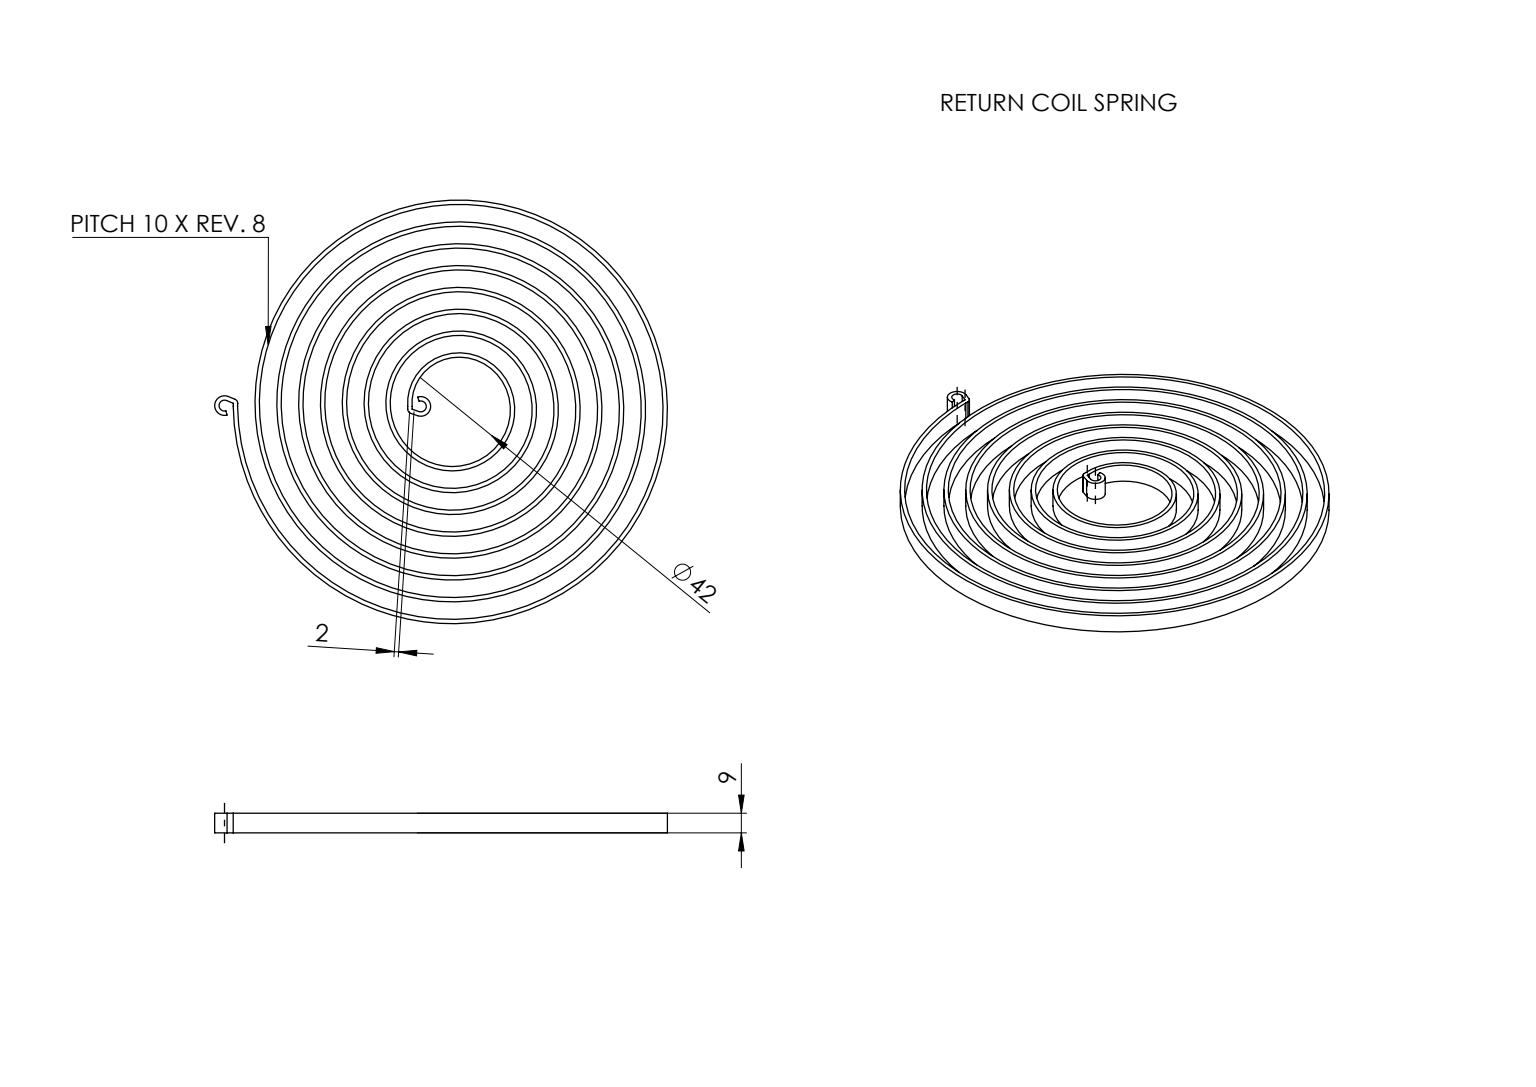
ISO-10303-21;
HEADER;
FILE_DESCRIPTION (('STEP AP214'),
    '1' );
FILE_NAME ('Return Coil Spring.step',
    '2026-10-08T11:45:07',
    ( '' ),
    ( '' ),
    'SwSTEP 2.0',
    'SolidWorks 2026',
    '' );
FILE_SCHEMA (( 'AUTOMOTIVE_DESIGN' ));
ENDSEC;

DATA;
#8=CARTESIAN_POINT ( 'NONE',  ( -38.31599561464027914, 40.00000000000000000, 10.26995502114586678 ) ) ;
#9=CARTESIAN_POINT ( 'NONE',  ( -48.87578956996785706, 40.00000000000000000, 16.50293044077288940 ) ) ;
#19=CARTESIAN_POINT ( 'NONE',  ( -15.99999999999997691, 17.11489954122026447, -2.499999999999994671 ) ) ;
#36=CARTESIAN_POINT ( 'NONE',  ( -50.06114249714176623, 31.00000000000000355, -38.53249520213265811 ) ) ;
#44=CARTESIAN_POINT ( 'NONE',  ( 25.34170449640226508, 40.00000000000000000, 74.97748276543396173 ) ) ;
#56=CARTESIAN_POINT ( 'NONE',  ( 73.00591898829820536, 31.00000000000000000, 19.54754034098114701 ) ) ;
#81=DIRECTION ( 'NONE',  ( 0.000000000000000000, 1.000000000000000000, -1.060184893785364939E-15 ) ) ;
#85=CARTESIAN_POINT ( 'NONE',  ( 15.66220904948440662, 31.00000000000000355, -31.63873590539992264 ) ) ;
#94=CARTESIAN_POINT ( 'NONE',  ( 55.55275676651330485, 40.00000000000000000, 14.97830846782891712 ) ) ;
#109=CARTESIAN_POINT ( 'NONE',  ( 33.03432996520027132, 31.00000000000000355, -28.98482729919588863 ) ) ;
#116=CARTESIAN_POINT ( 'NONE',  ( -78.67873774631718220, 31.00000000000000711, 60.36924185307643143 ) ) ;
#119=CARTESIAN_POINT ( 'NONE',  ( -67.85934734803990409, 31.00000000000000711, 22.92939687791763248 ) ) ;
#120=CARTESIAN_POINT ( 'NONE',  ( 33.43413415811954792, 40.00000000000000000, -67.56680175473154293 ) ) ;
#139=CARTESIAN_POINT ( 'NONE',  ( -5.399612364985466151, 40.00000000000000000, -82.39583333413678190 ) ) ;
#157=ADVANCED_FACE ( 'NONE', ( #19485 ), #6553, .F. ) ;
#159=( LENGTH_UNIT ( ) NAMED_UNIT ( * ) SI_UNIT ( .MILLI., .METRE. ) );
#168=CARTESIAN_POINT ( 'NONE',  ( -23.19911330973958030, 31.00000000000000355, -68.30030121463531145 ) ) ;
#171=CARTESIAN_POINT ( 'NONE',  ( 32.80084743084299248, 31.00000000000000355, 19.01436317119123842 ) ) ;
#172=CARTESIAN_POINT ( 'NONE',  ( -21.28946418274055929, 40.00000000000000000, -79.45670318283352174 ) ) ;
#183=CARTESIAN_POINT ( 'NONE',  ( 50.09382087749727930, 40.00000000000000000, 24.69014870349942825 ) ) ;
#197=CARTESIAN_POINT ( 'NONE',  ( 96.56285295106283684, 31.00000000000000000, 12.84127866191736977 ) ) ;
#213=CARTESIAN_POINT ( 'NONE',  ( -25.29482881991252086, 31.00000000000000355, -32.96004927633274662 ) ) ;
#219=CARTESIAN_POINT ( 'NONE',  ( 32.11716166826300167, 40.00000000000000000, 15.82712457579038912 ) ) ;
#221=CARTESIAN_POINT ( 'NONE',  ( 42.86166521172830102, 40.00000000000000000, 21.22462828019262204 ) ) ;
#230=CARTESIAN_POINT ( 'NONE',  ( 7.028922914820973311, 40.00000000000000000, 26.21578750688660264 ) ) ;
#237=VECTOR ( 'NONE', #15107, 1000.000000000000000 ) ;
#249=CARTESIAN_POINT ( 'NONE',  ( -20.51812799676685373, 31.00000000000000355, -60.74091093256831897 ) ) ;
#257=CARTESIAN_POINT ( 'NONE',  ( -10.54315780146311532, 40.00000000000000000, 79.17709703063971460 ) ) ;
#270=CARTESIAN_POINT ( 'NONE',  ( -45.94448050778635917, 31.00000000000000355, -79.54744219826071117 ) ) ;
#292=ORIENTED_EDGE ( 'NONE', *, *, #9832, .T. ) ;
#302=CARTESIAN_POINT ( 'NONE',  ( -29.39530816626169241, 31.00000000000000355, -14.54745122861254814 ) ) ;
#314=CARTESIAN_POINT ( 'NONE',  ( -17.30549157494238344, 40.00000000000000000, -51.24895740946764988 ) ) ;
#324=CARTESIAN_POINT ( 'NONE',  ( -105.9879088449591933, 17.11489954122026447, -4.880719929157669945 ) ) ;
#325=CARTESIAN_POINT ( 'NONE',  ( 3.108867721649529958, 31.00000000000000355, 47.39583333474234905 ) ) ;
#333=CARTESIAN_POINT ( 'NONE',  ( -20.64238946400878305, 31.00000000000000355, 3.177240882809045708 ) ) ;
#335=CARTESIAN_POINT ( 'NONE',  ( 58.84426737335365232, 31.00000000000000355, 76.69096868241209108 ) ) ;
#340=CARTESIAN_POINT ( 'NONE',  ( -25.88810397299713628, 31.00000000000000355, 75.89534075019484760 ) ) ;
#341=CARTESIAN_POINT ( 'NONE',  ( -79.00001692107187523, 40.00000000000000711, 21.04436337234429999 ) ) ;
#346=ORIENTED_EDGE ( 'NONE', *, *, #31412, .T. ) ;
#357=CARTESIAN_POINT ( 'NONE',  ( 36.87680687886029318, 40.00000000000000000, -74.81172728975037955 ) ) ;
#386=CARTESIAN_POINT ( 'NONE',  ( -20.07939870814534089, 31.00000000000000355, -2.638545259751242877 ) ) ;
#390=ADVANCED_FACE ( 'NONE', ( #24276 ), #4353, .F. ) ;
#393=CARTESIAN_POINT ( 'NONE',  ( -9.469526743414824921, 31.00000000000000355, -71.82433816204535049 ) ) ;
#396=CARTESIAN_POINT ( 'NONE',  ( 31.88898475263450649, 31.00000000000000355, 36.48290236124523744 ) ) ;
#397=CARTESIAN_POINT ( 'NONE',  ( 63.16980243745005907, 39.99999999999999289, -55.41789732285823078 ) ) ;
#413=CARTESIAN_POINT ( 'NONE',  ( 51.69409438402072965, 40.00000000000000000, -17.56033928829605273 ) ) ;
#426=CARTESIAN_POINT ( 'NONE',  ( -73.90312034494817794, 31.00000000000000711, -56.84521418461152109 ) ) ;
#440=CARTESIAN_POINT ( 'NONE',  ( -101.9145453900124068, 31.00000000000000355, -1.407535261550473704 ) ) ;
#448=AXIS2_PLACEMENT_3D ( 'NONE', #41556, #21331, #31328 ) ;
#450=CARTESIAN_POINT ( 'NONE',  ( -39.89583333501392559, 31.00000000000000355, 2.617993869485681468 ) ) ;
#457=CARTESIAN_POINT ( 'NONE',  ( -16.75480014238754478, 40.00000000000000000, -49.32177912249007790 ) ) ;
#458=CARTESIAN_POINT ( 'NONE',  ( -37.13421060599359436, 40.00000000000000000, -21.52932707635456211 ) ) ;
#466=CARTESIAN_POINT ( 'NONE',  ( -12.50349052776452297, 40.00000000000000000, 25.37591446456323041 ) ) ;
#468=DIRECTION ( 'NONE',  ( 0.000000000000000000, 1.000000000000000000, 0.000000000000000000 ) ) ;
#484=CARTESIAN_POINT ( 'NONE',  ( -59.63693792270941429, 31.00000000000000711, 15.87187584493272929 ) ) ;
#488=FACE_OUTER_BOUND ( 'NONE', #34162, .T. ) ;
#491=CARTESIAN_POINT ( 'NONE',  ( -82.09281090897877675, 40.00000000000000711, -5.486092462564050365 ) ) ;
#511=CARTESIAN_POINT ( 'NONE',  ( -60.37409795221152109, 31.00000000000000711, -68.82020352599361956 ) ) ;
#517=EDGE_CURVE ( 'NONE', #5078, #15357, #24037, .T. ) ;
#541=CARTESIAN_POINT ( 'NONE',  ( 2.319640971205256363, 31.00000000000000355, -34.59922639972668179 ) ) ;
#548=CARTESIAN_POINT ( 'NONE',  ( -6.590854309045714565, 40.00000000000000000, 49.37518673228670707 ) ) ;
#558=CARTESIAN_POINT ( 'NONE',  ( 40.56819808336118882, 31.00000000000000355, -35.59309480518532354 ) ) ;
#567=CARTESIAN_POINT ( 'NONE',  ( 5.935205493550105516, 40.00000000000000000, -22.18504493031268865 ) ) ;
#573=CARTESIAN_POINT ( 'NONE',  ( 61.98103557012429121, 31.00000000000000000, 47.69015029125303329 ) ) ;
#574=CARTESIAN_POINT ( 'NONE',  ( 73.52353481979008620, 39.99999999999999289, 25.08131146963209090 ) ) ;
#586=CARTESIAN_POINT ( 'NONE',  ( 84.89583333414414312, 39.99999999999999289, -5.563236982362012029 ) ) ;
#589=ORIENTED_EDGE ( 'NONE', *, *, #18866, .T. ) ;
#591=CARTESIAN_POINT ( 'NONE',  ( -105.9879088449591933, 31.00000000000000355, -0.3807199291576673361 ) ) ;
#600=DIRECTION ( 'NONE',  ( 0.000000000000000000, 1.000000000000000000, -1.060184893785364939E-15 ) ) ;
#608=CARTESIAN_POINT ( 'NONE',  ( -10.31048697494744815, 31.00000000000000355, -30.34325702988586215 ) ) ;
#614=CARTESIAN_POINT ( 'NONE',  ( -68.16583574478268304, 31.00000000000000711, -18.25112749842637427 ) ) ;
#617=CARTESIAN_POINT ( 'NONE',  ( -13.02511903071888355, 31.00000000000000355, 48.29538318457647961 ) ) ;
#618=CARTESIAN_POINT ( 'NONE',  ( -79.89583333417640176, 40.00000000000000711, 5.235987747608064957 ) ) ;
#627=CARTESIAN_POINT ( 'NONE',  ( 35.44578089419255917, 40.00000000000000000, -40.42088417236866604 ) ) ;
#644=VECTOR ( 'NONE', #35434, 1000.000000000000000 ) ;
#659=CARTESIAN_POINT ( 'NONE',  ( -19.20510714644778361, 31.00000000000000355, 33.27066566623395261 ) ) ;
#666=CARTESIAN_POINT ( 'NONE',  ( -29.60425243605831724, 40.00000000000000000, 38.59963703562669934 ) ) ;
#667=CARTESIAN_POINT ( 'NONE',  ( 40.10317558969867946, 40.00000000000000000, -23.06553963618951286 ) ) ;
#677=CARTESIAN_POINT ( 'NONE',  ( 15.62097837807030842, 40.00000000000000000, -17.81927981957692353 ) ) ;
#695=CARTESIAN_POINT ( 'NONE',  ( 4.437437895627577511, 31.00000000000000355, 69.40004907510417809 ) ) ;
#702=CARTESIAN_POINT ( 'NONE',  ( -6.060882879309179572, 40.00000000000000000, -94.40013096063921694 ) ) ;
#707=DIRECTION ( 'NONE',  ( 0.000000000000000000, 0.000000000000000000, -1.000000000000000000 ) ) ;
#716=CARTESIAN_POINT ( 'NONE',  ( -72.39171112334068425, 31.00000000000000711, -55.52881859171880308 ) ) ;
#733=DIRECTION ( 'NONE',  ( -0.9470131699890044219, 0.000000000000000000, 0.3211947320043981868 ) ) ;
#745=VECTOR ( 'NONE', #33359, 1000.000000000000000 ) ;
#749=CARTESIAN_POINT ( 'NONE',  ( -8.786317949316114095, 31.00000000000000355, -33.00646673688142840 ) ) ;
#757=CARTESIAN_POINT ( 'NONE',  ( 15.22596115864829969, 40.00000000000000000, 57.21640888977480444 ) ) ;
#771=CARTESIAN_POINT ( 'NONE',  ( 52.68777711438346500, 31.00000000000000355, 17.88338314711659294 ) ) ;
#776=CARTESIAN_POINT ( 'NONE',  ( -16.73417733071809721, 40.00000000000000000, -12.82953315787133519 ) ) ;
#781=CARTESIAN_POINT ( 'NONE',  ( 68.60033760563639760, 31.00000000000000000, -33.70054013428169526 ) ) ;
#782=CARTESIAN_POINT ( 'NONE',  ( 57.21690105882998267, 39.99999999999999289, -50.04162206025958426 ) ) ;
#796=CARTESIAN_POINT ( 'NONE',  ( 21.49215960483416410, 40.00000000000000000, -80.26604385357094884 ) ) ;
#820=CARTESIAN_POINT ( 'NONE',  ( -24.68525358734468611, 31.00000000000000355, -18.92943107747915832 ) ) ;
#827=CARTESIAN_POINT ( 'NONE',  ( -61.47519263390311295, 31.00000000000000711, -35.49250405583519807 ) ) ;
#832=CARTESIAN_POINT ( 'NONE',  ( 22.78600399167716262, 31.00000000000000355, -39.30137845375363526 ) ) ;
#834=CARTESIAN_POINT ( 'NONE',  ( -68.69954721042445556, 40.00000000000000711, 39.68009708086182741 ) ) ;
#845=CARTESIAN_POINT ( 'NONE',  ( -47.94314659152439617, 40.00000000000000000, -16.27230485535717719 ) ) ;
#858=CARTESIAN_POINT ( 'NONE',  ( -96.33078216555148288, 31.00000000000000711, 32.58251675337926656 ) ) ;
#859=ADVANCED_FACE ( 'NONE', ( #7595 ), #30942, .T. ) ;
#873=CARTESIAN_POINT ( 'NONE',  ( 21.71086051706764763, 31.00000000000000355, -37.60982366119799991 ) ) ;
#882=CARTESIAN_POINT ( 'NONE',  ( 6.197074855318628117, 40.00000000000000000, 46.98549035852928313 ) ) ;
#883=CARTESIAN_POINT ( 'NONE',  ( 56.43498182459031653, 40.00000000000000000, -7.339809665447900144 ) ) ;
#893=CARTESIAN_POINT ( 'NONE',  ( 24.60508655230852781, 40.00000000000000000, 6.583411914924224284 ) ) ;
#907=CARTESIAN_POINT ( 'NONE',  ( 58.79931003850258975, 31.00000000000000355, 51.72161244499935151 ) ) ;
#908=ADVANCED_FACE ( 'NONE', ( #10220 ), #3863, .T. ) ;
#916=CARTESIAN_POINT ( 'NONE',  ( 63.29164158768324455, 39.99999999999999289, -71.97807289018581400 ) ) ;
#927=CARTESIAN_POINT ( 'NONE',  ( -39.09256291070916944, 31.00000000000000355, 79.30589209199378331 ) ) ;
#934=CARTESIAN_POINT ( 'NONE',  ( -15.43003214871520434, 40.00000000000000000, -17.59684744742188300 ) ) ;
#954=CARTESIAN_POINT ( 'NONE',  ( 25.04716826810500763, 31.00000000000000355, 3.293035637142270655 ) ) ;
#962=CARTESIAN_POINT ( 'NONE',  ( -19.32876798325804302, 31.00000000000000355, -39.37500834189552279 ) ) ;
#969=CARTESIAN_POINT ( 'NONE',  ( 60.82800096160986669, 39.99999999999999289, 30.10617641797072963 ) ) ;
#981=CARTESIAN_POINT ( 'NONE',  ( 54.89583333452979730, 31.00000000000000355, -3.599741573803383332 ) ) ;
#991=CARTESIAN_POINT ( 'NONE',  ( -4.233603722440171246, 40.00000000000000000, -32.08218167604271542 ) ) ;
#995=CARTESIAN_POINT ( 'NONE',  ( 72.60479858918232310, 31.00000000000000000, -24.53750584076950503 ) ) ;
#996=CARTESIAN_POINT ( 'NONE',  ( 60.45897909546184934, 39.99999999999999289, -46.24578392211154210 ) ) ;
#999=AXIS2_PLACEMENT_3D ( 'NONE', #30530, #600, #23567 ) ;
#1009=FACE_OUTER_BOUND ( 'NONE', #21764, .T. ) ;
#1012=CARTESIAN_POINT ( 'NONE',  ( 76.36724925129128394, 39.99999999999999289, 58.57876755120444301 ) ) ;
#1013=LINE ( 'NONE', #20939, #23659 ) ;
#1023=CARTESIAN_POINT ( 'NONE',  ( -18.66214908251097881, 40.00000000000000000, 24.25811346063289164 ) ) ;
#1036=CARTESIAN_POINT ( 'NONE',  ( 23.12883206328222130, 31.00000000000000355, 11.39561251172168355 ) ) ;
#1047=CARTESIAN_POINT ( 'NONE',  ( 40.54457361686378647, 31.00000000000000355, 52.83773991529862712 ) ) ;
#1049=CARTESIAN_POINT ( 'NONE',  ( 38.14553738579559905, 31.00000000000000355, 29.36968266378863746 ) ) ;
#1050=CARTESIAN_POINT ( 'NONE',  ( -76.41092972884307244, 40.00000000000000711, -25.93877460596726436 ) ) ;
#1064=CARTESIAN_POINT ( 'NONE',  ( 47.00375723443311671, 40.00000000000000000, -27.15133022689256137 ) ) ;
#1096=CARTESIAN_POINT ( 'NONE',  ( 28.66079171547214699, 31.00000000000000355, 21.97938003711830035 ) ) ;
#1108=CARTESIAN_POINT ( 'NONE',  ( 12.21457428495364006, 40.00000000000000000, 45.57612047952555656 ) ) ;
#1109=CARTESIAN_POINT ( 'NONE',  ( -47.35250803175856049, 40.00000000000000000, -23.44639516808875257 ) ) ;
#1118=CARTESIAN_POINT ( 'NONE',  ( 25.10416666396844576, 40.00000000000000000, 1.636246165087044124 ) ) ;
#1136=CARTESIAN_POINT ( 'NONE',  ( 50.06853320191206791, 31.00000000000000000, -56.91684085115753078 ) ) ;
#1145=ORIENTED_EDGE ( 'NONE', *, *, #9536, .T. ) ;
#1146=CARTESIAN_POINT ( 'NONE',  ( 58.37089435906660384, 39.99999999999999289, -75.89027429297954086 ) ) ;
#1155=CARTESIAN_POINT ( 'NONE',  ( 81.15556025174309696, 31.00000000000000000, 27.54985289775053658 ) ) ;
#1160=CARTESIAN_POINT ( 'NONE',  ( -13.43146050690766735, 40.00000000000000000, 27.15249184974963015 ) ) ;
#1164=AXIS2_PLACEMENT_3D ( 'NONE', #31098, #1183, #33928 ) ;
#1183=DIRECTION ( 'NONE',  ( 0.000000000000000000, -1.000000000000000000, 5.297542245118643184E-16 ) ) ;
#1188=CARTESIAN_POINT ( 'NONE',  ( 14.57966847436265212, 31.00000000000000355, -42.69519604896471776 ) ) ;
#1197=CARTESIAN_POINT ( 'NONE',  ( -20.51812799677388455, 40.00000000000000000, -60.74091093256832607 ) ) ;
#1212=CARTESIAN_POINT ( 'NONE',  ( 17.07784400123870938, 31.00000000000000355, -50.31546185293520779 ) ) ;
#1219=CARTESIAN_POINT ( 'NONE',  ( 29.64712525329720449, 40.00000000000000000, -17.12831674356021239 ) ) ;
#1225=CARTESIAN_POINT ( 'NONE',  ( 64.75392801420538547, 31.00000000000000000, -56.64582372546510669 ) ) ;
#1226=CARTESIAN_POINT ( 'NONE',  ( 42.86165537668587433, 40.00000000000000000, -73.99543480067944756 ) ) ;
#1231=VECTOR ( 'NONE', #41233, 1000.000000000000000 ) ;
#1242=CARTESIAN_POINT ( 'NONE',  ( 63.67823170517923614, 39.99999999999999289, 72.58713758494482704 ) ) ;
#1257=CARTESIAN_POINT ( 'NONE',  ( -29.39530816626169596, 40.00000000000000000, -14.54745122861429252 ) ) ;
#1271=CARTESIAN_POINT ( 'NONE',  ( -4.233603722440171246, 31.00000000000000355, -32.08218167604271542 ) ) ;
#1272=ORIENTED_EDGE ( 'NONE', *, *, #26632, .F. ) ;
#1277=CARTESIAN_POINT ( 'NONE',  ( -75.41724699911947027, 31.00000000000000711, 25.61573074746135248 ) ) ;
#1280=CARTESIAN_POINT ( 'NONE',  ( 41.62382930724211860, 31.00000000000000355, -20.43270582883756248 ) ) ;
#1281=CARTESIAN_POINT ( 'NONE',  ( -58.57471716409879292, 40.00000000000000711, 66.78942258476980953 ) ) ;
#1289=CARTESIAN_POINT ( 'NONE',  ( -22.00000000000000000, 31.00000000000000355, -7.355690625810191807E-15 ) ) ;
#1291=AXIS2_PLACEMENT_3D ( 'NONE', #13178, #29752, #29970 ) ;
#1293=CARTESIAN_POINT ( 'NONE',  ( -16.10381281257427943, 40.00000000000000000, -60.09637020943575436 ) ) ;
#1325=CARTESIAN_POINT ( 'NONE',  ( 32.65420139560029611, 31.00000000000000355, -42.57517516360295673 ) ) ;
#1332=CARTESIAN_POINT ( 'NONE',  ( -38.92335646797288717, 40.00000000000000000, 29.86975225897632313 ) ) ;
#1333=CARTESIAN_POINT ( 'NONE',  ( -26.81486728383016072, 40.00000000000000000, -46.61672233255473685 ) ) ;
#1339=CARTESIAN_POINT ( 'NONE',  ( -38.31599561464027914, 40.00000000000000000, 10.26995502114586678 ) ) ;
#1355=CARTESIAN_POINT ( 'NONE',  ( -22.66037885604483648, 31.00000000000000355, 66.40833514169634100 ) ) ;
#1361=EDGE_CURVE ( 'NONE', #7867, #25259, #40258, .T. ) ;
#1364=CARTESIAN_POINT ( 'NONE',  ( -29.11455967534193334, 40.00000000000000000, 85.38284731560057139 ) ) ;
#1365=CARTESIAN_POINT ( 'NONE',  ( -1.587008504153756938, 31.00000000000000355, -24.39691638390477380 ) ) ;
#1381=CARTESIAN_POINT ( 'NONE',  ( 26.62151981922250243, 40.00000000000000000, -3.482817046706076169 ) ) ;
#1383=VERTEX_POINT ( 'NONE', #10602 ) ;
#1402=CARTESIAN_POINT ( 'NONE',  ( -15.99999999999997691, 17.11489954122026447, 5.571627607371296764E-15 ) ) ;
#1405=CARTESIAN_POINT ( 'NONE',  ( -40.27082278477694643, 31.00000000000000355, 10.71261860272906397 ) ) ;
#1414=CARTESIAN_POINT ( 'NONE',  ( 66.37122006405570573, 39.99999999999999289, -8.639838683448301637 ) ) ;
#1417=FACE_OUTER_BOUND ( 'NONE', #14128, .T. ) ;
#1425=CARTESIAN_POINT ( 'NONE',  ( -27.38011802910879311, 31.00000000000000355, -55.51905197969063011 ) ) ;
#1426=DIRECTION ( 'NONE',  ( 0.9247238835424298475, 0.000000000000000000, 0.3806385939525924744 ) ) ;
#1435=CARTESIAN_POINT ( 'NONE',  ( 83.01093309086799366, 31.00000000000000000, 28.30804032755801458 ) ) ;
#1436=CARTESIAN_POINT ( 'NONE',  ( -59.98614492175870794, 40.00000000000000711, 68.21249229748744369 ) ) ;
#1449=CARTESIAN_POINT ( 'NONE',  ( -99.89583333318432778, 40.00000000000000711, 6.544984695199788760 ) ) ;
#1463=CARTESIAN_POINT ( 'NONE',  ( -15.23573235977941032, 40.00000000000000000, 26.30445775087293114 ) ) ;
#1473=PLANE ( 'NONE',  #40141 ) ;
#1478=CARTESIAN_POINT ( 'NONE',  ( -1.799870782497340782, 31.00000000000000355, 27.60416666422008802 ) ) ;
#1484=CARTESIAN_POINT ( 'NONE',  ( -77.84600223180727596, 31.00000000000000711, -20.84395318355897686 ) ) ;
#1488=CARTESIAN_POINT ( 'NONE',  ( 43.74200748489511881, 31.00000000000000355, 38.49442098324159645 ) ) ;
#1491=CARTESIAN_POINT ( 'NONE',  ( 6.054110834496887250, 40.00000000000000000, -92.60416666599778068 ) ) ;
#1504=CARTESIAN_POINT ( 'NONE',  ( -8.856203846296160975, 40.00000000000000000, 67.27320953167645712 ) ) ;
#1517=CARTESIAN_POINT ( 'NONE',  ( 6.386360208629405122, 31.00000000000000355, 99.40013590833048340 ) ) ;
#1533=CARTESIAN_POINT ( 'NONE',  ( 23.39270017067629936, 31.00000000000000355, 40.49502024156475244 ) ) ;
#1544=CARTESIAN_POINT ( 'NONE',  ( -46.87443272357899815, 40.00000000000000000, 35.96965017775951878 ) ) ;
#1545=CARTESIAN_POINT ( 'NONE',  ( -59.63693792272297856, 40.00000000000000711, 15.87187584492933823 ) ) ;
#1552=CARTESIAN_POINT ( 'NONE',  ( 7.411374251232441424, 31.00000000000000355, -21.84767871671174788 ) ) ;
#1555=CARTESIAN_POINT ( 'NONE',  ( 20.45440555730427690, 40.00000000000000000, -26.67302265141799467 ) ) ;
#1563=FACE_OUTER_BOUND ( 'NONE', #19348, .T. ) ;
#1570=CARTESIAN_POINT ( 'NONE',  ( -31.21560191380782001, 31.00000000000000355, 63.07420938637471863 ) ) ;
#1578=CARTESIAN_POINT ( 'NONE',  ( 72.29027477046881245, 39.99999999999999289, -63.25088587038124643 ) ) ;
#1579=CARTESIAN_POINT ( 'NONE',  ( -101.1468392228030098, 40.00000000000000711, 13.20405500234329921 ) ) ;
#1594=CARTESIAN_POINT ( 'NONE',  ( -3.169834189307653816, 40.00000000000000000, -24.13593742708953727 ) ) ;
#1620=CARTESIAN_POINT ( 'NONE',  ( 41.62382930724211860, 31.00000000000000355, -20.43270582883756248 ) ) ;
#1621=ORIENTED_EDGE ( 'NONE', *, *, #34799, .T. ) ;
#1629=CARTESIAN_POINT ( 'NONE',  ( -38.62815422673675414, 40.00000000000000000, -50.51519254952906124 ) ) ;
#1636=( NAMED_UNIT ( * ) PLANE_ANGLE_UNIT ( ) SI_UNIT ( $, .RADIAN. ) );
#1640=CARTESIAN_POINT ( 'NONE',  ( 33.41571365387085280, 31.00000000000000355, 57.85165222247763239 ) ) ;
#1651=CARTESIAN_POINT ( 'NONE',  ( 69.92891852055319646, 31.00000000000000000, 53.79372986807582180 ) ) ;
#1652=CARTESIAN_POINT ( 'NONE',  ( 83.01093309090690298, 39.99999999999999289, 28.30804032753857058 ) ) ;
#1667=CARTESIAN_POINT ( 'NONE',  ( -12.08748825390017068, 40.00000000000000000, -91.69541640458645304 ) ) ;
#1682=CARTESIAN_POINT ( 'NONE',  ( -23.27229071022945561, 40.00000000000000000, 20.35677778009942074 ) ) ;
#1694=CARTESIAN_POINT ( 'NONE',  ( -5.542584477697039880, 31.00000000000000355, -42.01772079774592328 ) ) ;
#1700=CARTESIAN_POINT ( 'NONE',  ( -5.072363130230006512, 31.00000000000000355, 77.60416666578095146 ) ) ;
#1702=CARTESIAN_POINT ( 'NONE',  ( -38.36856355434107257, 31.00000000000000355, 33.53830235993100217 ) ) ;
#1704=CARTESIAN_POINT ( 'NONE',  ( 38.45889818826288575, 40.00000000000000000, 77.98987599019784511 ) ) ;
#1719=CARTESIAN_POINT ( 'NONE',  ( -59.82155519081633344, 40.00000000000000711, -7.874468279900277423 ) ) ;
#1724=CLOSED_SHELL ( 'NONE', ( #33748, #24407, #157, #36662, #5189, #23558, #390, #13764, #40052, #859, #36455, #9652, #29855, #18232, #42688, #39745, #11732, #908, #27872, #4463, #1907, #5772, #22328, #14283, #29088, #39216, #37250, #35865 ) ) ;
#1738=VERTEX_POINT ( 'NONE', #36723 ) ;
#1750=CARTESIAN_POINT ( 'NONE',  ( -50.10416666532988472, 31.00000000000000355, -3.272492339034341224 ) ) ;
#1757=CARTESIAN_POINT ( 'NONE',  ( -51.34291522965900612, 40.00000000000000000, 29.65708359768123970 ) ) ;
#1759=CARTESIAN_POINT ( 'NONE',  ( 32.82854187708761629, 40.00000000000000000, -56.64543409044760125 ) ) ;
#1769=CARTESIAN_POINT ( 'NONE',  ( 23.79574588541966662, 31.00000000000000355, -6.380716493563439506 ) ) ;
#1772=CARTESIAN_POINT ( 'NONE',  ( 10.63353083439206870, 40.00000000000000000, -31.33693976183458219 ) ) ;
#1785=CARTESIAN_POINT ( 'NONE',  ( -74.30604906370724905, 31.00000000000000711, -36.76128443491435860 ) ) ;
#1796=CARTESIAN_POINT ( 'NONE',  ( -6.638544827991895048, 40.00000000000000000, 99.59190654106264162 ) ) ;
#1797=CARTESIAN_POINT ( 'NONE',  ( -14.30682334061562067, 31.00000000000000355, -18.65445469299708492 ) ) ;
#1809=CARTESIAN_POINT ( 'NONE',  ( -94.39576909109665337, 31.00000000000000711, 32.06004391471374504 ) ) ;
#1812=CARTESIAN_POINT ( 'NONE',  ( -18.66214908251097881, 40.00000000000000000, 24.25811346063289164 ) ) ;
#1835=ORIENTED_EDGE ( 'NONE', *, *, #5889, .T. ) ;
#1838=CIRCLE ( 'NONE', #22774, 4.500000000000000888 ) ;
#1840=CYLINDRICAL_SURFACE ( 'NONE', #32683, 2.500000000000000444 ) ;
#1842=CARTESIAN_POINT ( 'NONE',  ( -5.264430561742837078, 31.00000000000000355, 39.44269128747090747 ) ) ;
#1846=EDGE_CURVE ( 'NONE', #7063, #33557, #17971, .T. ) ;
#1851=CARTESIAN_POINT ( 'NONE',  ( -53.44803860755722269, 40.00000000000000000, 46.73995993581220176 ) ) ;
#1863=CARTESIAN_POINT ( 'NONE',  ( 49.83821931962687302, 31.00000000000000355, 43.70611527624207326 ) ) ;
#1872=CARTESIAN_POINT ( 'NONE',  ( 66.32976035609178211, 31.00000000000000000, 58.33333674018341952 ) ) ;
#1873=CARTESIAN_POINT ( 'NONE',  ( 78.79907178679739843, 39.99999999999999289, 38.97904116291323362 ) ) ;
#1900=CARTESIAN_POINT ( 'NONE',  ( 33.88265278290065652, 40.00000000000000000, 16.77599488388066007 ) ) ;
#1907=ADVANCED_FACE ( 'NONE', ( #4413 ), #18019, .F. ) ;
#1908=EDGE_LOOP ( 'NONE', ( #29076, #35836, #6519, #20696 ) ) ;
#1912=CARTESIAN_POINT ( 'NONE',  ( -20.88694679984194380, 31.00000000000000355, -36.15586224631631751 ) ) ;
#1918=CARTESIAN_POINT ( 'NONE',  ( 10.12401712103624263, 31.00000000000000355, 76.79210772277129138 ) ) ;
#1923=CARTESIAN_POINT ( 'NONE',  ( -48.87578956997907653, 31.00000000000000355, 16.50293044076727611 ) ) ;
#1924=CARTESIAN_POINT ( 'NONE',  ( -44.26264085331523290, 40.00000000000000711, 76.66224561666088277 ) ) ;
#1936=CARTESIAN_POINT ( 'NONE',  ( -51.86900026051868196, 40.00000000000000000, 45.50549606403863123 ) ) ;
#1950=EDGE_LOOP ( 'NONE', ( #13636, #31594, #9140, #29773 ) ) ;
#1958=CARTESIAN_POINT ( 'NONE',  ( -15.99999999999997691, 31.00000000000000355, -2.499999999999994671 ) ) ;
#1968=CARTESIAN_POINT ( 'NONE',  ( 26.72236725836960147, 31.00000000000000355, -46.28813965123160301 ) ) ;
#1975=CARTESIAN_POINT ( 'NONE',  ( 18.36587843422771016, 40.00000000000000000, 54.06640964556338957 ) ) ;
#1981=CARTESIAN_POINT ( 'NONE',  ( 17.96659372829068246, 31.00000000000000355, -15.76829228678407624 ) ) ;
#1983=CARTESIAN_POINT ( 'NONE',  ( -4.929261580875707871, 40.00000000000000000, 37.46659216873931797 ) ) ;
#1995=CARTESIAN_POINT ( 'NONE',  ( -5.410573124821301150, 31.00000000000000355, -84.40011308935179102 ) ) ;
#1998=AXIS2_PLACEMENT_3D ( 'NONE', #12015, #32851, #21645 ) ;
#2005=CARTESIAN_POINT ( 'NONE',  ( -80.34276469473088866, 40.00000000000000711, 61.48650092628135866 ) ) ;
#2006=CARTESIAN_POINT ( 'NONE',  ( 26.10672890669568602, 31.00000000000000355, 8.893381768403882504 ) ) ;
#2018=CARTESIAN_POINT ( 'NONE',  ( 4.274771203358150196, 40.00000000000000000, -32.49882260841580006 ) ) ;
#2019=CARTESIAN_POINT ( 'NONE',  ( -30.82418422902937039, 40.00000000000000000, 26.94311707097686792 ) ) ;
#2037=DIRECTION ( 'NONE',  ( 0.000000000000000000, 1.541976423090494253E-15, 1.000000000000000000 ) ) ;
#2046=ORIENTED_EDGE ( 'NONE', *, *, #35248, .T. ) ;
#2047=CARTESIAN_POINT ( 'NONE',  ( 46.08863070263671347, 31.00000000000000355, 35.47900410130831972 ) ) ;
#2053=CARTESIAN_POINT ( 'NONE',  ( -19.10382689932985656, 40.00000000000000000, -71.73905014343321795 ) ) ;
#2060=FACE_OUTER_BOUND ( 'NONE', #15986, .T. ) ;
#2065=CARTESIAN_POINT ( 'NONE',  ( 16.30650823456882748, 31.00000000000000355, -60.90571087954511142 ) ) ;
#2073=CARTESIAN_POINT ( 'NONE',  ( -37.02054590706428172, 31.00000000000000355, -75.34311506435014394 ) ) ;
#2074=CARTESIAN_POINT ( 'NONE',  ( -40.08783408682389648, 40.00000000000000000, 81.04563091341927361 ) ) ;
#2095=CARTESIAN_POINT ( 'NONE',  ( 27.02985023942251175, 31.00000000000000355, 3.586895573513789071 ) ) ;
#2096=DIRECTION ( 'NONE',  ( 0.000000000000000000, 0.000000000000000000, 1.000000000000000000 ) ) ;
#2102=CARTESIAN_POINT ( 'NONE',  ( -2.659806967433698599, 40.00000000000000000, 39.59793253468611596 ) ) ;
#2118=CARTESIAN_POINT ( 'NONE',  ( 34.98270738856093232, 31.00000000000000355, 4.602016392115340970 ) ) ;
#2124=CARTESIAN_POINT ( 'NONE',  ( -45.94448050778635917, 31.00000000000000355, -79.54744219826071117 ) ) ;
#2126=CARTESIAN_POINT ( 'NONE',  ( 25.95756378415329024, 31.00000000000000355, 52.86556711865710412 ) ) ;
#2128=CARTESIAN_POINT ( 'NONE',  ( -84.90650804512098659, 40.00000000000000711, 28.83788733109305014 ) ) ;
#2141=CARTESIAN_POINT ( 'NONE',  ( 55.68207322487837274, 39.99999999999999289, -32.16283696846894458 ) ) ;
#2154=ORIENTED_EDGE ( 'NONE', *, *, #19399, .F. ) ;
#2169=CARTESIAN_POINT ( 'NONE',  ( 43.96541952717798551, 31.00000000000000355, 11.76906328551413239 ) ) ;
#2175=CARTESIAN_POINT ( 'NONE',  ( 28.01378275134445772, 40.00000000000000000, -56.83506808085938644 ) ) ;
#2184=CARTESIAN_POINT ( 'NONE',  ( 11.92156526682413720, 40.00000000000000000, 35.08788755311113761 ) ) ;
#2198=CARTESIAN_POINT ( 'NONE',  ( 77.59064570035201314, 31.00000000000000000, -38.12735739514867817 ) ) ;
#2208=CARTESIAN_POINT ( 'NONE',  ( 14.33709021557830887, 31.00000000000000355, 24.89380824183666263 ) ) ;
#2221=CARTESIAN_POINT ( 'NONE',  ( -26.76192867387533170, 40.00000000000000000, -15.44647709060871321 ) ) ;
#2223=CARTESIAN_POINT ( 'NONE',  ( 37.09854380388319584, 40.00000000000000000, 2.490183985263671129 ) ) ;
#2247=CARTESIAN_POINT ( 'NONE',  ( -45.80426865612386678, 31.00000000000000355, -26.55377233851146812 ) ) ;
#2253=CARTESIAN_POINT ( 'NONE',  ( 4.437437895627098783, 40.00000000000000000, 69.40004907513484511 ) ) ;
#2267=CARTESIAN_POINT ( 'NONE',  ( -47.15756294055117337, 31.00000000000000355, -53.75246728999482571 ) ) ;
#2272=EDGE_CURVE ( 'NONE', #5078, #31476, #13578, .T. ) ;
#2276=CARTESIAN_POINT ( 'NONE',  ( 43.66223835209735427, 31.00000000000000355, 88.82794485014694885 ) ) ;
#2277=CARTESIAN_POINT ( 'NONE',  ( 96.90013369365227902, 39.99999999999999289, -6.223598210838602540 ) ) ;
#2295=CARTESIAN_POINT ( 'NONE',  ( -21.37212791037561388, 31.00000000000000355, -7.253704819187424491 ) ) ;
#2302=CARTESIAN_POINT ( 'NONE',  ( -37.13421060599359436, 40.00000000000000000, -21.52932707635456211 ) ) ;
#2317=CARTESIAN_POINT ( 'NONE',  ( 2.454369252093185239, 31.00000000000000355, 37.39583333513270702 ) ) ;
#2319=( NAMED_UNIT ( * ) PLANE_ANGLE_UNIT ( ) SI_UNIT ( $, .RADIAN. ) );
#2323=CARTESIAN_POINT ( 'NONE',  ( -77.37786320076959612, 31.00000000000000711, 44.69160382239309115 ) ) ;
#2327=CARTESIAN_POINT ( 'NONE',  ( 8.570044366903687205, 31.00000000000000355, -64.27561742005508449 ) ) ;
#2341=CARTESIAN_POINT ( 'NONE',  ( 74.89583333416871369, 39.99999999999999289, -4.908738512848213276 ) ) ;
#2347=AXIS2_PLACEMENT_3D ( 'NONE', #14230, #10722, #10960 ) ;
#2367=DIRECTION ( 'NONE',  ( 0.000000000000000000, -1.000000000000000000, 5.297542245118643184E-16 ) ) ;
#2373=CARTESIAN_POINT ( 'NONE',  ( 3.763366191185776088, 31.00000000000000355, 57.39583333449059666 ) ) ;
#2378=CARTESIAN_POINT ( 'NONE',  ( -59.82155519081633344, 40.00000000000000711, -7.874468279900277423 ) ) ;
#2388=CARTESIAN_POINT ( 'NONE',  ( 11.12085686420672381, 40.00000000000000000, -41.54537790535560760 ) ) ;
#2400=CARTESIAN_POINT ( 'NONE',  ( 76.16439905407254685, 31.00000000000000000, 44.11546174421767574 ) ) ;
#2409=CARTESIAN_POINT ( 'NONE',  ( 43.66223835209735427, 40.00000000000000000, 88.82794485019093145 ) ) ;
#2421=CARTESIAN_POINT ( 'NONE',  ( 33.47591237148697729, 31.00000000000000355, -8.973542178613062248 ) ) ;
#2429=CARTESIAN_POINT ( 'NONE',  ( 24.63052733448982323, 40.00000000000000000, -3.251868155982907904 ) ) ;
#2430=CARTESIAN_POINT ( 'NONE',  ( 36.95980244579788376, 40.00000000000000000, 4.931273285801174744 ) ) ;
#2441=CARTESIAN_POINT ( 'NONE',  ( -105.3367680159044966, 40.00000000000000000, 2.032994142711228136 ) ) ;
#2451=CARTESIAN_POINT ( 'NONE',  ( -90.10416666596678681, 40.00000000000000711, -5.890486217120279200 ) ) ;
#2460=CARTESIAN_POINT ( 'NONE',  ( -17.30549157494827384, 31.00000000000000355, -51.24895740946764988 ) ) ;
#2469=CARTESIAN_POINT ( 'NONE',  ( 67.48878131082858545, 39.99999999999999289, 39.09986611101696496 ) ) ;
#2480=CARTESIAN_POINT ( 'NONE',  ( 57.76613438074698337, 31.00000000000000000, -28.48799604501563110 ) ) ;
#2493=CARTESIAN_POINT ( 'NONE',  ( 92.49871336439160530, 31.00000000000000000, 31.53380891771210415 ) ) ;
#2494=CARTESIAN_POINT ( 'NONE',  ( 59.96221986557397088, 40.00000000000000000, 78.35452998770438171 ) ) ;
#2499=CARTESIAN_POINT ( 'NONE',  ( -105.9879088449591933, 31.00000000000000355, -2.880719929157669945 ) ) ;
#2511=CARTESIAN_POINT ( 'NONE',  ( 12.72035051019680729, 31.00000000000000355, 25.87482915247129611 ) ) ;
#2524=CARTESIAN_POINT ( 'NONE',  ( 14.57966847436756019, 40.00000000000000000, -42.69519604897453036 ) ) ;
#2539=CARTESIAN_POINT ( 'NONE',  ( 24.02862666965263116, 31.00000000000000355, 27.38392887651082575 ) ) ;
#2545=CARTESIAN_POINT ( 'NONE',  ( 52.74436945453300041, 31.00000000000000355, 68.73989242669851762 ) ) ;
#2549=CARTESIAN_POINT ( 'NONE',  ( -38.62815422673675414, 31.00000000000000355, -50.51519254952904703 ) ) ;
#2550=CARTESIAN_POINT ( 'NONE',  ( -46.76215110880508519, 40.00000000000000000, 53.15211786533807725 ) ) ;
#2568=CARTESIAN_POINT ( 'NONE',  ( 5.072363130230502115, 40.00000000000000000, 77.39583333421907696 ) ) ;
#2594=CARTESIAN_POINT ( 'NONE',  ( -104.2750351721725650, 39.99999999999999289, -4.541977405098627685 ) ) ;
#2597=CARTESIAN_POINT ( 'NONE',  ( 8.201713468707295007, 31.00000000000000355, -62.30543997111072940 ) ) ;
#2600=CARTESIAN_POINT ( 'NONE',  ( -27.06829236441750552, 31.00000000000000355, 15.58100167312263018 ) ) ;
#2601=CARTESIAN_POINT ( 'NONE',  ( -68.16583574478268304, 40.00000000000000711, -18.25112749842637427 ) ) ;
#2612=CARTESIAN_POINT ( 'NONE',  ( -12.41726970680908515, 40.00000000000000000, 46.38546114896210071 ) ) ;
#2626=CARTESIAN_POINT ( 'NONE',  ( 56.68048384767583769, 31.00000000000000000, -64.44707192207098956 ) ) ;
#2632=DIRECTION ( 'NONE',  ( -0.9979848074931935153, 0.000000000000000000, -0.06345332152672163162 ) ) ;
#2633=CARTESIAN_POINT ( 'NONE',  ( 12.87762912549411354, 40.00000000000000000, 98.66289914827740404 ) ) ;
#2640=AXIS2_PLACEMENT_3D ( 'NONE', #29871, #16124, #40056 ) ;
#2643=CARTESIAN_POINT ( 'NONE',  ( -9.022452542771789652, 31.00000000000000355, 26.59230923919664491 ) ) ;
#2649=CARTESIAN_POINT ( 'NONE',  ( -2.454369252093152376, 40.00000000000000000, 37.60416666486730009 ) ) ;
#2650=CARTESIAN_POINT ( 'NONE',  ( 31.41502175087570947, 40.00000000000000000, -18.07270130326806523 ) ) ;
#2660=CARTESIAN_POINT ( 'NONE',  ( -19.99999999999999645, 40.00000000000000000, 0.000000000000000000 ) ) ;
#2676=CARTESIAN_POINT ( 'NONE',  ( -42.11670055801651102, 31.00000000000000355, -32.42481051985740237 ) ) ;
#2683=CARTESIAN_POINT ( 'NONE',  ( 9.885896071376818028, 40.00000000000000000, -74.20985814143865866 ) ) ;
#2694=CARTESIAN_POINT ( 'NONE',  ( -64.44063486737354651, 31.00000000000000711, -49.42892067282641477 ) ) ;
#2704=CARTESIAN_POINT ( 'NONE',  ( -46.83686391397709770, 31.00000000000000355, -81.34213072392142863 ) ) ;
#2705=CARTESIAN_POINT ( 'NONE',  ( -91.59543978412355614, 40.00000000000000711, -12.18496625897608254 ) ) ;
#2707=EDGE_CURVE ( 'NONE', #1738, #25968, #37641, .T. ) ;
#2733=CARTESIAN_POINT ( 'NONE',  ( 34.59698569361206211, 40.00000000000000000, -30.23997570423562209 ) ) ;
#2744=CARTESIAN_POINT ( 'NONE',  ( -45.59965607524345899, 31.00000000000000355, -22.47439267160796916 ) ) ;
#2749=CARTESIAN_POINT ( 'NONE',  ( 5.726861599741335240, 31.00000000000000355, 87.39583333411552246 ) ) ;
#2756=CARTESIAN_POINT ( 'NONE',  ( 22.12550800842194931, 31.00000000000000355, 65.48657384636695156 ) ) ;
#2757=CARTESIAN_POINT ( 'NONE',  ( -61.81085491475939619, 40.00000000000000711, 35.57109242552864004 ) ) ;
#2758=CARTESIAN_POINT ( 'NONE',  ( 91.55691129138550366, 39.99999999999999289, -24.53049628908797430 ) ) ;
#2768=CARTESIAN_POINT ( 'NONE',  ( -43.59452257625678584, 40.00000000000000000, -56.81327804312699925 ) ) ;
#2799=CARTESIAN_POINT ( 'NONE',  ( -54.58798567973315841, 31.00000000000000355, -26.90590473539369754 ) ) ;
#2803=CARTESIAN_POINT ( 'NONE',  ( -29.88476798293162418, 31.00000000000000355, 10.10044382456042911 ) ) ;
#2804=CARTESIAN_POINT ( 'NONE',  ( 48.66231590555653241, 39.99999999999999289, -55.48862040801123641 ) ) ;
#2815=CARTESIAN_POINT ( 'NONE',  ( 43.15607885788778475, 40.00000000000000000, -11.56636786368396486 ) ) ;
#2828=CARTESIAN_POINT ( 'NONE',  ( -23.42519174998115616, 31.00000000000000355, 87.00664592748896098 ) ) ;
#2837=VECTOR ( 'NONE', #8399, 1000.000000000000000 ) ;
#2846=DIRECTION ( 'NONE',  ( 1.000000000000000000, 0.000000000000000000, 0.000000000000000000 ) ) ;
#2849=CARTESIAN_POINT ( 'NONE',  ( 7.028922914820973311, 31.00000000000000355, 26.21578750688660264 ) ) ;
#2856=CARTESIAN_POINT ( 'NONE',  ( 2.781618486875130358, 40.00000000000000000, -42.60416666509636485 ) ) ;
#2857=CARTESIAN_POINT ( 'NONE',  ( -17.88900094062007184, 40.00000000000000000, 36.12696699726038219 ) ) ;
#2882=CARTESIAN_POINT ( 'NONE',  ( 67.09393615762301977, 31.00000000000000000, 4.495243625008654043 ) ) ;
#2888=CARTESIAN_POINT ( 'NONE',  ( -70.49178429274644486, 40.00000000000000711, 40.57739572807859929 ) ) ;
#2903=CARTESIAN_POINT ( 'NONE',  ( -5.072363130230006512, 31.00000000000000355, 77.60416666578095146 ) ) ;
#2915=CARTESIAN_POINT ( 'NONE',  ( -79.17211737996690601, 31.00000000000000711, 45.58486055166099504 ) ) ;
#2916=CARTESIAN_POINT ( 'NONE',  ( 6.309545988805658645, 40.00000000000000000, -94.59213238963913284 ) ) ;
#2933=CARTESIAN_POINT ( 'NONE',  ( -20.42974159057666483, 31.00000000000000355, -10.07157319949386753 ) ) ;
#2941=CARTESIAN_POINT ( 'NONE',  ( -41.03896728212566103, 40.00000000000000000, -11.06873348903577892 ) ) ;
#2951=CARTESIAN_POINT ( 'NONE',  ( -6.851565232941113415, 31.00000000000000355, -51.95325991929587417 ) ) ;
#2957=CARTESIAN_POINT ( 'NONE',  ( 84.66040299356156140, 31.00000000000000000, 11.14692016787551765 ) ) ;
#2961=CARTESIAN_POINT ( 'NONE',  ( -9.228224334391116557, 31.00000000000000355, 69.24269282083176336 ) ) ;
#2962=CARTESIAN_POINT ( 'NONE',  ( 30.38134496340388324, 40.00000000000000000, 61.85720693096894252 ) ) ;
#2975=EDGE_CURVE ( 'NONE', #7939, #15282, #32818, .T. ) ;
#2976=CARTESIAN_POINT ( 'NONE',  ( -10.16518460146908787, 40.00000000000000000, 77.20874865269769316 ) ) ;
#2984=VECTOR ( 'NONE', #19550, 1000.000000000000000 ) ;
#3007=CARTESIAN_POINT ( 'NONE',  ( 42.30435120181500963, 31.00000000000000355, 37.09784777058769123 ) ) ;
#3010=CARTESIAN_POINT ( 'NONE',  ( 36.89914868738900822, 31.00000000000000355, -2.354335741662294534 ) ) ;
#3011=CARTESIAN_POINT ( 'NONE',  ( -35.92146702467432817, 40.00000000000000000, -62.19081021767443218 ) ) ;
#3019=CARTESIAN_POINT ( 'NONE',  ( -32.63632984357925437, 40.00000000000000000, -25.02932899672474676 ) ) ;
#3032=ORIENTED_EDGE ( 'NONE', *, *, #15639, .F. ) ;
#3035=CARTESIAN_POINT ( 'NONE',  ( 22.98560153734151257, 31.00000000000000355, 86.26083236265422727 ) ) ;
#3053=CARTESIAN_POINT ( 'NONE',  ( -10.31048697494744815, 31.00000000000000355, -30.34325702988586215 ) ) ;
#3061=CARTESIAN_POINT ( 'NONE',  ( -23.50435451693408950, 40.00000000000000000, 30.64856077952424940 ) ) ;
#3062=CARTESIAN_POINT ( 'NONE',  ( 20.11321884379431779, 40.00000000000000000, -40.61652209560084259 ) ) ;
#3094=CARTESIAN_POINT ( 'NONE',  ( -58.36801134197498442, 31.00000000000000711, 19.71467013092928866 ) ) ;
#3102=CARTESIAN_POINT ( 'NONE',  ( 83.01093309090690298, 39.99999999999999289, 28.30804032753857058 ) ) ;
#3116=CARTESIAN_POINT ( 'NONE',  ( -68.69954721042445556, 31.00000000000000711, 39.68009708086182741 ) ) ;
#3125=CARTESIAN_POINT ( 'NONE',  ( 94.26586287999620595, 31.00000000000000000, 25.37251369639959364 ) ) ;
#3150=CARTESIAN_POINT ( 'NONE',  ( -13.43146050690766380, 31.00000000000000355, 27.15249184975281693 ) ) ;
#3157=CARTESIAN_POINT ( 'NONE',  ( 24.31498657911848227, 40.00000000000000000, 42.27453502171530175 ) ) ;
#3168=CARTESIAN_POINT ( 'NONE',  ( -105.9879088449591933, 39.99999999999999289, -4.880719929157669945 ) ) ;
#3171=CARTESIAN_POINT ( 'NONE',  ( 42.20483333784007840, 31.00000000000000355, -14.33818270462009359 ) ) ;
#3179=CARTESIAN_POINT ( 'NONE',  ( -86.05617919112455638, 31.00000000000000711, 49.70311056393224192 ) ) ;
#3181=VERTEX_POINT ( 'NONE', #27161 ) ;
#3182=CARTESIAN_POINT ( 'NONE',  ( -62.09442273006147417, 31.00000000000000711, -4.163950221635984938 ) ) ;
#3183=CARTESIAN_POINT ( 'NONE',  ( -31.21560191380782712, 40.00000000000000000, 63.07420938637471863 ) ) ;
#3184=CARTESIAN_POINT ( 'NONE',  ( -99.89583333318432778, 40.00000000000000711, 6.544984695199788760 ) ) ;
#3199=CARTESIAN_POINT ( 'NONE',  ( 24.81019160154284720, 40.00000000000000000, 73.04493173762017477 ) ) ;
#3214=CARTESIAN_POINT ( 'NONE',  ( -15.43003214871520434, 40.00000000000000000, -17.59684744742188300 ) ) ;
#3233=CARTESIAN_POINT ( 'NONE',  ( 4.090615425948669781, 31.00000000000000355, -62.60416666561555132 ) ) ;
#3238=CARTESIAN_POINT ( 'NONE',  ( 23.59836588145513048, 31.00000000000000355, -26.81698947917456266 ) ) ;
#3239=CARTESIAN_POINT ( 'NONE',  ( -30.22953878324074495, 40.00000000000000000, 61.32923288305941867 ) ) ;
#3249=CARTESIAN_POINT ( 'NONE',  ( -29.60425243605831724, 40.00000000000000000, 38.59963703562669934 ) ) ;
#3263=CARTESIAN_POINT ( 'NONE',  ( -105.9879088449591933, 40.00000000000000000, -2.880719929157669945 ) ) ;
#3266=CARTESIAN_POINT ( 'NONE',  ( -46.83686391397709770, 31.00000000000000355, -81.34213072392142863 ) ) ;
#3281=CARTESIAN_POINT ( 'NONE',  ( -29.59829689555773058, 31.00000000000000355, 3.906358533625565954 ) ) ;
#3289=CARTESIAN_POINT ( 'NONE',  ( 33.47591237148697729, 40.00000000000000000, -8.973542178613062248 ) ) ;
#3291=CARTESIAN_POINT ( 'NONE',  ( -52.09564885855072447, 40.00000000000000000, -3.498939618562995513 ) ) ;
#3321=CARTESIAN_POINT ( 'NONE',  ( -61.79211991636739754, 31.00000000000000711, -8.240724169199884486 ) ) ;
#3324=DIRECTION ( 'NONE',  ( 0.2604563316218754254, 5.114700905345146860E-16, 0.9654856287475623855 ) ) ;
#3333=CARTESIAN_POINT ( 'NONE',  ( 11.20008397363331198, 40.00000000000000000, -84.14439686172906363 ) ) ;
#3345=CARTESIAN_POINT ( 'NONE',  ( -26.42126989340051324, 31.00000000000000355, -77.78956226056263290 ) ) ;
#3353=CARTESIAN_POINT ( 'NONE',  ( -22.00000000000000711, 40.00000000000000000, 0.000000000000000000 ) ) ;
#3358=CARTESIAN_POINT ( 'NONE',  ( -91.07534658258107640, 31.00000000000000711, 44.76935032132903558 ) ) ;
#3375=CARTESIAN_POINT ( 'NONE',  ( -1.974796425974089331, 31.00000000000000355, 29.60085432090884439 ) ) ;
#3378=FACE_OUTER_BOUND ( 'NONE', #6020, .T. ) ;
#3383=CARTESIAN_POINT ( 'NONE',  ( 12.64472494877221997, 40.00000000000000000, 47.53373494968590762 ) ) ;
#3395=CARTESIAN_POINT ( 'NONE',  ( -48.80550277073417931, 31.00000000000000355, -13.06547612810710035 ) ) ;
#3404=CARTESIAN_POINT ( 'NONE',  ( 48.45023387855729879, 31.00000000000000355, 83.88660019351674180 ) ) ;
#3407=CARTESIAN_POINT ( 'NONE',  ( 67.48878131082855703, 31.00000000000000000, 39.09986611101695786 ) ) ;
#3408=CARTESIAN_POINT ( 'NONE',  ( -35.65230965300054322, 40.00000000000000000, 72.05959145982365044 ) ) ;
#3425=CARTESIAN_POINT ( 'NONE',  ( -44.26264085331523290, 40.00000000000000711, 76.66224561666088277 ) ) ;
#3455=CARTESIAN_POINT ( 'NONE',  ( 64.78932475141161262, 31.00000000000000000, 8.528958657501300777 ) ) ;
#3457=CARTESIAN_POINT ( 'NONE',  ( -30.58448433907586761, 31.00000000000000355, 8.146263651248247584 ) ) ;
#3458=CARTESIAN_POINT ( 'NONE',  ( 75.10416666583130052, 39.99999999999999289, 4.908738512847474311 ) ) ;
#3467=CARTESIAN_POINT ( 'NONE',  ( -18.68892229297488683, 40.00000000000000000, 55.06009237583231197 ) ) ;
#3481=CARTESIAN_POINT ( 'NONE',  ( 84.84057271803867195, 31.00000000000000000, 49.13019966417499518 ) ) ;
#3497=CARTESIAN_POINT ( 'NONE',  ( 33.70925502316616473, 31.00000000000000355, 11.43906998022225707 ) ) ;
#3498=CIRCLE ( 'NONE', #33483, 2.500000000000002665 ) ;
#3506=CARTESIAN_POINT ( 'NONE',  ( 9.621748599878955588, 40.00000000000000000, 35.89595399306684698 ) ) ;
#3507=CARTESIAN_POINT ( 'NONE',  ( 22.78600399168703916, 40.00000000000000000, -39.30137845373389638 ) ) ;
#3525=AXIS2_PLACEMENT_3D ( 'NONE', #15837, #12560, #28719 ) ;
#3533=CARTESIAN_POINT ( 'NONE',  ( 16.92944795086299337, 31.00000000000000355, -62.81076020704204410 ) ) ;
#3541=CARTESIAN_POINT ( 'NONE',  ( -49.21613380539481142, 40.00000000000000000, 63.96793098899348706 ) ) ;
#3552=CARTESIAN_POINT ( 'NONE',  ( -71.24862878704732339, 31.00000000000000711, 35.13526414049667324 ) ) ;
#3581=CARTESIAN_POINT ( 'NONE',  ( 36.95980244579787666, 31.00000000000000355, 4.931273285801173856 ) ) ;
#3591=CARTESIAN_POINT ( 'NONE',  ( 56.43498182459031653, 40.00000000000000000, -7.339809665447900144 ) ) ;
#3599=ORIENTED_EDGE ( 'NONE', *, *, #18866, .F. ) ;
#3604=CARTESIAN_POINT ( 'NONE',  ( 20.73284993368543638, 31.00000000000000355, 42.03655757353646294 ) ) ;
#3610=EDGE_CURVE ( 'NONE', #39678, #29860, #33844, .T. ) ;
#3611=CARTESIAN_POINT ( 'NONE',  ( -99.99999999999997158, 31.00000000000000711, 2.428179185498535730E-12 ) ) ;
#3615=CARTESIAN_POINT ( 'NONE',  ( -9.616483412539254871, 31.00000000000000355, -73.82325415884287168 ) ) ;
#3616=CARTESIAN_POINT ( 'NONE',  ( -32.59403919554602425, 40.00000000000000000, -66.35267222978370683 ) ) ;
#3630=CARTESIAN_POINT ( 'NONE',  ( -84.90650804512098659, 40.00000000000000711, 28.83788733109305014 ) ) ;
#3645=CARTESIAN_POINT ( 'NONE',  ( -22.00000000000000711, 40.00000000000000000, 0.000000000000000000 ) ) ;
#3661=CARTESIAN_POINT ( 'NONE',  ( -70.10416666575086708, 31.00000000000000711, -4.581489278090966621 ) ) ;
#3663=CARTESIAN_POINT ( 'NONE',  ( -40.32452739092001792, 31.00000000000000355, -13.76986825753265897 ) ) ;
#3664=CARTESIAN_POINT ( 'NONE',  ( -75.41724699911947027, 40.00000000000000711, 25.61573074746135248 ) ) ;
#3672=CARTESIAN_POINT ( 'NONE',  ( 6.892732713553924917, 40.00000000000000000, -52.36990085009771434 ) ) ;
#3687=CARTESIAN_POINT ( 'NONE',  ( -91.21105805184879500, 31.00000000000000711, 11.89862498597365104 ) ) ;
#3696=EDGE_CURVE ( 'NONE', #42330, #5107, #17780, .T. ) ;
#3705=CARTESIAN_POINT ( 'NONE',  ( 4.888094100070568437, 31.00000000000000355, 37.04995123692341252 ) ) ;
#3711=CARTESIAN_POINT ( 'NONE',  ( 35.44578089419255917, 40.00000000000000000, -40.42088417236866604 ) ) ;
#3712=CARTESIAN_POINT ( 'NONE',  ( -22.33566874673302038, 40.00000000000000000, 45.10700316350094141 ) ) ;
#3719=CARTESIAN_POINT ( 'NONE',  ( -5.732510072307491988, 40.00000000000000000, -21.37570426403446078 ) ) ;
#3721=CARTESIAN_POINT ( 'NONE',  ( -15.99999999999997691, 40.00000000000000000, -2.499999999999994671 ) ) ;
#3732=CARTESIAN_POINT ( 'NONE',  ( -105.9879088449591933, 17.11489954122026447, 2.119280070842335384 ) ) ;
#3737=CARTESIAN_POINT ( 'NONE',  ( -37.00582609755892349, 31.00000000000000355, 48.07482304779467341 ) ) ;
#3747=CARTESIAN_POINT ( 'NONE',  ( 39.32569335900156915, 40.00000000000000000, 68.32161714264680086 ) ) ;
#3760=CARTESIAN_POINT ( 'NONE',  ( -89.21153162435624040, 31.00000000000000711, 11.76024306507019901 ) ) ;
#3769=CARTESIAN_POINT ( 'NONE',  ( -87.85203729257557370, 31.00000000000000711, 50.59313708110082786 ) ) ;
#3790=CARTESIAN_POINT ( 'NONE',  ( -31.59164309906361368, 31.00000000000000355, 4.115917706319392799 ) ) ;
#3801=CARTESIAN_POINT ( 'NONE',  ( 56.82522199879618086, 40.00000000000000000, 7.581518937762242949 ) ) ;
#3803=PRODUCT_DEFINITION_CONTEXT ( 'detailed design', #33984, 'design' ) ;
#3812=CARTESIAN_POINT ( 'NONE',  ( 54.85378563033546584, 31.00000000000000355, 7.219977902337870290 ) ) ;
#3819=CARTESIAN_POINT ( 'NONE',  ( 21.81281596512078025, 40.00000000000000000, -10.76194779073239083 ) ) ;
#3820=EDGE_CURVE ( 'NONE', #6869, #29181, #27764, .T. ) ;
#3823=CARTESIAN_POINT ( 'NONE',  ( -105.9879088449591933, 31.00000000000000711, 4.119280070842334496 ) ) ;
#3826=CARTESIAN_POINT ( 'NONE',  ( -58.00742674159663892, 31.00000000000000711, -44.63796826975934096 ) ) ;
#3828=CARTESIAN_POINT ( 'NONE',  ( 25.34170449640226508, 40.00000000000000000, 74.97748276543396173 ) ) ;
#3841=CARTESIAN_POINT ( 'NONE',  ( -58.57471716409879292, 40.00000000000000711, 66.78942258476980953 ) ) ;
#3852=CARTESIAN_POINT ( 'NONE',  ( 0.000000000000000000, 0.000000000000000000, 0.000000000000000000 ) ) ;
#3856=CARTESIAN_POINT ( 'NONE',  ( 18.71272080434063056, 40.00000000000000000, 21.38210947162712117 ) ) ;
#3863=PLANE ( 'NONE',  #999 ) ;
#3865=CARTESIAN_POINT ( 'NONE',  ( -104.8158553526607477, 31.00000000000000711, 3.963965400206363565 ) ) ;
#3866=ORIENTED_EDGE ( 'NONE', *, *, #33914, .F. ) ;
#3871=CARTESIAN_POINT ( 'NONE',  ( -28.96462450050677973, 31.00000000000000355, -9.827991688575851370 ) ) ;
#3877=CARTESIAN_POINT ( 'NONE',  ( -45.35818215263140019, 31.00000000000000355, 51.72168634911185592 ) ) ;
#3882=CARTESIAN_POINT ( 'NONE',  ( -37.12595630542501368, 31.00000000000000355, 18.22532657727797556 ) ) ;
#3886=CARTESIAN_POINT ( 'NONE',  ( 34.02738612458995959, 40.00000000000000000, 69.00154638599002510 ) ) ;
#3896=CARTESIAN_POINT ( 'NONE',  ( -3.436116956419240864, 40.00000000000000000, -52.39583333462812931 ) ) ;
#3910=CARTESIAN_POINT ( 'NONE',  ( 25.57473013255608052, 31.00000000000000355, 95.94174708837350352 ) ) ;
#3930=CARTESIAN_POINT ( 'NONE',  ( -33.98628324864968420, 31.00000000000000355, 19.63407011443918293 ) ) ;
#3939=CARTESIAN_POINT ( 'NONE',  ( 47.00375723443311671, 40.00000000000000000, -27.15133022689256137 ) ) ;
#3940=CARTESIAN_POINT ( 'NONE',  ( -3.331996295684063636, 40.00000000000000000, 49.59602437329134972 ) ) ;
#3951=CARTESIAN_POINT ( 'NONE',  ( -9.654069774896838041, 40.00000000000000000, -19.56573356436190636 ) ) ;
#3971=CARTESIAN_POINT ( 'NONE',  ( -36.82253293460209420, 31.00000000000000355, -63.98115709646774718 ) ) ;
#3978=CARTESIAN_POINT ( 'NONE',  ( -23.42519174997118014, 40.00000000000000000, 87.00664592748896098 ) ) ;
#3992=CARTESIAN_POINT ( 'NONE',  ( 68.41617299536980568, 31.00000000000000000, 52.47886963225217016 ) ) ;
#4000=CYLINDRICAL_SURFACE ( 'NONE', #13688, 2.500000000000002665 ) ;
#4022=CARTESIAN_POINT ( 'NONE',  ( -20.28213647682921206, 31.00000000000000355, 23.06128528321892546 ) ) ;
#4030=CARTESIAN_POINT ( 'NONE',  ( -7.015336270754768400, 40.00000000000000000, -53.95087245962636047 ) ) ;
#4039=CARTESIAN_POINT ( 'NONE',  ( -38.74991464700507748, 31.00000000000000355, 44.18781823130588293 ) ) ;
#4048=CARTESIAN_POINT ( 'NONE',  ( -31.57754862722326905, 31.00000000000000355, 93.01713655900283584 ) ) ;
#4053=CARTESIAN_POINT ( 'NONE',  ( -4.761419979751499554, 31.00000000000000355, -74.40007767863900767 ) ) ;
#4054=CARTESIAN_POINT ( 'NONE',  ( 67.48878131082858545, 39.99999999999999289, 39.09986611101696496 ) ) ;
#4070=CARTESIAN_POINT ( 'NONE',  ( 63.16980243745005907, 39.99999999999999289, -55.41789732285823078 ) ) ;
#4084=CARTESIAN_POINT ( 'NONE',  ( -20.42974159057667194, 40.00000000000000000, -10.07157319949504526 ) ) ;
#4095=CARTESIAN_POINT ( 'NONE',  ( 7.411374251232441424, 31.00000000000000355, -21.84767871671174788 ) ) ;
#4102=CARTESIAN_POINT ( 'NONE',  ( 57.13603463884887645, 31.00000000000000355, 32.98675068510902264 ) ) ;
#4106=CARTESIAN_POINT ( 'NONE',  ( -11.35616125661755937, 31.00000000000000355, -42.69191301634815261 ) ) ;
#4107=CARTESIAN_POINT ( 'NONE',  ( -10.16518460146908787, 40.00000000000000000, 77.20874865269769316 ) ) ;
#4120=CARTESIAN_POINT ( 'NONE',  ( 23.58227068755204314, 40.00000000000000000, -47.84673847638903510 ) ) ;
#4151=CARTESIAN_POINT ( 'NONE',  ( 34.89583333524210218, 31.00000000000000355, -2.290744634698907767 ) ) ;
#4157=CARTESIAN_POINT ( 'NONE',  ( 13.71368254939966036, 40.00000000000000000, -51.22554439249349656 ) ) ;
#4158=CARTESIAN_POINT ( 'NONE',  ( -19.43072497041043079, 40.00000000000000000, 56.92208038676060511 ) ) ;
#4170=CARTESIAN_POINT ( 'NONE',  ( -1.472621547668719444, 40.00000000000000000, -22.39583333634585571 ) ) ;
#4185=CARTESIAN_POINT ( 'NONE',  ( 66.15140951848846385, 31.00000000000000000, -38.07406969931856366 ) ) ;
#4195=EDGE_CURVE ( 'NONE', #9994, #39678, #22024, .T. ) ;
#4197=CARTESIAN_POINT ( 'NONE',  ( -89.42636861580037078, 40.00000000000000711, -24.07434901465519417 ) ) ;
#4210=CARTESIAN_POINT ( 'NONE',  ( 77.05880969081472642, 31.00000000000000000, 37.98468489477117771 ) ) ;
#4214=CARTESIAN_POINT ( 'NONE',  ( 8.075107282079295956, 40.00000000000000000, -23.73893940452291318 ) ) ;
#4222=AXIS2_PLACEMENT_3D ( 'NONE', #35229, #5355, #18722 ) ;
#4228=CARTESIAN_POINT ( 'NONE',  ( -16.80298683001097260, 31.00000000000000355, 2.367532924972516994 ) ) ;
#4233=EDGE_LOOP ( 'NONE', ( #37828, #38523, #36491, #14282, #3599, #30070, #8392, #9395, #11512, #40219, #19104, #21567, #19961, #35781, #42014, #41297, #19739, #32050, #20009, #17336, #29884, #26607, #26119, #33390, #7628, #26668 ) ) ;
#4242=CARTESIAN_POINT ( 'NONE',  ( -26.91141215548883991, 31.00000000000000355, 30.57553017914614557 ) ) ;
#4251=CARTESIAN_POINT ( 'NONE',  ( 63.11376326756305843, 39.99999999999999289, -21.32174659672108774 ) ) ;
#4263=CARTESIAN_POINT ( 'NONE',  ( 3.763366191185776088, 31.00000000000000355, 57.39583333449059666 ) ) ;
#4268=CARTESIAN_POINT ( 'NONE',  ( -15.87544005811639458, 40.00000000000000000, -27.47754625559162989 ) ) ;
#4273=CARTESIAN_POINT ( 'NONE',  ( -46.76215110878947456, 31.00000000000000355, 53.15211786535368788 ) ) ;
#4274=CARTESIAN_POINT ( 'NONE',  ( 74.15939217265263039, 39.99999999999999289, -19.75058139460558237 ) ) ;
#4286=CARTESIAN_POINT ( 'NONE',  ( 75.74279358916429317, 39.99999999999999289, -37.35102017232331661 ) ) ;
#4299=CARTESIAN_POINT ( 'NONE',  ( 23.40755275317130568, 40.00000000000000000, 30.61714766194360848 ) ) ;
#4311=CARTESIAN_POINT ( 'NONE',  ( 7.028922914820973311, 31.00000000000000355, 26.21578750688660264 ) ) ;
#4318=CARTESIAN_POINT ( 'NONE',  ( 23.52215716829092074, 31.00000000000000355, -69.29398394448777765 ) ) ;
#4321=CARTESIAN_POINT ( 'NONE',  ( 46.89968353241609833, 31.00000000000000355, -2.988513402017745513 ) ) ;
#4323=CARTESIAN_POINT ( 'NONE',  ( 71.66629920589342362, 39.99999999999999289, 24.32769631419027689 ) ) ;
#4336=CARTESIAN_POINT ( 'NONE',  ( -45.59965607524345899, 40.00000000000000000, -22.47439267160796916 ) ) ;
#4353=CYLINDRICAL_SURFACE ( 'NONE', #19923, 2.500000000000002665 ) ;
#4358=CIRCLE ( 'NONE', #35716, 2.500000000000000444 ) ;
#4366=CARTESIAN_POINT ( 'NONE',  ( -9.824444021593908616, 31.00000000000000355, 36.70529466175499778 ) ) ;
#4373=CARTESIAN_POINT ( 'NONE',  ( -36.80126402429788612, 40.00000000000000000, 32.28896105221774349 ) ) ;
#4374=CARTESIAN_POINT ( 'NONE',  ( 44.54779904932823342, 40.00000000000000000, -34.05916983163054113 ) ) ;
#4385=CARTESIAN_POINT ( 'NONE',  ( 19.70274684888802952, 40.00000000000000000, 17.27304525429847359 ) ) ;
#4401=CARTESIAN_POINT ( 'NONE',  ( 9.885896071376816252, 31.00000000000000355, -74.20985814147174153 ) ) ;
#4404=VECTOR ( 'NONE', #35127, 1000.000000000000114 ) ;
#4410=CARTESIAN_POINT ( 'NONE',  ( -68.52217190868857699, 40.00000000000000711, 59.94826526062049510 ) ) ;
#4413=FACE_OUTER_BOUND ( 'NONE', #31086, .T. ) ;
#4422=CARTESIAN_POINT ( 'NONE',  ( 26.74431375183570481, 31.00000000000000355, -78.78324499025107741 ) ) ;
#4425=CARTESIAN_POINT ( 'NONE',  ( 6.473670811831357064, 40.00000000000000000, -24.11571013580714151 ) ) ;
#4432=DIRECTION ( 'NONE',  ( -0.000000000000000000, -1.060184893785364939E-15, -1.000000000000000000 ) ) ;
#4455=CARTESIAN_POINT ( 'NONE',  ( 46.49836147156941024, 31.00000000000000355, -6.043767708844123732 ) ) ;
#4461=CARTESIAN_POINT ( 'NONE',  ( 64.47787635702036368, 39.99999999999999289, -17.16423577040998438 ) ) ;
#4463=ADVANCED_FACE ( 'NONE', ( #8029 ), #1473, .T. ) ;
#4474=CARTESIAN_POINT ( 'NONE',  ( 35.44578089419255917, 31.00000000000000355, -40.42088417236866604 ) ) ;
#4480=CARTESIAN_POINT ( 'NONE',  ( 25.50046184691807483, 40.00000000000000000, -22.37655979312362931 ) ) ;
#4484=CARTESIAN_POINT ( 'NONE',  ( -74.30604906370724905, 31.00000000000000711, -36.76128443491435860 ) ) ;
#4485=CARTESIAN_POINT ( 'NONE',  ( -81.66074000183850501, 40.00000000000000711, -10.87165890510346777 ) ) ;
#4505=CARTESIAN_POINT ( 'NONE',  ( -89.62817255407412631, 40.00000000000000711, -11.80141054548196422 ) ) ;
#4509=DIRECTION ( 'NONE',  ( 0.000000000000000000, -1.000000000000000000, 5.297542245118643184E-16 ) ) ;
#4518=CARTESIAN_POINT ( 'NONE',  ( 32.62694724487211317, 40.00000000000000000, -16.02036196159510339 ) ) ;
#4532=CARTESIAN_POINT ( 'NONE',  ( -20.72449291656876369, 31.00000000000000355, -23.61699481730619610 ) ) ;
#4538=CARTESIAN_POINT ( 'NONE',  ( -79.69263343296167079, 31.00000000000000711, -10.49242979028127820 ) ) ;
#4540=CARTESIAN_POINT ( 'NONE',  ( -26.91141215548883991, 31.00000000000000355, 30.57553017914614557 ) ) ;
#4542=CARTESIAN_POINT ( 'NONE',  ( 81.71702119589899382, 39.99999999999999289, -47.19735719316410183 ) ) ;
#4557=CARTESIAN_POINT ( 'NONE',  ( -40.54929543462775143, 40.00000000000000000, -46.21859917192507794 ) ) ;
#4574=CARTESIAN_POINT ( 'NONE',  ( -98.36195137685432144, 31.00000000000000711, 26.22212808231157055 ) ) ;
#4591=CARTESIAN_POINT ( 'NONE',  ( -40.58740609958903889, 31.00000000000000355, -31.12922691583434798 ) ) ;
#4602=CARTESIAN_POINT ( 'NONE',  ( 43.96541952717798551, 40.00000000000000000, 11.76906328551413239 ) ) ;
#4604=CARTESIAN_POINT ( 'NONE',  ( -30.31917247939794180, 40.00000000000000000, 52.30862930535366928 ) ) ;
#4606=DIRECTION ( 'NONE',  ( 0.000000000000000000, 1.000000000000000000, 0.000000000000000000 ) ) ;
#4609=CARTESIAN_POINT ( 'NONE',  ( -16.73417733071809721, 31.00000000000000355, -12.82953315787133519 ) ) ;
#4612=CARTESIAN_POINT ( 'NONE',  ( -29.26739590608564967, 40.00000000000000000, 25.68069354617348665 ) ) ;
#4629=CARTESIAN_POINT ( 'NONE',  ( 76.69346925293527306, 31.00000000000000000, 10.21457306974767398 ) ) ;
#4638=CARTESIAN_POINT ( 'NONE',  ( 77.87745995356456774, 39.99999999999999289, 59.89653754212418590 ) ) ;
#4640=CARTESIAN_POINT ( 'NONE',  ( -91.07534658258109062, 40.00000000000000711, 44.76935032130646874 ) ) ;
#4652=CARTESIAN_POINT ( 'NONE',  ( -78.67873774631718220, 31.00000000000000711, 60.36924185307643143 ) ) ;
#4658=CARTESIAN_POINT ( 'NONE',  ( -20.42974159057667194, 40.00000000000000000, -10.07157319949504526 ) ) ;
#4683=ORIENTED_EDGE ( 'NONE', *, *, #30969, .T. ) ;
#4686=CARTESIAN_POINT ( 'NONE',  ( -37.12595630542501368, 31.00000000000000355, 18.22532657727797556 ) ) ;
#4694=CARTESIAN_POINT ( 'NONE',  ( -45.90931453312558119, 40.00000000000000000, 40.13788153756827626 ) ) ;
#4708=( LENGTH_UNIT ( ) NAMED_UNIT ( * ) SI_UNIT ( .MILLI., .METRE. ) );
#4712=CARTESIAN_POINT ( 'NONE',  ( -15.01009539198478748, 31.00000000000000355, 56.06562763604418365 ) ) ;
#4713=FACE_OUTER_BOUND ( 'NONE', #10652, .T. ) ;
#4716=CARTESIAN_POINT ( 'NONE',  ( 30.80114556864472775, 40.00000000000000000, -15.19345985420777190 ) ) ;
#4721=CARTESIAN_POINT ( 'NONE',  ( 42.86165537668586722, 31.00000000000000355, -73.99543480067944756 ) ) ;
#4722=CARTESIAN_POINT ( 'NONE',  ( 87.09251733236553150, 39.99999999999999289, 5.815661930448016825 ) ) ;
#4740=CARTESIAN_POINT ( 'NONE',  ( -6.054110834496889026, 40.00000000000000000, -92.39583333400220511 ) ) ;
#4745=DIRECTION ( 'NONE',  ( 0.000000000000000000, 1.000000000000000000, 0.000000000000000000 ) ) ;
#4746=CYLINDRICAL_SURFACE ( 'NONE', #7165, 2.500000000000002665 ) ;
#4753=CARTESIAN_POINT ( 'NONE',  ( 7.507699080470448649, 40.00000000000000000, 28.16210111025598906 ) ) ;
#4772=CARTESIAN_POINT ( 'NONE',  ( -26.76192867387533170, 31.00000000000000355, -15.44647709060871321 ) ) ;
#4779=CARTESIAN_POINT ( 'NONE',  ( 84.24376206367318787, 31.00000000000000000, -11.10575268747775901 ) ) ;
#4781=CARTESIAN_POINT ( 'NONE',  ( 14.32751628686350287, 31.00000000000000355, -53.13354968560084757 ) ) ;
#4782=CARTESIAN_POINT ( 'NONE',  ( 28.03234818517180216, 40.00000000000000000, 82.53419278363811884 ) ) ;
#4795=CARTESIAN_POINT ( 'NONE',  ( 16.30650823456882748, 40.00000000000000000, -60.90571087954511142 ) ) ;
#4799=CARTESIAN_POINT ( 'NONE',  ( -100.0000000000000568, 40.00000000000000000, 2.687954026026062593E-12 ) ) ;
#4816=ORIENTED_EDGE ( 'NONE', *, *, #22573, .T. ) ;
#4824=CARTESIAN_POINT ( 'NONE',  ( 51.69409438402072965, 31.00000000000000355, -17.56033928829605273 ) ) ;
#4832=CARTESIAN_POINT ( 'NONE',  ( 54.43714469963884284, 40.00000000000000000, -7.178810421751046000 ) ) ;
#4833=CARTESIAN_POINT ( 'NONE',  ( 3.791180027291366272, 40.00000000000000000, 59.39995347152935778 ) ) ;
#4837=CARTESIAN_POINT ( 'NONE',  ( -5.732510072307491988, 31.00000000000000355, -21.37570426403446078 ) ) ;
#4839=CARTESIAN_POINT ( 'NONE',  ( -2.127120017302697619, 40.00000000000000000, -32.39583333539214038 ) ) ;
#4854=CARTESIAN_POINT ( 'NONE',  ( -65.32047834223114080, 31.00000000000000711, -32.32491738443057017 ) ) ;
#4862=CARTESIAN_POINT ( 'NONE',  ( 64.90225467577229779, 39.99999999999999289, 74.17428024387139374 ) ) ;
#4863=CARTESIAN_POINT ( 'NONE',  ( 1.622176940739286310, 31.00000000000000355, -24.60292901074088334 ) ) ;
#4877=CARTESIAN_POINT ( 'NONE',  ( 46.76839422403993751, 31.00000000000000000, -81.00140361174831583 ) ) ;
#4879=LINE ( 'NONE', #18240, #16305 ) ;
#4881=CARTESIAN_POINT ( 'NONE',  ( -29.88476798293163128, 40.00000000000000000, 10.10044382456043266 ) ) ;
#4907=CARTESIAN_POINT ( 'NONE',  ( 22.78600399167716262, 31.00000000000000355, -39.30137845375363526 ) ) ;
#4916=CARTESIAN_POINT ( 'NONE',  ( 29.31577600748121881, 40.00000000000000000, 50.95836110724019363 ) ) ;
#4927=CARTESIAN_POINT ( 'NONE',  ( 50.84997085137049311, 31.00000000000000000, -39.01959913718239648 ) ) ;
#4939=CARTESIAN_POINT ( 'NONE',  ( 22.98560153734151257, 31.00000000000000355, 86.26083236265422727 ) ) ;
#4940=CARTESIAN_POINT ( 'NONE',  ( 44.33290732825513203, 40.00000000000000000, 77.00207852759155003 ) ) ;
#4955=CARTESIAN_POINT ( 'NONE',  ( 6.054110834496887250, 40.00000000000000000, -92.60416666599778068 ) ) ;
#4969=CARTESIAN_POINT ( 'NONE',  ( 11.33656872182470643, 40.00000000000000000, -33.21392199183605953 ) ) ;
#4983=CARTESIAN_POINT ( 'NONE',  ( -18.51709390187839688, 31.00000000000000355, -37.54239277154294996 ) ) ;
#4988=CARTESIAN_POINT ( 'NONE',  ( 19.99305134020393382, 31.00000000000000355, 74.61661993947731730 ) ) ;
#4991=CARTESIAN_POINT ( 'NONE',  ( 56.82522199878360425, 31.00000000000000355, 7.581518937762241173 ) ) ;
#4992=CARTESIAN_POINT ( 'NONE',  ( -89.62817255407412631, 40.00000000000000711, -11.80141054548196422 ) ) ;
#5007=CARTESIAN_POINT ( 'NONE',  ( 57.13603463884887645, 40.00000000000000000, 32.98675068510902264 ) ) ;
#5034=CARTESIAN_POINT ( 'NONE',  ( 44.89583333484414140, 31.00000000000000355, -2.945243104263157274 ) ) ;
#5040=CARTESIAN_POINT ( 'NONE',  ( 3.763366191185776088, 40.00000000000000000, 57.39583333449059666 ) ) ;
#5041=CARTESIAN_POINT ( 'NONE',  ( 7.664524495375378166, 40.00000000000000000, 58.91906827748253050 ) ) ;
#5047=CARTESIAN_POINT ( 'NONE',  ( 23.22631124480444598, 31.00000000000000355, -7.893869537065737241 ) ) ;
#5051=CARTESIAN_POINT ( 'NONE',  ( -30.10416666442597844, 40.00000000000000000, -1.963495399902747574 ) ) ;
#5065=CARTESIAN_POINT ( 'NONE',  ( 83.84057477258951963, 31.00000000000000000, -22.33845567675551180 ) ) ;
#5066=VERTEX_POINT ( 'NONE', #14988 ) ;
#5073=CARTESIAN_POINT ( 'NONE',  ( -10.52919346384764054, 31.00000000000000355, -21.36894910329525032 ) ) ;
#5078=VERTEX_POINT ( 'NONE', #28296 ) ;
#5083=CARTESIAN_POINT ( 'NONE',  ( 95.10416666600561086, 31.00000000000000000, 6.217735451873073416 ) ) ;
#5088=CARTESIAN_POINT ( 'NONE',  ( 26.53203760875094019, 40.00000000000000000, 7.134992448515056651 ) ) ;
#5103=DIRECTION ( 'NONE',  ( 0.000000000000000000, 1.000000000000000000, -1.060184893785364939E-15 ) ) ;
#5107=VERTEX_POINT ( 'NONE', #30893 ) ;
#5116=CARTESIAN_POINT ( 'NONE',  ( 12.49611804805956261, 31.00000000000000355, 37.00809541493615029 ) ) ;
#5123=( GEOMETRIC_REPRESENTATION_CONTEXT ( 3 ) GLOBAL_UNCERTAINTY_ASSIGNED_CONTEXT ( ( #26975 ) ) GLOBAL_UNIT_ASSIGNED_CONTEXT ( ( #12825, #2319, #25307 ) ) REPRESENTATION_CONTEXT ( 'NONE', 'WORKASPACE' ) );
#5124=CARTESIAN_POINT ( 'NONE',  ( -59.63693792272297856, 40.00000000000000711, 15.87187584492933823 ) ) ;
#5136=CARTESIAN_POINT ( 'NONE',  ( -23.19911330973958030, 31.00000000000000355, -68.30030121463531145 ) ) ;
#5144=CARTESIAN_POINT ( 'NONE',  ( -10.92011822083620309, 31.00000000000000355, -83.75917815547792600 ) ) ;
#5145=CARTESIAN_POINT ( 'NONE',  ( 5.735608225908777946, 40.00000000000000000, 89.40012361736363289 ) ) ;
#5175=CARTESIAN_POINT ( 'NONE',  ( 35.58384423644164229, 40.00000000000000000, 12.14845634898874494 ) ) ;
#5188=CARTESIAN_POINT ( 'NONE',  ( 30.80114556864472775, 31.00000000000000355, -15.19345985420777190 ) ) ;
#5189=ADVANCED_FACE ( 'NONE', ( #2060 ), #29352, .T. ) ;
#5194=CARTESIAN_POINT ( 'NONE',  ( -70.15350862410126354, 31.00000000000000711, -40.50401079722123399 ) ) ;
#5198=CARTESIAN_POINT ( 'NONE',  ( -23.74678488967455436, 31.00000000000000355, -48.36925102894097961 ) ) ;
#5200=CARTESIAN_POINT ( 'NONE',  ( -70.72766149062127283, 40.00000000000000711, 54.26934393422349956 ) ) ;
#5214=CARTESIAN_POINT ( 'NONE',  ( -19.97695672607123640, 40.00000000000000000, -58.81104016858105155 ) ) ;
#5247=CARTESIAN_POINT ( 'NONE',  ( 13.71368254939966036, 31.00000000000000355, -51.22554439249349656 ) ) ;
#5256=CARTESIAN_POINT ( 'NONE',  ( -4.090615425948576522, 40.00000000000000000, -62.39583333438447710 ) ) ;
#5264=CARTESIAN_POINT ( 'NONE',  ( -20.10416666680962550, 31.00000000000000355, -1.308996940106889273 ) ) ;
#5265=EDGE_CURVE ( 'NONE', #7867, #37436, #23095, .T. ) ;
#5267=CARTESIAN_POINT ( 'NONE',  ( 31.10108666877329853, 40.00000000000000000, 17.95223046116557697 ) ) ;
#5280=CARTESIAN_POINT ( 'NONE',  ( -54.99468034530342919, 31.00000000000000355, -62.86974495748531666 ) ) ;
#5291=CARTESIAN_POINT ( 'NONE',  ( 19.49047152472852673, 31.00000000000000355, -17.07028940128360261 ) ) ;
#5311=CARTESIAN_POINT ( 'NONE',  ( 33.88265278290065652, 40.00000000000000000, 16.77599488388066007 ) ) ;
#5341=CARTESIAN_POINT ( 'NONE',  ( 50.61746024623598572, 31.00000000000000355, -24.85206051842254737 ) ) ;
#5347=CARTESIAN_POINT ( 'NONE',  ( -44.72205690102931896, 40.00000000000000000, -58.47036224960022111 ) ) ;
#5355=DIRECTION ( 'NONE',  ( 0.000000000000000000, 1.000000000000000000, -1.060184893785364939E-15 ) ) ;
#5360=CARTESIAN_POINT ( 'NONE',  ( 29.59587406094124873, 31.00000000000000355, 60.01321678176139329 ) ) ;
#5372=CARTESIAN_POINT ( 'NONE',  ( 37.87019299815447937, 31.00000000000000355, -76.55254356380190472 ) ) ;
#5373=CARTESIAN_POINT ( 'NONE',  ( 11.20008397363331198, 40.00000000000000000, -84.14439686172906363 ) ) ;
#5392=CARTESIAN_POINT ( 'NONE',  ( 25.73918080462996372, 31.00000000000000355, -6.871072672212910959 ) ) ;
#5401=CARTESIAN_POINT ( 'NONE',  ( 40.10317558969867946, 40.00000000000000000, -23.06553963618951286 ) ) ;
#5408=EDGE_CURVE ( 'NONE', #5107, #19359, #27774, .T. ) ;
#5412=CARTESIAN_POINT ( 'NONE',  ( 33.70925502316616473, 31.00000000000000355, 11.43906998022225707 ) ) ;
#5420=CARTESIAN_POINT ( 'NONE',  ( -71.24862878704732339, 31.00000000000000711, 35.13526414049667324 ) ) ;
#5426=CARTESIAN_POINT ( 'NONE',  ( -51.89982240187124063, 31.00000000000000355, 3.308651922604603168 ) ) ;
#5427=CARTESIAN_POINT ( 'NONE',  ( 84.89583333414414312, 39.99999999999999289, -5.563236982362012029 ) ) ;
#5438=CARTESIAN_POINT ( 'NONE',  ( 62.17703816010947548, 39.99999999999999289, 21.10553973064489597 ) ) ;
#5470=CARTESIAN_POINT ( 'NONE',  ( -36.80126402429788612, 31.00000000000000355, 32.28896105221774349 ) ) ;
#5478=CARTESIAN_POINT ( 'NONE',  ( -57.67632858778466698, 40.00000000000000711, 15.45560639130400205 ) ) ;
#5485=CARTESIAN_POINT ( 'NONE',  ( -39.53383601736616271, 40.00000000000000000, 5.215339288884301538 ) ) ;
#5500=CARTESIAN_POINT ( 'NONE',  ( 5.650912336215120568, 31.00000000000000355, -84.59266001507907617 ) ) ;
#5509=DIRECTION ( 'NONE',  ( -0.06345332152672161774, 0.000000000000000000, 0.9979848074931934043 ) ) ;
#5511=CARTESIAN_POINT ( 'NONE',  ( 20.65150112226810819, 31.00000000000000355, -15.81946110361252522 ) ) ;
#5521=CARTESIAN_POINT ( 'NONE',  ( -31.57754862722326905, 31.00000000000000355, 93.01713655900283584 ) ) ;
#5525=CARTESIAN_POINT ( 'NONE',  ( 23.12883206328222130, 40.00000000000000000, 11.39561251172168355 ) ) ;
#5526=CARTESIAN_POINT ( 'NONE',  ( -5.264430561742839743, 40.00000000000000000, 39.44269128746232411 ) ) ;
#5536=DIRECTION ( 'NONE',  ( 0.06345332152672161774, -5.286866677681789116E-16, -0.9979848074931934043 ) ) ;
#5555=CARTESIAN_POINT ( 'NONE',  ( -49.80813925210023996, 31.00000000000000355, -17.00652635548579994 ) ) ;
#5560=CARTESIAN_POINT ( 'NONE',  ( 8.965261019434027645, 40.00000000000000000, 68.85524230650666766 ) ) ;
#5569=CARTESIAN_POINT ( 'NONE',  ( -15.99999999999997691, 17.11489954122026447, -4.499999999999995559 ) ) ;
#5571=CARTESIAN_POINT ( 'NONE',  ( -66.92166868300088822, 31.00000000000000711, -22.71661802240650019 ) ) ;
#5574=ORIENTED_EDGE ( 'NONE', *, *, #5265, .F. ) ;
#5580=CARTESIAN_POINT ( 'NONE',  ( 86.58052584568748955, 31.00000000000000000, -42.55516686010645344 ) ) ;
#5581=CARTESIAN_POINT ( 'NONE',  ( 49.34100556531813453, 40.00000000000000000, 85.68208892729249726 ) ) ;
#5607=CARTESIAN_POINT ( 'NONE',  ( 30.22238470470974292, 40.00000000000000000, -34.33595424619393555 ) ) ;
#5620=CARTESIAN_POINT ( 'NONE',  ( -19.20510714644778361, 31.00000000000000355, 33.27066566623395261 ) ) ;
#5626=CARTESIAN_POINT ( 'NONE',  ( -39.09256291070916944, 31.00000000000000355, 79.30589209199378331 ) ) ;
#5629=CARTESIAN_POINT ( 'NONE',  ( 44.54779904930365575, 31.00000000000000355, -34.05916983163054113 ) ) ;
#5637=ORIENTED_EDGE ( 'NONE', *, *, #5408, .T. ) ;
#5643=CARTESIAN_POINT ( 'NONE',  ( -47.15756294055117337, 40.00000000000000000, -53.75246728999482571 ) ) ;
#5671=CARTESIAN_POINT ( 'NONE',  ( 34.44467569804516671, 31.00000000000000355, 44.88666365967159777 ) ) ;
#5680=CARTESIAN_POINT ( 'NONE',  ( -27.38011802910879311, 40.00000000000000000, -55.51905197969063011 ) ) ;
#5689=CARTESIAN_POINT ( 'NONE',  ( -46.94946386092573221, 40.00000000000000000, 15.94926099647653928 ) ) ;
#5694=DIRECTION ( 'NONE',  ( 0.000000000000000000, 0.000000000000000000, 1.000000000000000000 ) ) ;
#5702=CARTESIAN_POINT ( 'NONE',  ( 86.62806645044915399, 31.00000000000000000, 11.52843970785434990 ) ) ;
#5725=CARTESIAN_POINT ( 'NONE',  ( 1.799870782497353439, 40.00000000000000000, 27.39583333577991908 ) ) ;
#5726=CARTESIAN_POINT ( 'NONE',  ( 27.04960320298795651, 40.00000000000000000, -23.64836272119224247 ) ) ;
#5747=CARTESIAN_POINT ( 'NONE',  ( 83.17098260925966713, 39.99999999999999289, 48.02127090943169208 ) ) ;
#5750=EDGE_CURVE ( 'NONE', #10114, #6578, #10501, .T. ) ;
#5754=CARTESIAN_POINT ( 'NONE',  ( -32.53655534684842365, 31.00000000000000355, -42.55839752837237455 ) ) ;
#5761=CARTESIAN_POINT ( 'NONE',  ( 74.90833963778730720, 39.99999999999999289, 20.17845691863183077 ) ) ;
#5772=ADVANCED_FACE ( 'NONE', ( #27102 ), #37105, .T. ) ;
#5773=CARTESIAN_POINT ( 'NONE',  ( 62.17703816010947548, 31.00000000000000000, 21.10553973062999589 ) ) ;
#5783=DIRECTION ( 'NONE',  ( 0.000000000000000000, 1.000000000000000000, -1.060184893785364939E-15 ) ) ;
#5784=CARTESIAN_POINT ( 'NONE',  ( -91.21105805184879500, 31.00000000000000711, 11.89862498597365104 ) ) ;
#5785=CARTESIAN_POINT ( 'NONE',  ( -6.060882879309179572, 40.00000000000000000, -94.40013096063921694 ) ) ;
#5804=CARTESIAN_POINT ( 'NONE',  ( -7.718844055051848230, 31.00000000000000355, -22.75659427661714673 ) ) ;
#5813=CARTESIAN_POINT ( 'NONE',  ( -32.60815990948594134, 40.00000000000000000, 24.92795611697640368 ) ) ;
#5826=CARTESIAN_POINT ( 'NONE',  ( 35.10416666475790493, 31.00000000000000355, 2.290744634698880233 ) ) ;
#5833=CARTESIAN_POINT ( 'NONE',  ( -23.88228986782336349, 31.00000000000000355, -89.13686966975919290 ) ) ;
#5836=EDGE_LOOP ( 'NONE', ( #23350, #23842, #40671, #35473 ) ) ;
#5837=CARTESIAN_POINT ( 'NONE',  ( -54.47698434024490410, 31.00000000000000355, -31.57393205620728693 ) ) ;
#5838=CARTESIAN_POINT ( 'NONE',  ( -47.50570208456527865, 40.00000000000000000, -41.80188021843024870 ) ) ;
#5839=CARTESIAN_POINT ( 'NONE',  ( 90.64482129758324902, 39.99999999999999289, 30.77200948131585889 ) ) ;
#5852=CARTESIAN_POINT ( 'NONE',  ( -68.69954721042445556, 40.00000000000000711, 39.68009708086182741 ) ) ;
#5872=CARTESIAN_POINT ( 'NONE',  ( -101.9145453900124068, 40.00000000000000000, -1.407535261550463268 ) ) ;
#5881=CARTESIAN_POINT ( 'NONE',  ( 57.76613438074698337, 31.00000000000000000, -28.48799604501563110 ) ) ;
#5884=CARTESIAN_POINT ( 'NONE',  ( -10.41556553088919834, 31.00000000000000355, 38.62046602036556209 ) ) ;
#5885=CARTESIAN_POINT ( 'NONE',  ( -65.92798595308768483, 40.00000000000000711, 22.39357416381200849 ) ) ;
#5889=EDGE_CURVE ( 'NONE', #3181, #5107, #40578, .T. ) ;
#5896=CARTESIAN_POINT ( 'NONE',  ( 28.83751338862256119, 40.00000000000000000, -32.88701605462710376 ) ) ;
#5911=CARTESIAN_POINT ( 'NONE',  ( -82.09281090897877675, 31.00000000000000711, -5.486092462564049477 ) ) ;
#5918=CARTESIAN_POINT ( 'NONE',  ( -101.1468392228030098, 40.00000000000000711, 13.20405500234329921 ) ) ;
#5927=CARTESIAN_POINT ( 'NONE',  ( -8.325335757348113930, 31.00000000000000355, -31.05587074991522201 ) ) ;
#5933=CARTESIAN_POINT ( 'NONE',  ( -39.53383601736616271, 40.00000000000000000, 5.215339288884301538 ) ) ;
#5934=CARTESIAN_POINT ( 'NONE',  ( 36.20216622922067984, 40.00000000000000000, 9.761693653842600682 ) ) ;
#5966=CARTESIAN_POINT ( 'NONE',  ( -48.87578956997907653, 31.00000000000000355, 16.50293044076727611 ) ) ;
#5977=CARTESIAN_POINT ( 'NONE',  ( -58.00742674161275403, 40.00000000000000711, -44.63796826977546317 ) ) ;
#5988=CARTESIAN_POINT ( 'NONE',  ( 44.85399723358655422, 31.00000000000000355, -58.47732767552992073 ) ) ;
#6003=CARTESIAN_POINT ( 'NONE',  ( -32.34013556242301490, 31.00000000000000355, 94.87070470182929682 ) ) ;
#6005=CARTESIAN_POINT ( 'NONE',  ( 6.386360208629404234, 40.00000000000000000, 99.40013590833049761 ) ) ;
#6020=EDGE_LOOP ( 'NONE', ( #42361, #27556, #1621, #16749 ) ) ;
#6022=CARTESIAN_POINT ( 'NONE',  ( 11.19416946702030735, 31.00000000000000355, -22.66942529387728555 ) ) ;
#6035=CARTESIAN_POINT ( 'NONE',  ( 38.14553738578516828, 40.00000000000000000, 29.36968266378342207 ) ) ;
#6048=CARTESIAN_POINT ( 'NONE',  ( 39.78947517253659072, 31.00000000000000355, -19.62497191778171413 ) ) ;
#6049=PRESENTATION_STYLE_ASSIGNMENT (( #38984 ) ) ;
#6054=CARTESIAN_POINT ( 'NONE',  ( -78.83182461418512332, 31.00000000000000711, -45.51551753872077910 ) ) ;
#6058=CARTESIAN_POINT ( 'NONE',  ( 49.67886955982877595, 31.00000000000000355, -43.43868092391004865 ) ) ;
#6059=CARTESIAN_POINT ( 'NONE',  ( -38.62815422673675414, 40.00000000000000000, -50.51519254952906124 ) ) ;
#6073=CARTESIAN_POINT ( 'NONE',  ( 66.75446398494719347, 39.99999999999999289, -32.91950810868348043 ) ) ;
#6089=AXIS2_PLACEMENT_3D ( 'NONE', #38053, #5103, #8382 ) ;
#6105=CARTESIAN_POINT ( 'NONE',  ( -19.97695672607123640, 31.00000000000000355, -58.81104016858105155 ) ) ;
#6108=CARTESIAN_POINT ( 'NONE',  ( -20.36888183406315278, 31.00000000000000355, -26.63352584488936614 ) ) ;
#6109=CARTESIAN_POINT ( 'NONE',  ( 36.74538074116732389, 40.00000000000000000, -63.64477163140654170 ) ) ;
#6118=CARTESIAN_POINT ( 'NONE',  ( 43.19851606872948935, 40.00000000000000000, 14.66122656362567689 ) ) ;
#6134=CARTESIAN_POINT ( 'NONE',  ( 64.90225467581601038, 31.00000000000000000, 74.17428024387139374 ) ) ;
#6140=VERTEX_POINT ( 'NONE', #2594 ) ;
#6146=VECTOR ( 'NONE', #42494, 1000.000000000000000 ) ;
#6152=CARTESIAN_POINT ( 'NONE',  ( 19.70274684888802952, 31.00000000000000355, 17.27304525429847359 ) ) ;
#6159=CARTESIAN_POINT ( 'NONE',  ( -35.44024466369167925, 40.00000000000000000, -20.45798383175513635 ) ) ;
#6161=CARTESIAN_POINT ( 'NONE',  ( 23.40755275317130568, 40.00000000000000000, 30.61714766194360848 ) ) ;
#6188=CARTESIAN_POINT ( 'NONE',  ( 56.82522199878360425, 31.00000000000000355, 7.581518937762241173 ) ) ;
#6195=CARTESIAN_POINT ( 'NONE',  ( 50.06853320189533463, 39.99999999999999289, -56.91684085114077618 ) ) ;
#6205=CARTESIAN_POINT ( 'NONE',  ( -79.89583333417640176, 31.00000000000000711, 5.235987747608064957 ) ) ;
#6219=CARTESIAN_POINT ( 'NONE',  ( 64.90225467581601038, 31.00000000000000000, 74.17428024387139374 ) ) ;
#6220=CARTESIAN_POINT ( 'NONE',  ( -30.16842255227261660, 40.00000000000000000, -89.21315370691763746 ) ) ;
#6230=VERTEX_POINT ( 'NONE', #36192 ) ;
#6237=CARTESIAN_POINT ( 'NONE',  ( 19.49047152472852673, 31.00000000000000355, -17.07028940128360261 ) ) ;
#6247=CARTESIAN_POINT ( 'NONE',  ( -32.45554871466747215, 40.00000000000000000, -28.56710966684967090 ) ) ;
#6257=CARTESIAN_POINT ( 'NONE',  ( -47.94314659152439617, 31.00000000000000355, -16.27230485535717719 ) ) ;
#6258=FILL_AREA_STYLE ('',( #18984 ) ) ;
#6261=CARTESIAN_POINT ( 'NONE',  ( -81.55297449308174862, 31.00000000000000711, -40.20044092665353475 ) ) ;
#6267=CARTESIAN_POINT ( 'NONE',  ( -20.51812799676685373, 31.00000000000000355, -60.74091093256831897 ) ) ;
#6269=CARTESIAN_POINT ( 'NONE',  ( 64.03668805593822810, 39.99999999999999289, 21.85318084037336561 ) ) ;
#6270=CARTESIAN_POINT ( 'NONE',  ( 86.04713929520032423, 39.99999999999999289, 42.41619695850760507 ) ) ;
#6281=CARTESIAN_POINT ( 'NONE',  ( -69.75709431192164800, 40.00000000000000711, -9.183449035091399537 ) ) ;
#6311=CARTESIAN_POINT ( 'NONE',  ( -4.090615425948576522, 31.00000000000000355, -62.39583333438447710 ) ) ;
#6316=CARTESIAN_POINT ( 'NONE',  ( -28.46928290085317315, 31.00000000000000355, -16.49637127829624106 ) ) ;
#6319=CARTESIAN_POINT ( 'NONE',  ( -70.10416666575086708, 40.00000000000000711, -4.581489278090966621 ) ) ;
#6330=CARTESIAN_POINT ( 'NONE',  ( 3.108867721649529958, 40.00000000000000000, 47.39583333474234905 ) ) ;
#6332=DIRECTION ( 'NONE',  ( 0.9654856287475623855, 0.000000000000000000, -0.2604563316218754254 ) ) ;
#6342=CARTESIAN_POINT ( 'NONE',  ( 49.34100556531812742, 31.00000000000000355, 85.68208892729249726 ) ) ;
#6359=CARTESIAN_POINT ( 'NONE',  ( -7.231618336280544845, 31.00000000000000355, 27.02512817425793656 ) ) ;
#6368=CARTESIAN_POINT ( 'NONE',  ( -29.26739590608564967, 40.00000000000000000, 25.68069354617348665 ) ) ;
#6369=CARTESIAN_POINT ( 'NONE',  ( -6.590854309045714565, 40.00000000000000000, 49.37518673228670707 ) ) ;
#6383=CIRCLE ( 'NONE', #12000, 4.500000000000002665 ) ;
#6395=LINE ( 'NONE', #9244, #41776 ) ;
#6397=CARTESIAN_POINT ( 'NONE',  ( 18.91139405008774688, 31.00000000000000355, 55.99505798891475195 ) ) ;
#6404=CARTESIAN_POINT ( 'NONE',  ( 86.62806645044916820, 39.99999999999999289, 11.52843970785434990 ) ) ;
#6415=CARTESIAN_POINT ( 'NONE',  ( -53.76583044639610165, 31.00000000000000355, -61.28633540801820345 ) ) ;
#6425=CARTESIAN_POINT ( 'NONE',  ( -12.22491041698737746, 31.00000000000000355, -93.69500887688226953 ) ) ;
#6444=CARTESIAN_POINT ( 'NONE',  ( -31.36635120280995537, 31.00000000000000355, -8.451140850656344128 ) ) ;
#6453=CARTESIAN_POINT ( 'NONE',  ( 50.61746024623599993, 40.00000000000000000, -24.85206051842255093 ) ) ;
#6462=CARTESIAN_POINT ( 'NONE',  ( 3.436116956419347002, 31.00000000000000355, -52.60416666537189911 ) ) ;
#6468=CARTESIAN_POINT ( 'NONE',  ( -55.79431841392906222, 31.00000000000000355, -72.71543055464235294 ) ) ;
#6471=CARTESIAN_POINT ( 'NONE',  ( -4.113979049837550583, 31.00000000000000355, -64.40000927351897531 ) ) ;
#6472=CARTESIAN_POINT ( 'NONE',  ( -4.660665814384791439, 40.00000000000000000, 69.59371722953135020 ) ) ;
#6473=CARTESIAN_POINT ( 'NONE',  ( 63.67823170517923614, 39.99999999999999289, 72.58713758494482704 ) ) ;
#6483=EDGE_CURVE ( 'NONE', #6869, #38968, #9266, .T. ) ;
#6486=CARTESIAN_POINT ( 'NONE',  ( -104.8158553526607477, 40.00000000000000711, 3.963965400206364453 ) ) ;
#6487=CARTESIAN_POINT ( 'NONE',  ( -39.25113411183426848, 40.00000000000000000, 67.98392962655870519 ) ) ;
#6517=CARTESIAN_POINT ( 'NONE',  ( -7.547223091130065953, 31.00000000000000355, 57.33767041057931380 ) ) ;
#6519=ORIENTED_EDGE ( 'NONE', *, *, #36834, .T. ) ;
#6520=CARTESIAN_POINT ( 'NONE',  ( -17.88900094061790469, 31.00000000000000355, 36.12696699725170646 ) ) ;
#6522=CARTESIAN_POINT ( 'NONE',  ( 57.13603463884887645, 40.00000000000000000, 32.98675068510902264 ) ) ;
#6530=CARTESIAN_POINT ( 'NONE',  ( -31.00354902519490352, 40.00000000000000000, -27.18544651223506392 ) ) ;
#6546=CARTESIAN_POINT ( 'NONE',  ( 96.90013369365226481, 31.00000000000000000, -6.223598210838602540 ) ) ;
#6553=CYLINDRICAL_SURFACE ( 'NONE', #31014, 2.500000000000000444 ) ;
#6561=CARTESIAN_POINT ( 'NONE',  ( -19.99999999999999645, 31.00000000000000355, 0.000000000000000000 ) ) ;
#6564=CARTESIAN_POINT ( 'NONE',  ( -28.63582912838407069, 31.00000000000000355, 7.677129336082076705 ) ) ;
#6571=CARTESIAN_POINT ( 'NONE',  ( -22.00000000000000000, 17.11489954122026447, 1.283214542831021765 ) ) ;
#6572=CARTESIAN_POINT ( 'NONE',  ( -9.824444021593908616, 40.00000000000000000, 36.70529466175499778 ) ) ;
#6573=CARTESIAN_POINT ( 'NONE',  ( 46.89968353242633015, 40.00000000000000000, -2.988513402017745069 ) ) ;
#6578=VERTEX_POINT ( 'NONE', #39780 ) ;
#6602=CARTESIAN_POINT ( 'NONE',  ( 15.22596115864829791, 31.00000000000000355, 57.21640888978779316 ) ) ;
#6614=CARTESIAN_POINT ( 'NONE',  ( 86.90011881125597881, 39.99999999999999289, -5.573058087428396590 ) ) ;
#6617=DIRECTION ( 'NONE',  ( 0.000000000000000000, -1.000000000000000000, 5.297542245118643184E-16 ) ) ;
#6627=CARTESIAN_POINT ( 'NONE',  ( 24.81019160154284720, 31.00000000000000355, 73.04493173762017477 ) ) ;
#6633=ORIENTED_EDGE ( 'NONE', *, *, #3820, .F. ) ;
#6647=DIRECTION ( 'NONE',  ( -0.06345332152672161774, 1.058048417131579272E-15, 0.9979848074931934043 ) ) ;
#6660=CARTESIAN_POINT ( 'NONE',  ( -2.197745971918068530, 31.00000000000000355, -34.39891587002171036 ) ) ;
#6668=CARTESIAN_POINT ( 'NONE',  ( 48.78760054484346398, 40.00000000000000000, -28.06521077754944926 ) ) ;
#6685=CARTESIAN_POINT ( 'NONE',  ( -29.60425243605831724, 31.00000000000000355, 38.59963703562669934 ) ) ;
#6693=CARTESIAN_POINT ( 'NONE',  ( -18.08361268445098347, 40.00000000000000000, -10.43497034982449456 ) ) ;
#6697=CARTESIAN_POINT ( 'NONE',  ( 66.75914267695947046, 31.00000000000000000, 8.899205196610871837 ) ) ;
#6698=CARTESIAN_POINT ( 'NONE',  ( 40.05902963217418744, 40.00000000000000000, -52.04757428485088866 ) ) ;
#6713=CARTESIAN_POINT ( 'NONE',  ( 50.95389515256417923, 40.00000000000000000, -66.42840393140320998 ) ) ;
#6725=CARTESIAN_POINT ( 'NONE',  ( 23.62253089228586944, 40.00000000000000000, -11.62353008834529255 ) ) ;
#6745=CARTESIAN_POINT ( 'NONE',  ( 66.75446398494719347, 31.00000000000000000, -32.91950810868348043 ) ) ;
#6749=CARTESIAN_POINT ( 'NONE',  ( 27.04960320298028620, 31.00000000000000355, -23.64836272119223892 ) ) ;
#6750=CARTESIAN_POINT ( 'NONE',  ( -56.48955861152074220, 40.00000000000000711, -43.32902275383659685 ) ) ;
#6757=ORIENTED_EDGE ( 'NONE', *, *, #20205, .F. ) ;
#6762=CARTESIAN_POINT ( 'NONE',  ( -46.87443272357899815, 40.00000000000000000, 35.96965017775951878 ) ) ;
#6767=DIRECTION ( 'NONE',  ( 0.000000000000000000, -1.000000000000000000, 5.297542245118643184E-16 ) ) ;
#6771=ORIENTED_EDGE ( 'NONE', *, *, #3696, .F. ) ;
#6778=CARTESIAN_POINT ( 'NONE',  ( -24.28006566512905451, 31.00000000000000355, -91.10131089348453770 ) ) ;
#6793=CARTESIAN_POINT ( 'NONE',  ( 8.528031178950213231, 31.00000000000000355, -31.86521141804621493 ) ) ;
#6800=CARTESIAN_POINT ( 'NONE',  ( -18.51709390187839688, 40.00000000000000000, -37.54239277154294996 ) ) ;
#6802=CARTESIAN_POINT ( 'NONE',  ( -41.03896728212566103, 40.00000000000000000, -11.06873348903577892 ) ) ;
#6812=EDGE_CURVE ( 'NONE', #17691, #41039, #4879, .T. ) ;
#6830=CARTESIAN_POINT ( 'NONE',  ( -19.43072497042362556, 31.00000000000000355, 56.92208038676059800 ) ) ;
#6840=CARTESIAN_POINT ( 'NONE',  ( 20.39742982868580157, 40.00000000000000000, 76.57971376067894198 ) ) ;
#6851=CARTESIAN_POINT ( 'NONE',  ( -75.41724699911947027, 31.00000000000000711, 25.61573074746135248 ) ) ;
#6869=VERTEX_POINT ( 'NONE', #17581 ) ;
#6880=CARTESIAN_POINT ( 'NONE',  ( 35.42814233785335176, 31.00000000000000355, -9.427541829740359702 ) ) ;
#6887=CARTESIAN_POINT ( 'NONE',  ( -42.11670055800494339, 40.00000000000000000, -32.42481051986320040 ) ) ;
#6897=CARTESIAN_POINT ( 'NONE',  ( -49.88601606984090608, 31.00000000000000355, -6.565487524765669214 ) ) ;
#6902=CARTESIAN_POINT ( 'NONE',  ( -15.93581279029885422, 40.00000000000000000, -13.96891150189262021 ) ) ;
#6905=CARTESIAN_POINT ( 'NONE',  ( 10.26812810425290579, 31.00000000000000355, 78.79123036457541218 ) ) ;
#6906=CARTESIAN_POINT ( 'NONE',  ( -73.09555549758189841, 40.00000000000000711, 35.91380138263622257 ) ) ;
#6925=CARTESIAN_POINT ( 'NONE',  ( 38.45889818826288575, 40.00000000000000000, 77.98987599019784511 ) ) ;
#6936=CARTESIAN_POINT ( 'NONE',  ( 26.62151981922250243, 40.00000000000000000, -3.482817046706076169 ) ) ;
#6947=SURFACE_STYLE_USAGE ( .BOTH. , #27864 ) ;
#6951=CARTESIAN_POINT ( 'NONE',  ( -13.09503298281258132, 31.00000000000000355, -17.05789676611946959 ) ) ;
#6957=CARTESIAN_POINT ( 'NONE',  ( -47.15756294055117337, 31.00000000000000355, -53.75246728999482571 ) ) ;
#6959=CARTESIAN_POINT ( 'NONE',  ( 20.11321884379921343, 31.00000000000000355, -40.61652209561064097 ) ) ;
#6961=CARTESIAN_POINT ( 'NONE',  ( -47.90394619311608437, 40.00000000000000000, 62.45286580340285099 ) ) ;
#6970=CARTESIAN_POINT ( 'NONE',  ( -35.70415035507907930, 40.00000000000000000, 46.55071329160319493 ) ) ;
#6985=CARTESIAN_POINT ( 'NONE',  ( -79.17211737996690601, 31.00000000000000711, 45.58486055166099504 ) ) ;
#7003=CARTESIAN_POINT ( 'NONE',  ( 31.10108666877329853, 31.00000000000000355, 17.95223046116557697 ) ) ;
#7013=CARTESIAN_POINT ( 'NONE',  ( 20.73284993368543638, 40.00000000000000000, 42.03655757353646294 ) ) ;
#7015=CARTESIAN_POINT ( 'NONE',  ( -41.92568936861482598, 40.00000000000000000, -5.596851440153165491 ) ) ;
#7022=CARTESIAN_POINT ( 'NONE',  ( 24.63052733448982323, 40.00000000000000000, -3.251868155982907904 ) ) ;
#7032=ORIENTED_EDGE ( 'NONE', *, *, #34378, .T. ) ;
#7040=CARTESIAN_POINT ( 'NONE',  ( 52.50410707182467718, 31.00000000000000000, -40.15145572480454916 ) ) ;
#7047=CARTESIAN_POINT ( 'NONE',  ( -64.43604943162229404, 40.00000000000000711, 49.29347324003091302 ) ) ;
#7060=CARTESIAN_POINT ( 'NONE',  ( 84.66040299356156140, 31.00000000000000000, 11.14692016787551765 ) ) ;
#7063=VERTEX_POINT ( 'NONE', #27112 ) ;
#7090=CARTESIAN_POINT ( 'NONE',  ( 9.106956811745659408, 31.00000000000000355, -33.78410985267935018 ) ) ;
#7098=CARTESIAN_POINT ( 'NONE',  ( -51.85848278221650531, 40.00000000000000000, -6.921372802089502230 ) ) ;
#7113=CARTESIAN_POINT ( 'NONE',  ( 4.090615425948669781, 31.00000000000000355, -62.60416666561555132 ) ) ;
#7118=CARTESIAN_POINT ( 'NONE',  ( -65.18298466990795248, 31.00000000000000711, 74.32329070269128124 ) ) ;
#7122=CARTESIAN_POINT ( 'NONE',  ( 73.52353481979008620, 31.00000000000000000, 25.08131146961490998 ) ) ;
#7123=CARTESIAN_POINT ( 'NONE',  ( 77.09314031436157677, 39.99999999999999289, 5.156213784760051766 ) ) ;
#7138=CARTESIAN_POINT ( 'NONE',  ( -21.28946418274055929, 40.00000000000000000, -79.45670318283352174 ) ) ;
#7162=CARTESIAN_POINT ( 'NONE',  ( -9.654069774896838041, 31.00000000000000355, -19.56573356436190636 ) ) ;
#7165=AXIS2_PLACEMENT_3D ( 'NONE', #8011, #21808, #2096 ) ;
#7168=CARTESIAN_POINT ( 'NONE',  ( -41.80404827410195168, 31.00000000000000355, 54.50178954758867889 ) ) ;
#7172=CARTESIAN_POINT ( 'NONE',  ( 12.64472494877221997, 31.00000000000000355, 47.53373494968589341 ) ) ;
#7173=CARTESIAN_POINT ( 'NONE',  ( -5.399612364985466151, 40.00000000000000000, -82.39583333413678190 ) ) ;
#7182=CARTESIAN_POINT ( 'NONE',  ( -15.01009539198478748, 40.00000000000000000, 56.06562763604418365 ) ) ;
#7187=CARTESIAN_POINT ( 'NONE',  ( -17.44537629401975920, 31.00000000000000711, 4.261559264950522952 ) ) ;
#7210=CARTESIAN_POINT ( 'NONE',  ( -19.99999999999999645, 17.11489954122026447, 0.000000000000000000 ) ) ;
#7216=CARTESIAN_POINT ( 'NONE',  ( -35.29531037056285214, 31.00000000000000355, 17.40921588598563119 ) ) ;
#7224=CARTESIAN_POINT ( 'NONE',  ( 48.77780477658175329, 40.00000000000000000, -24.05648398140741406 ) ) ;
#7225=CARTESIAN_POINT ( 'NONE',  ( 6.367266499441480931, 40.00000000000000000, 48.98256792610028754 ) ) ;
#7232=CARTESIAN_POINT ( 'NONE',  ( -19.47536345555549886, 40.00000000000000000, -6.605835105517199324 ) ) ;
#7250=CARTESIAN_POINT ( 'NONE',  ( -31.81746463534672387, 31.00000000000000355, -55.29958784370775504 ) ) ;
#7258=CARTESIAN_POINT ( 'NONE',  ( -30.16842255227261660, 40.00000000000000000, -89.21315370691763746 ) ) ;
#7272=CARTESIAN_POINT ( 'NONE',  ( 12.12865573427490062, 31.00000000000000355, -92.11205733446308841 ) ) ;
#7280=FACE_OUTER_BOUND ( 'NONE', #36602, .T. ) ;
#7294=DIRECTION ( 'NONE',  ( 0.000000000000000000, -1.000000000000000000, 5.297542245118643184E-16 ) ) ;
#7297=AXIS2_PLACEMENT_3D ( 'NONE', #21167, #33998, #27459 ) ;
#7302=CARTESIAN_POINT ( 'NONE',  ( 1.888402776346428835, 31.00000000000000355, 29.39821258742166066 ) ) ;
#7310=CARTESIAN_POINT ( 'NONE',  ( 46.08863070263672057, 40.00000000000000000, 35.47900410130833393 ) ) ;
#7322=CARTESIAN_POINT ( 'NONE',  ( 50.09382087749727930, 31.00000000000000355, 24.69014870349942825 ) ) ;
#7332=CARTESIAN_POINT ( 'NONE',  ( -25.38139813252123034, 31.00000000000000355, 94.78629358389331117 ) ) ;
#7338=CARTESIAN_POINT ( 'NONE',  ( -36.82253293460209420, 31.00000000000000355, -63.98115709646774718 ) ) ;
#7340=CARTESIAN_POINT ( 'NONE',  ( -55.03444096782886419, 40.00000000000000000, -48.41538206857744342 ) ) ;
#7357=CARTESIAN_POINT ( 'NONE',  ( -40.93297376624923345, 40.00000000000000000, -70.86912620794510076 ) ) ;
#7360=DIRECTION ( 'NONE',  ( -0.9470131699890049770, -3.405258028344997528E-16, -0.3211947320043963550 ) ) ;
#7385=CARTESIAN_POINT ( 'NONE',  ( 22.42277067908921850, 31.00000000000000355, 12.94072372014797701 ) ) ;
#7390=CARTESIAN_POINT ( 'NONE',  ( 49.83821931962687302, 31.00000000000000355, 43.70611527624207326 ) ) ;
#7393=CARTESIAN_POINT ( 'NONE',  ( -38.37160831357631707, 31.00000000000000355, -19.00137192356237392 ) ) ;
#7395=CARTESIAN_POINT ( 'NONE',  ( -61.13902149641835138, 40.00000000000000000, -53.61851653479526902 ) ) ;
#7413=CARTESIAN_POINT ( 'NONE',  ( 42.89889459577944564, 40.00000000000000000, -32.91970121835214513 ) ) ;
#7443=CARTESIAN_POINT ( 'NONE',  ( -31.00354902519490352, 31.00000000000000355, -27.18544651223506392 ) ) ;
#7449=CARTESIAN_POINT ( 'NONE',  ( -42.66459923921424036, 40.00000000000000000, 24.64557685607233140 ) ) ;
#7450=CARTESIAN_POINT ( 'NONE',  ( -48.52617905696451572, 40.00000000000000000, 37.10499320822106029 ) ) ;
#7462=CARTESIAN_POINT ( 'NONE',  ( -28.63582912838407069, 40.00000000000000000, 7.677129336082076705 ) ) ;
#7480=CARTESIAN_POINT ( 'NONE',  ( 76.90008882636698218, 31.00000000000000000, -4.923574515426284215 ) ) ;
#7486=CARTESIAN_POINT ( 'NONE',  ( 24.72345498302142630, 40.00000000000000000, -91.84610802670698604 ) ) ;
#7500=CARTESIAN_POINT ( 'NONE',  ( -5.726861599740728614, 31.00000000000000355, 87.60416666588449175 ) ) ;
#7504=CARTESIAN_POINT ( 'NONE',  ( 3.245924575715140481, 40.00000000000000000, -24.54795925723446359 ) ) ;
#7535=CARTESIAN_POINT ( 'NONE',  ( -11.35616125661755937, 31.00000000000000355, -42.69191301634815261 ) ) ;
#7542=CARTESIAN_POINT ( 'NONE',  ( 3.791180027291366272, 40.00000000000000000, 59.39995347152935778 ) ) ;
#7552=CARTESIAN_POINT ( 'NONE',  ( -53.27196957865878346, 31.00000000000000711, 26.27224001321920355 ) ) ;
#7560=CARTESIAN_POINT ( 'NONE',  ( 7.411374251232441424, 40.00000000000000000, -21.84767871671174788 ) ) ;
#7564=CARTESIAN_POINT ( 'NONE',  ( -69.31868535681203980, 31.00000000000000711, 18.45717643660088214 ) ) ;
#7565=CARTESIAN_POINT ( 'NONE',  ( 72.60479858918233731, 39.99999999999999289, -24.53750584076950858 ) ) ;
#7579=CARTESIAN_POINT ( 'NONE',  ( 57.06996419936330511, 39.99999999999999289, 65.05326946697847745 ) ) ;
#7593=CARTESIAN_POINT ( 'NONE',  ( 30.20675218207097501, 40.00000000000000000, 23.25504409023340813 ) ) ;
#7595=FACE_OUTER_BOUND ( 'NONE', #9933, .T. ) ;
#7602=CARTESIAN_POINT ( 'NONE',  ( 16.14498194198480618, 31.00000000000000355, 21.03343489346954698 ) ) ;
#7609=CARTESIAN_POINT ( 'NONE',  ( -8.856203846296160975, 31.00000000000000355, 67.27320953167645712 ) ) ;
#7610=ORIENTED_EDGE ( 'NONE', *, *, #30321, .T. ) ;
#7612=CARTESIAN_POINT ( 'NONE',  ( 46.89194940766294906, 31.00000000000000355, 6.259973086888626526 ) ) ;
#7613=CARTESIAN_POINT ( 'NONE',  ( -64.44063486737354651, 40.00000000000000711, -49.42892067282641477 ) ) ;
#7625=CARTESIAN_POINT ( 'NONE',  ( -44.11856065373272173, 40.00000000000000000, -25.46949057303769948 ) ) ;
#7628=ORIENTED_EDGE ( 'NONE', *, *, #12975, .T. ) ;
#7642=DIRECTION ( 'NONE',  ( 0.000000000000000000, 0.000000000000000000, 1.000000000000000000 ) ) ;
#7657=CARTESIAN_POINT ( 'NONE',  ( 34.28525303991722240, 31.00000000000000355, 9.176237600273646322 ) ) ;
#7664=CARTESIAN_POINT ( 'NONE',  ( 3.108867721649529958, 40.00000000000000000, 47.39583333474234905 ) ) ;
#7665=CARTESIAN_POINT ( 'NONE',  ( -35.18788409414197815, 40.00000000000000000, -40.25400722681193599 ) ) ;
#7675=CARTESIAN_POINT ( 'NONE',  ( 16.14498194198480618, 40.00000000000000000, 21.03343489346954698 ) ) ;
#7689=CARTESIAN_POINT ( 'NONE',  ( 4.991138515316659863, 31.00000000000000355, -74.59332054773635434 ) ) ;
#7697=CARTESIAN_POINT ( 'NONE',  ( 22.98560153735141043, 40.00000000000000000, 86.26083236265425569 ) ) ;
#7713=CARTESIAN_POINT ( 'NONE',  ( -70.72766149062127283, 31.00000000000000711, 54.26934393422349956 ) ) ;
#7716=CARTESIAN_POINT ( 'NONE',  ( 3.798394181604433761, 40.00000000000000000, 29.10671710469611284 ) ) ;
#7717=ORIENTED_EDGE ( 'NONE', *, *, #11186, .T. ) ;
#7722=DIRECTION ( 'NONE',  ( 0.000000000000000000, 0.000000000000000000, 1.000000000000000000 ) ) ;
#7747=CARTESIAN_POINT ( 'NONE',  ( 24.31498657912377226, 31.00000000000000355, 42.27453502171529465 ) ) ;
#7753=CARTESIAN_POINT ( 'NONE',  ( -19.43072497041043079, 40.00000000000000000, 56.92208038676060511 ) ) ;
#7764=CARTESIAN_POINT ( 'NONE',  ( 28.40420691229738281, 31.00000000000000355, 49.17333623205379922 ) ) ;
#7768=CIRCLE ( 'NONE', #18944, 4.500000000000000888 ) ;
#7772=CARTESIAN_POINT ( 'NONE',  ( 8.528031178950213231, 40.00000000000000000, -31.86521141804621493 ) ) ;
#7778=CARTESIAN_POINT ( 'NONE',  ( -72.09351246574976813, 31.00000000000000711, -4.825959690424619808 ) ) ;
#7779=CARTESIAN_POINT ( 'NONE',  ( 61.98103557012430542, 39.99999999999999289, 47.69015029125304039 ) ) ;
#7791=CARTESIAN_POINT ( 'NONE',  ( 94.89583333399441756, 39.99999999999999289, -6.217735451874103703 ) ) ;
#7807=CARTESIAN_POINT ( 'NONE',  ( -10.89792128226954482, 40.00000000000000000, -32.25956908328721795 ) ) ;
#7817=CARTESIAN_POINT ( 'NONE',  ( -26.30698076681265363, 31.00000000000000355, 12.97770382244945253 ) ) ;
#7825=CARTESIAN_POINT ( 'NONE',  ( -61.13902149641835138, 31.00000000000000355, -53.61851653479526902 ) ) ;
#7827=CARTESIAN_POINT ( 'NONE',  ( 5.928665350384932253, 31.00000000000000355, -44.40877992884582426 ) ) ;
#7830=CARTESIAN_POINT ( 'NONE',  ( -36.24314215638268877, 40.00000000000000000, -73.49571118816069770 ) ) ;
#7840=CARTESIAN_POINT ( 'NONE',  ( -67.35649507452052376, 40.00000000000000711, 18.04843207638801772 ) ) ;
#7855=CARTESIAN_POINT ( 'NONE',  ( -44.52253807734693680, 31.00000000000000355, 90.03212995789276363 ) ) ;
#7867=VERTEX_POINT ( 'NONE', #39209 ) ;
#7871=CARTESIAN_POINT ( 'NONE',  ( -45.59965607524345899, 31.00000000000000355, -22.47439267160796916 ) ) ;
#7881=CARTESIAN_POINT ( 'NONE',  ( -3.108867721649295035, 40.00000000000000000, 47.60416666525765095 ) ) ;
#7882=CARTESIAN_POINT ( 'NONE',  ( 50.14038141241296387, 40.00000000000000000, 29.06424286984033145 ) ) ;
#7889=CARTESIAN_POINT ( 'NONE',  ( -27.97094176822542977, 40.00000000000000000, 9.504947828999611659 ) ) ;
#7907=CARTESIAN_POINT ( 'NONE',  ( -48.39074809477736494, 31.00000000000000355, -55.33250407651094349 ) ) ;
#7917=CARTESIAN_POINT ( 'NONE',  ( -80.50242771303932443, 40.00000000000000711, -46.62292012066232871 ) ) ;
#7927=CARTESIAN_POINT ( 'NONE',  ( -78.83182461418512332, 31.00000000000000711, -45.51551753872077910 ) ) ;
#7931=CARTESIAN_POINT ( 'NONE',  ( -28.12618851199097492, 40.00000000000000000, 13.81902982503211064 ) ) ;
#7939=VERTEX_POINT ( 'NONE', #6486 ) ;
#7959=CARTESIAN_POINT ( 'NONE',  ( 45.11287655886648906, 31.00000000000000355, -12.00022417491544324 ) ) ;
#7967=CARTESIAN_POINT ( 'NONE',  ( -8.314562429032193336, 40.00000000000000000, -63.88718494337742015 ) ) ;
#7979=CARTESIAN_POINT ( 'NONE',  ( -46.07128526072433772, 31.00000000000000355, -40.40198152342698990 ) ) ;
#7985=CARTESIAN_POINT ( 'NONE',  ( -1.799870782497340782, 40.00000000000000000, 27.60416666422008802 ) ) ;
#7989=CARTESIAN_POINT ( 'NONE',  ( 11.20008397362390618, 31.00000000000000355, -84.14439686172904942 ) ) ;
#7990=CARTESIAN_POINT ( 'NONE',  ( -10.92011822083620309, 40.00000000000000000, -83.75917815547794021 ) ) ;
#8007=CARTESIAN_POINT ( 'NONE',  ( 94.59594211465898184, 39.99999999999999289, 12.45590092308117569 ) ) ;
#8008=DIRECTION ( 'NONE',  ( -0.9247238835424298475, -2.016449031586420221E-16, -0.3806385939525924744 ) ) ;
#8011=CARTESIAN_POINT ( 'NONE',  ( -105.9879088449591933, 17.11489954122026447, -0.3807199291576673361 ) ) ;
#8020=CARTESIAN_POINT ( 'NONE',  ( -28.12618851199097492, 40.00000000000000000, 13.81902982503211064 ) ) ;
#8029=FACE_OUTER_BOUND ( 'NONE', #4233, .T. ) ;
#8034=CARTESIAN_POINT ( 'NONE',  ( -2.127120017302697619, 31.00000000000000355, -32.39583333539214038 ) ) ;
#8041=CARTESIAN_POINT ( 'NONE',  ( 81.87674480462379734, 31.00000000000000000, -21.93767060400471891 ) ) ;
#8042=ORIENTED_EDGE ( 'NONE', *, *, #28981, .F. ) ;
#8043=CARTESIAN_POINT ( 'NONE',  ( -13.93478910046839125, 31.00000000000000355, -52.37520058406987999 ) ) ;
#8044=CARTESIAN_POINT ( 'NONE',  ( -89.89583333403318477, 40.00000000000000711, 5.890486217120591839 ) ) ;
#8058=CARTESIAN_POINT ( 'NONE',  ( 20.30000058474805869, 40.00000000000000000, -59.80472289869057789 ) ) ;
#8075=CARTESIAN_POINT ( 'NONE',  ( -50.38378093998269946, 31.00000000000000711, 87.00968337440518496 ) ) ;
#8091=CARTESIAN_POINT ( 'NONE',  ( -38.53741714288415210, 31.00000000000000355, -33.79371401777069650 ) ) ;
#8103=CARTESIAN_POINT ( 'NONE',  ( -29.22812062908682051, 40.00000000000000000, 50.62729764625685647 ) ) ;
#8104=CARTESIAN_POINT ( 'NONE',  ( -58.36801134196149832, 40.00000000000000711, 19.71467013091580256 ) ) ;
#8109=CARTESIAN_POINT ( 'NONE',  ( -10.86393331615775892, 31.00000000000000355, -18.79923026442779843 ) ) ;
#8112=CARTESIAN_POINT ( 'NONE',  ( 34.98270738856093232, 40.00000000000000000, 4.602016392115340970 ) ) ;
#8124=VECTOR ( 'NONE', #20246, 1000.000000000000000 ) ;
#8130=CARTESIAN_POINT ( 'NONE',  ( -46.76215110878947456, 31.00000000000000355, 53.15211786535368788 ) ) ;
#8140=CARTESIAN_POINT ( 'NONE',  ( 97.09201668843398636, 39.99999999999999289, 6.474068422258194566 ) ) ;
#8142=CARTESIAN_POINT ( 'NONE',  ( -3.169834189307652927, 31.00000000000000355, -24.13593742708953016 ) ) ;
#8152=CARTESIAN_POINT ( 'NONE',  ( 89.65113856817994531, 31.00000000000000000, -30.44896562292877462 ) ) ;
#8159=CARTESIAN_POINT ( 'NONE',  ( -15.23573235977941032, 40.00000000000000000, 26.30445775087293114 ) ) ;
#8186=CARTESIAN_POINT ( 'NONE',  ( 30.22238470471967631, 31.00000000000000355, -34.33595424619392844 ) ) ;
#8196=CARTESIAN_POINT ( 'NONE',  ( -16.51797447735934199, 40.00000000000000000, -62.05742538352703974 ) ) ;
#8210=CARTESIAN_POINT ( 'NONE',  ( -9.469526743414824921, 31.00000000000000355, -71.82433816204535049 ) ) ;
#8221=CARTESIAN_POINT ( 'NONE',  ( -40.35386350238496789, 31.00000000000000355, 69.65762217234957632 ) ) ;
#8222=CARTESIAN_POINT ( 'NONE',  ( 39.23423008407738877, 40.00000000000000000, 79.83814995801118641 ) ) ;
#8236=CARTESIAN_POINT ( 'NONE',  ( 95.10416666600561086, 39.99999999999999289, 6.217735451873073416 ) ) ;
#8249=CARTESIAN_POINT ( 'NONE',  ( -30.84436395684957333, 40.00000000000000000, -10.52363363425145337 ) ) ;
#8262=CARTESIAN_POINT ( 'NONE',  ( -30.01493782828161017, 31.00000000000000355, -3.947526014606304035 ) ) ;
#8270=CARTESIAN_POINT ( 'NONE',  ( 75.10416666583130052, 31.00000000000000000, 4.908738512847474311 ) ) ;
#8272=CARTESIAN_POINT ( 'NONE',  ( -33.53193138075044999, 31.00000000000000355, 38.09769221459629307 ) ) ;
#8273=CARTESIAN_POINT ( 'NONE',  ( -87.52616871875942195, 40.00000000000000711, -23.43677886868077209 ) ) ;
#8286=CARTESIAN_POINT ( 'NONE',  ( 42.05404839982585941, 40.00000000000000000, -47.95475229022623864 ) ) ;
#8309=VECTOR ( 'NONE', #468, 1000.000000000000000 ) ;
#8312=CARTESIAN_POINT ( 'NONE',  ( -21.36651465564686703, 31.00000000000000355, 43.35257367405362317 ) ) ;
#8318=CARTESIAN_POINT ( 'NONE',  ( 4.090615425948669781, 40.00000000000000000, -62.60416666561555132 ) ) ;
#8319=CARTESIAN_POINT ( 'NONE',  ( 18.91139405008128804, 40.00000000000000000, 55.99505798892768382 ) ) ;
#8325=CARTESIAN_POINT ( 'NONE',  ( -7.088330391075835735, 31.00000000000000355, -20.85399598300688595 ) ) ;
#8328=CARTESIAN_POINT ( 'NONE',  ( -30.01493782828161017, 40.00000000000000000, -3.947526014606304035 ) ) ;
#8343=CARTESIAN_POINT ( 'NONE',  ( -68.78002826185903018, 31.00000000000000711, -23.46745878763085358 ) ) ;
#8350=CARTESIAN_POINT ( 'NONE',  ( 6.386360208629404234, 40.00000000000000000, 99.40013590833049761 ) ) ;
#8351=CARTESIAN_POINT ( 'NONE',  ( 17.33436897218374639, 31.00000000000000355, 22.64673195036552755 ) ) ;
#8363=CARTESIAN_POINT ( 'NONE',  ( -99.14707074559267141, 31.00000000000000711, 13.06922382031732610 ) ) ;
#8367=CARTESIAN_POINT ( 'NONE',  ( -3.925388345520635536, 40.00000000000000000, 29.51202942214662173 ) ) ;
#8382=DIRECTION ( 'NONE',  ( 0.000000000000000000, 1.541976423090494844E-15, 1.000000000000000000 ) ) ;
#8392=ORIENTED_EDGE ( 'NONE', *, *, #6812, .T. ) ;
#8394=CARTESIAN_POINT ( 'NONE',  ( 46.89968353241609833, 31.00000000000000355, -2.988513402017745513 ) ) ;
#8399=DIRECTION ( 'NONE',  ( 0.000000000000000000, 1.000000000000000000, 0.000000000000000000 ) ) ;
#8403=CARTESIAN_POINT ( 'NONE',  ( -7.911223860816524400, 40.00000000000000000, 59.30865348673674475 ) ) ;
#8413=CARTESIAN_POINT ( 'NONE',  ( -43.59452257625678584, 31.00000000000000355, -56.81327804312699925 ) ) ;
#8426=CARTESIAN_POINT ( 'NONE',  ( -41.82916961767931951, 31.00000000000000355, -72.66191475361131324 ) ) ;
#8427=CARTESIAN_POINT ( 'NONE',  ( -50.81742119984753714, 40.00000000000000000, -66.42451308377114572 ) ) ;
#8456=CARTESIAN_POINT ( 'NONE',  ( 1.888402776346428613, 40.00000000000000000, 29.39821258742166776 ) ) ;
#8467=CARTESIAN_POINT ( 'NONE',  ( -23.50435451693408950, 31.00000000000000355, 30.64856077952424940 ) ) ;
#8472=CARTESIAN_POINT ( 'NONE',  ( 60.46509673945340779, 31.00000000000000000, 46.37897171330492085 ) ) ;
#8475=CARTESIAN_POINT ( 'NONE',  ( -25.29816761085220378, 31.00000000000000355, 43.63644233510515846 ) ) ;
#8476=CARTESIAN_POINT ( 'NONE',  ( 11.43299787627070607, 40.00000000000000000, 86.72764684403134083 ) ) ;
#8489=CARTESIAN_POINT ( 'NONE',  ( 8.815036365794538753, 40.00000000000000000, 66.85656860134390911 ) ) ;
#8521=CARTESIAN_POINT ( 'NONE',  ( -47.94314659152439617, 31.00000000000000355, -16.27230485535717719 ) ) ;
#8525=DIRECTION ( 'NONE',  ( 0.9470131699890049770, 1.701542661702850483E-16, 0.3211947320043963550 ) ) ;
#8527=CARTESIAN_POINT ( 'NONE',  ( -44.33513214241411760, 40.00000000000000000, 38.89722855811361768 ) ) ;
#8534=CARTESIAN_POINT ( 'NONE',  ( -10.31048697494744815, 40.00000000000000000, -30.34325702988586215 ) ) ;
#8550=CARTESIAN_POINT ( 'NONE',  ( -79.00001692110807028, 31.00000000000000711, 21.04436337235335230 ) ) ;
#8557=CARTESIAN_POINT ( 'NONE',  ( -91.07534658258109062, 40.00000000000000711, 44.76935032130646874 ) ) ;
#8558=CARTESIAN_POINT ( 'NONE',  ( -21.70016380022026681, 31.00000000000000355, -5.809120511592387182 ) ) ;
#8570=CARTESIAN_POINT ( 'NONE',  ( 70.70367055548476287, 31.00000000000000000, -62.02616482874480397 ) ) ;
#8573=CARTESIAN_POINT ( 'NONE',  ( -26.91141215548883991, 40.00000000000000000, 30.57553017915055449 ) ) ;
#8574=EDGE_CURVE ( 'NONE', #41039, #20422, #7768, .T. ) ;
#8599=CARTESIAN_POINT ( 'NONE',  ( 42.13926417418816328, 31.00000000000000355, -36.83769365847010846 ) ) ;
#8606=CARTESIAN_POINT ( 'NONE',  ( -4.660665814384791439, 40.00000000000000000, 69.59371722953135020 ) ) ;
#8614=VECTOR ( 'NONE', #14049, 1000.000000000000000 ) ;
#8620=CARTESIAN_POINT ( 'NONE',  ( -69.34045338167970840, 31.00000000000000711, 9.142281554609933636 ) ) ;
#8631=CARTESIAN_POINT ( 'NONE',  ( -78.26717753304431824, 31.00000000000000711, -26.69481836928899554 ) ) ;
#8632=CARTESIAN_POINT ( 'NONE',  ( -45.36921519482122989, 40.00000000000000711, 78.33339762292068542 ) ) ;
#8653=CARTESIAN_POINT ( 'NONE',  ( -1.587008504153756938, 31.00000000000000355, -24.39691638390477380 ) ) ;
#8664=CARTESIAN_POINT ( 'NONE',  ( -30.82418422902937039, 40.00000000000000000, 26.94311707097686792 ) ) ;
#8675=CARTESIAN_POINT ( 'NONE',  ( 33.47591237148697729, 31.00000000000000355, -8.973542178613062248 ) ) ;
#8681=CARTESIAN_POINT ( 'NONE',  ( -72.56464488860213180, 31.00000000000000711, -35.76892886290303863 ) ) ;
#8685=CARTESIAN_POINT ( 'NONE',  ( -47.35250803175854628, 31.00000000000000355, -23.44639516808300073 ) ) ;
#8689=CARTESIAN_POINT ( 'NONE',  ( 12.12865573427490062, 40.00000000000000000, -92.11205733446308841 ) ) ;
#8701=CARTESIAN_POINT ( 'NONE',  ( -69.89583333424914713, 40.00000000000000711, 4.581489278091138040 ) ) ;
#8721=ORIENTED_EDGE ( 'NONE', *, *, #40675, .T. ) ;
#8731=CARTESIAN_POINT ( 'NONE',  ( 12.21457428495364006, 31.00000000000000355, 45.57612047952555656 ) ) ;
#8735=EDGE_CURVE ( 'NONE', #16446, #1738, #9876, .T. ) ;
#8741=CARTESIAN_POINT ( 'NONE',  ( -59.89583333444493718, 40.00000000000000711, 3.926990808566372060 ) ) ;
#8754=CARTESIAN_POINT ( 'NONE',  ( 34.28525303991722240, 40.00000000000000000, 9.176237600273646322 ) ) ;
#8765=CARTESIAN_POINT ( 'NONE',  ( 27.50146173783093317, 31.00000000000000355, -80.63904244945182143 ) ) ;
#8774=CARTESIAN_POINT ( 'NONE',  ( -76.05825820879898913, 40.00000000000000711, 66.55365856249082412 ) ) ;
#8776=CARTESIAN_POINT ( 'NONE',  ( -9.709369018688816411, 31.00000000000000355, 28.47525938324675820 ) ) ;
#8789=CARTESIAN_POINT ( 'NONE',  ( 57.05379307149791401, 31.00000000000000000, -74.37948018729004218 ) ) ;
#8794=CARTESIAN_POINT ( 'NONE',  ( 24.21999397792122366, 40.00000000000000000, 8.216913396989165008 ) ) ;
#8795=CARTESIAN_POINT ( 'NONE',  ( -24.93870012979089168, 40.00000000000000000, -21.94074674037796058 ) ) ;
#8824=CARTESIAN_POINT ( 'NONE',  ( 29.31577600746836154, 31.00000000000000355, 50.95836110721448620 ) ) ;
#8825=ORIENTED_EDGE ( 'NONE', *, *, #30741, .T. ) ;
#8831=CARTESIAN_POINT ( 'NONE',  ( 4.991138515316659863, 40.00000000000000000, -74.59332054773635434 ) ) ;
#8844=CARTESIAN_POINT ( 'NONE',  ( 64.78932475141161262, 31.00000000000000000, 8.528958657501300777 ) ) ;
#8857=CARTESIAN_POINT ( 'NONE',  ( -88.68107738130200346, 31.00000000000000711, 23.63280646692842524 ) ) ;
#8858=CARTESIAN_POINT ( 'NONE',  ( 64.90225467577229779, 39.99999999999999289, 74.17428024387139374 ) ) ;
#8873=AXIS2_PLACEMENT_3D ( 'NONE', #19246, #42322, #25788 ) ;
#8880=CARTESIAN_POINT ( 'NONE',  ( 22.27703560431448793, 31.00000000000000355, 17.12883495622356023 ) ) ;
#8891=CARTESIAN_POINT ( 'NONE',  ( -41.89947471387619515, 40.00000000000000000, 2.670153906482984230 ) ) ;
#8901=CARTESIAN_POINT ( 'NONE',  ( 29.64712525329720449, 31.00000000000000355, -17.12831674356021239 ) ) ;
#8903=CARTESIAN_POINT ( 'NONE',  ( -99.91857577502598531, 31.00000000000000355, -1.280628618496984616 ) ) ;
#8909=CARTESIAN_POINT ( 'NONE',  ( 85.10416666585589951, 31.00000000000000000, 5.563236982362346872 ) ) ;
#8915=CARTESIAN_POINT ( 'NONE',  ( 54.55067978551168295, 31.00000000000000355, 18.62288743479739139 ) ) ;
#8916=CARTESIAN_POINT ( 'NONE',  ( 74.70319961851696178, 39.99999999999999289, -57.31929289364909152 ) ) ;
#8922=DIRECTION ( 'NONE',  ( 0.000000000000000000, 0.000000000000000000, -1.000000000000000000 ) ) ;
#8929=CARTESIAN_POINT ( 'NONE',  ( -61.47519263390311295, 40.00000000000000711, -35.49250405581909007 ) ) ;
#8957=CARTESIAN_POINT ( 'NONE',  ( 38.75409931461306456, 31.00000000000000355, -50.52625141960567134 ) ) ;
#8963=CARTESIAN_POINT ( 'NONE',  ( -37.49462465745612860, 40.00000000000000000, -48.86220178749748300 ) ) ;
#8967=FACE_OUTER_BOUND ( 'NONE', #23309, .T. ) ;
#8972=CARTESIAN_POINT ( 'NONE',  ( 18.38119342899891961, 40.00000000000000000, 31.81670425098764099 ) ) ;
#8984=CARTESIAN_POINT ( 'NONE',  ( -49.21613380539480431, 31.00000000000000355, 63.96793098899347996 ) ) ;
#8997=CARTESIAN_POINT ( 'NONE',  ( -96.33078216555149709, 40.00000000000000711, 32.58251675340183340 ) ) ;
#9008=CARTESIAN_POINT ( 'NONE',  ( 20.45440555730427690, 40.00000000000000000, -26.67302265141799467 ) ) ;
#9009=CARTESIAN_POINT ( 'NONE',  ( -20.27214883179920690, 40.00000000000000000, 34.96734655410256210 ) ) ;
#9028=CARTESIAN_POINT ( 'NONE',  ( -60.10374203099167545, 40.00000000000000711, 78.35501831527777483 ) ) ;
#9030=DIRECTION ( 'NONE',  ( 0.000000000000000000, 0.000000000000000000, 1.000000000000000000 ) ) ;
#9034=CARTESIAN_POINT ( 'NONE',  ( 25.95756378415329024, 31.00000000000000355, 52.86556711865710412 ) ) ;
#9042=CARTESIAN_POINT ( 'NONE',  ( 68.60033760563641181, 39.99999999999999289, -33.70054013428169526 ) ) ;
#9056=CARTESIAN_POINT ( 'NONE',  ( 43.85342918759069164, 31.00000000000000355, 49.98553323097543455 ) ) ;
#9064=CARTESIAN_POINT ( 'NONE',  ( 31.77777543000702565, 31.00000000000000355, 93.95825142778512884 ) ) ;
#9065=CARTESIAN_POINT ( 'NONE',  ( 96.17895579825814423, 39.99999999999999289, -12.55124642863780338 ) ) ;
#9090=CARTESIAN_POINT ( 'NONE',  ( 46.89968353242633015, 40.00000000000000000, -2.988513402017745069 ) ) ;
#9107=CARTESIAN_POINT ( 'NONE',  ( 26.99674208481366833, 31.00000000000000355, -20.71990538090019029 ) ) ;
#9113=CARTESIAN_POINT ( 'NONE',  ( -60.37409795221152109, 31.00000000000000711, -68.82020352599361956 ) ) ;
#9116=CARTESIAN_POINT ( 'NONE',  ( 64.03668805592332092, 31.00000000000000000, 21.85318084035846198 ) ) ;
#9117=CARTESIAN_POINT ( 'NONE',  ( 28.99662776679782539, 40.00000000000000000, -58.58186007941694129 ) ) ;
#9118=CARTESIAN_POINT ( 'NONE',  ( -96.39699453480135105, 40.00000000000000711, 25.82690913164849889 ) ) ;
#9131=CARTESIAN_POINT ( 'NONE',  ( -20.19574676229028043, 40.00000000000000000, 75.42596061005518493 ) ) ;
#9140=ORIENTED_EDGE ( 'NONE', *, *, #31412, .F. ) ;
#9142=ORIENTED_EDGE ( 'NONE', *, *, #38506, .T. ) ;
#9148=ORIENTED_EDGE ( 'NONE', *, *, #26266, .T. ) ;
#9160=CARTESIAN_POINT ( 'NONE',  ( -30.90996028308246224, 31.00000000000000355, -53.51249422725337013 ) ) ;
#9166=CARTESIAN_POINT ( 'NONE',  ( 12.49611804805956261, 31.00000000000000355, 37.00809541493615029 ) ) ;
#9168=CARTESIAN_POINT ( 'NONE',  ( -53.60515337853228601, 40.00000000000000000, -47.01024902908782366 ) ) ;
#9178=CARTESIAN_POINT ( 'NONE',  ( 19.15075862373047144, 40.00000000000000000, -38.85840887180553693 ) ) ;
#9181=VERTEX_POINT ( 'NONE', #38169 ) ;
#9192=CARTESIAN_POINT ( 'NONE',  ( 69.92891852055319646, 31.00000000000000000, 53.79372986807582180 ) ) ;
#9209=CARTESIAN_POINT ( 'NONE',  ( 17.42035916340572399, 31.00000000000000355, 19.85006075799527991 ) ) ;
#9214=CARTESIAN_POINT ( 'NONE',  ( -31.00354902519490352, 40.00000000000000000, -27.18544651223506392 ) ) ;
#9215=CARTESIAN_POINT ( 'NONE',  ( 34.63398384099732397, 40.00000000000000000, -11.69655689657770559 ) ) ;
#9226=CIRCLE ( 'NONE', #34330, 4.500000000000002665 ) ;
#9240=CARTESIAN_POINT ( 'NONE',  ( 58.84426737335365232, 40.00000000000000000, 76.69096868241209108 ) ) ;
#9244=CARTESIAN_POINT ( 'NONE',  ( -16.80298683001097260, 17.11489954122026447, 2.367532924972517439 ) ) ;
#9246=CARTESIAN_POINT ( 'NONE',  ( -3.469229457552013507, 31.00000000000000355, -54.39987425099493379 ) ) ;
#9252=CARTESIAN_POINT ( 'NONE',  ( -46.76215110880508519, 40.00000000000000000, 53.15211786533807725 ) ) ;
#9263=DIRECTION ( 'NONE',  ( -0.2604563316218754254, -1.023593278765030694E-15, -0.9654856287475623855 ) ) ;
#9264=CARTESIAN_POINT ( 'NONE',  ( -47.90394619311608437, 31.00000000000000355, 62.45286580340285099 ) ) ;
#9266=LINE ( 'NONE', #25885, #28361 ) ;
#9273=CARTESIAN_POINT ( 'NONE',  ( -6.638544827991894159, 31.00000000000000355, 99.59190654106262741 ) ) ;
#9274=CARTESIAN_POINT ( 'NONE',  ( 58.37089435906660384, 39.99999999999999289, -75.89027429297954086 ) ) ;
#9301=CARTESIAN_POINT ( 'NONE',  ( 10.06970066534629815, 40.00000000000000000, 37.84957806120350199 ) ) ;
#9313=CARTESIAN_POINT ( 'NONE',  ( 22.22924588317381023, 31.00000000000000355, -25.35314793696836588 ) ) ;
#9317=CARTESIAN_POINT ( 'NONE',  ( 81.71702119589899382, 31.00000000000000000, -47.19735719316410183 ) ) ;
#9321=CARTESIAN_POINT ( 'NONE',  ( -45.90931453311223720, 31.00000000000000355, 40.13788153756826915 ) ) ;
#9322=CARTESIAN_POINT ( 'NONE',  ( -50.06114249711410480, 40.00000000000000000, -38.53249520213266521 ) ) ;
#9339=CARTESIAN_POINT ( 'NONE',  ( 4.745113895470035814, 40.00000000000000000, -72.60416666572081112 ) ) ;
#9348=CARTESIAN_POINT ( 'NONE',  ( -22.00000000000000000, 31.00000000000000355, 0.000000000000000000 ) ) ;
#9368=CARTESIAN_POINT ( 'NONE',  ( 37.24516168167158270, 31.00000000000000355, 42.45166511289891531 ) ) ;
#9371=CARTESIAN_POINT ( 'NONE',  ( 17.75583184595726749, 31.00000000000000355, -30.63479189996604646 ) ) ;
#9373=CARTESIAN_POINT ( 'NONE',  ( 23.52215716829092074, 40.00000000000000000, -69.29398394448777765 ) ) ;
#9384=CARTESIAN_POINT ( 'NONE',  ( 34.94781834021004840, 40.00000000000000000, -26.81980329959834108 ) ) ;
#9395=ORIENTED_EDGE ( 'NONE', *, *, #8574, .T. ) ;
#9399=CARTESIAN_POINT ( 'NONE',  ( 76.36627019853398224, 31.00000000000000000, -58.43797548692494814 ) ) ;
#9402=DIRECTION ( 'NONE',  ( 0.000000000000000000, 1.000000000000000000, 0.000000000000000000 ) ) ;
#9419=CARTESIAN_POINT ( 'NONE',  ( -21.73352778766994575, 31.00000000000000355, 19.07242603999910457 ) ) ;
#9428=CARTESIAN_POINT ( 'NONE',  ( -12.24460912605626106, 40.00000000000000000, 36.08157028455360660 ) ) ;
#9430=CARTESIAN_POINT ( 'NONE',  ( -10.89792128226954482, 40.00000000000000000, -32.25956908328721795 ) ) ;
#9441=CARTESIAN_POINT ( 'NONE',  ( -15.99999999999997691, 40.00000000000000711, 4.500000000000005329 ) ) ;
#9450=EDGE_CURVE ( 'NONE', #1738, #39440, #9226, .T. ) ;
#9461=CARTESIAN_POINT ( 'NONE',  ( 54.79583221319987985, 31.00000000000000355, -14.58025558542526490 ) ) ;
#9471=CARTESIAN_POINT ( 'NONE',  ( -55.03444096782886419, 40.00000000000000000, -48.41538206857744342 ) ) ;
#9481=LINE ( 'NONE', #5569, #2984 ) ;
#9482=CARTESIAN_POINT ( 'NONE',  ( -100.0589655806010967, 40.00000000000002132, 21.59728106529621883 ) ) ;
#9483=CARTESIAN_POINT ( 'NONE',  ( 66.75446398494719347, 31.00000000000000000, -32.91950810868348043 ) ) ;
#9496=CARTESIAN_POINT ( 'NONE',  ( 96.56285295106283684, 31.00000000000000000, 12.84127866191736977 ) ) ;
#9498=CARTESIAN_POINT ( 'NONE',  ( -73.90312034494817794, 40.00000000000000711, -56.84521418463217657 ) ) ;
#9528=CARTESIAN_POINT ( 'NONE',  ( -24.78443185004241656, 40.00000000000000000, 32.19086620116434005 ) ) ;
#9536=EDGE_CURVE ( 'NONE', #1383, #39440, #37678, .T. ) ;
#9545=CARTESIAN_POINT ( 'NONE',  ( 23.39270017067629936, 31.00000000000000355, 40.49502024156475244 ) ) ;
#9550=CARTESIAN_POINT ( 'NONE',  ( -6.054110834496889026, 31.00000000000000355, -92.39583333400220511 ) ) ;
#9554=CARTESIAN_POINT ( 'NONE',  ( 52.50410707182467718, 31.00000000000000000, -40.15145572480454916 ) ) ;
#9555=CARTESIAN_POINT ( 'NONE',  ( -31.81746463534672387, 40.00000000000000000, -55.29958784370776925 ) ) ;
#9570=CARTESIAN_POINT ( 'NONE',  ( 46.64447153568531945, 40.00000000000000000, 60.78881617101084345 ) ) ;
#9601=CARTESIAN_POINT ( 'NONE',  ( -56.43872490705654599, 31.00000000000000711, 19.17141758013517716 ) ) ;
#9605=CARTESIAN_POINT ( 'NONE',  ( -15.23573235977617379, 31.00000000000000355, 26.30445775087292404 ) ) ;
#9606=CARTESIAN_POINT ( 'NONE',  ( -45.35818215263140019, 40.00000000000000000, 51.72168634911185592 ) ) ;
#9616=CARTESIAN_POINT ( 'NONE',  ( 39.77940265867437120, 40.00000000000000000, 22.96373720238702276 ) ) ;
#9630=CARTESIAN_POINT ( 'NONE',  ( -59.98614492175870794, 31.00000000000000711, 68.21249229744711329 ) ) ;
#9648=CARTESIAN_POINT ( 'NONE',  ( 2.127120017302678523, 31.00000000000000355, -32.60416666460785962 ) ) ;
#9650=ORIENTED_EDGE ( 'NONE', *, *, #19399, .T. ) ;
#9652=ADVANCED_FACE ( 'NONE', ( #25286 ), #4746, .F. ) ;
#9656=CARTESIAN_POINT ( 'NONE',  ( 34.89583333524210218, 40.00000000000000000, -2.290744634698907767 ) ) ;
#9657=CARTESIAN_POINT ( 'NONE',  ( 21.53706125533296500, 40.00000000000000000, 43.87245753945351368 ) ) ;
#9684=CARTESIAN_POINT ( 'NONE',  ( -3.998040010416403334, 31.00000000000000355, 59.59469406578620720 ) ) ;
#9691=CARTESIAN_POINT ( 'NONE',  ( -20.82795069772234342, 40.00000000000000000, 77.32795358076222669 ) ) ;
#9701=CARTESIAN_POINT ( 'NONE',  ( -80.10416666582359824, 31.00000000000000711, -5.235987747607834031 ) ) ;
#9713=CARTESIAN_POINT ( 'NONE',  ( 49.34100556531812742, 31.00000000000000355, 85.68208892729249726 ) ) ;
#9714=CARTESIAN_POINT ( 'NONE',  ( 73.86091552542920624, 39.99999999999999289, 64.94433634442138725 ) ) ;
#9731=CARTESIAN_POINT ( 'NONE',  ( 17.75583184595726749, 31.00000000000000355, -30.63479189996604646 ) ) ;
#9739=CARTESIAN_POINT ( 'NONE',  ( -52.09564885855072447, 40.00000000000000000, -3.498939618562995513 ) ) ;
#9750=CARTESIAN_POINT ( 'NONE',  ( -50.10416666532988472, 31.00000000000000355, -3.272492339034341224 ) ) ;
#9754=CARTESIAN_POINT ( 'NONE',  ( 43.43872713698582544, 31.00000000000000355, 75.20828420317944563 ) ) ;
#9759=CARTESIAN_POINT ( 'NONE',  ( -58.36801134197498442, 31.00000000000000711, 19.71467013092928866 ) ) ;
#9760=CARTESIAN_POINT ( 'NONE',  ( -61.79211991639481028, 40.00000000000000711, -8.240724169186190551 ) ) ;
#9761=CARTESIAN_POINT ( 'NONE',  ( 6.381360069253262601, 40.00000000000000000, 97.39583333395333398 ) ) ;
#9775=CARTESIAN_POINT ( 'NONE',  ( 57.37208743749949491, 40.00000000000000000, 50.31438278193533620 ) ) ;
#9777=ORIENTED_EDGE ( 'NONE', *, *, #16267, .F. ) ;
#9797=CARTESIAN_POINT ( 'NONE',  ( -15.93581279029885422, 31.00000000000000355, -13.96891150189262021 ) ) ;
#9803=CARTESIAN_POINT ( 'NONE',  ( 18.36587843422771016, 31.00000000000000355, 54.06640964556338957 ) ) ;
#9806=CARTESIAN_POINT ( 'NONE',  ( -26.24023198663968515, 31.00000000000000355, -20.19409642360271917 ) ) ;
#9807=CARTESIAN_POINT ( 'NONE',  ( -69.34045338167970840, 40.00000000000000711, 9.142281554609933636 ) ) ;
#9819=CARTESIAN_POINT ( 'NONE',  ( -38.92335646797288717, 40.00000000000000000, 29.86975225897632313 ) ) ;
#9832=EDGE_CURVE ( 'NONE', #7063, #15282, #37412, .T. ) ;
#9833=CARTESIAN_POINT ( 'NONE',  ( -11.85673204380701939, 31.00000000000000355, 89.11174773313419450 ) ) ;
#9849=CARTESIAN_POINT ( 'NONE',  ( -30.01493782828161017, 31.00000000000000355, -3.947526014606304035 ) ) ;
#9855=DIRECTION ( 'NONE',  ( 0.000000000000000000, 1.000000000000000000, 0.000000000000000000 ) ) ;
#9856=CARTESIAN_POINT ( 'NONE',  ( 34.98270738856093232, 40.00000000000000000, 4.602016392115340970 ) ) ;
#9857=CARTESIAN_POINT ( 'NONE',  ( -44.44570800418432555, 40.00000000000000000, 25.56477902013099524 ) ) ;
#9869=ORIENTED_EDGE ( 'NONE', *, *, #30853, .T. ) ;
#9876=CIRCLE ( 'NONE', #42594, 4.500000000000002665 ) ;
#9887=CARTESIAN_POINT ( 'NONE',  ( -60.39136959358631174, 31.00000000000000711, -16.27924862579292054 ) ) ;
#9894=CARTESIAN_POINT ( 'NONE',  ( -40.35386350238497499, 40.00000000000000000, 69.65762217234959053 ) ) ;
#9905=CARTESIAN_POINT ( 'NONE',  ( -70.15350862410126354, 31.00000000000000711, -40.50401079722123399 ) ) ;
#9933=EDGE_LOOP ( 'NONE', ( #3866, #32045, #8042, #9777 ) ) ;
#9935=CARTESIAN_POINT ( 'NONE',  ( -32.09999204393464822, 31.00000000000000355, -2.147948991655045159 ) ) ;
#9944=CARTESIAN_POINT ( 'NONE',  ( 3.665567271000699012, 40.00000000000000000, -54.59530427606813419 ) ) ;
#9954=CARTESIAN_POINT ( 'NONE',  ( 43.19851606872948935, 31.00000000000000355, 14.66122656362567689 ) ) ;
#9961=CARTESIAN_POINT ( 'NONE',  ( -10.86393331615775892, 40.00000000000000000, -18.79923026442779843 ) ) ;
#9965=CARTESIAN_POINT ( 'NONE',  ( -37.00582609755892349, 31.00000000000000355, 48.07482304779467341 ) ) ;
#9966=CARTESIAN_POINT ( 'NONE',  ( 66.37122006405570573, 39.99999999999999289, -8.639838683448301637 ) ) ;
#9978=DIRECTION ( 'NONE',  ( 0.000000000000000000, -1.000000000000000000, 5.297542245118643184E-16 ) ) ;
#9982=CARTESIAN_POINT ( 'NONE',  ( 5.726861599741335240, 40.00000000000000000, 87.39583333411552246 ) ) ;
#9994=VERTEX_POINT ( 'NONE', #40893 ) ;
#9997=FACE_OUTER_BOUND ( 'NONE', #29660, .T. ) ;
#10015=CARTESIAN_POINT ( 'NONE',  ( -43.59452257625678584, 31.00000000000000355, -56.81327804312699925 ) ) ;
#10018=CARTESIAN_POINT ( 'NONE',  ( -32.09999204393464822, 31.00000000000000355, -2.147948991655045159 ) ) ;
#10020=CARTESIAN_POINT ( 'NONE',  ( -61.47519263390311295, 40.00000000000000711, -35.49250405581909007 ) ) ;
#10029=CARTESIAN_POINT ( 'NONE',  ( 41.10549127292548377, 40.00000000000000000, 20.25863663968860706 ) ) ;
#10035=CARTESIAN_POINT ( 'NONE',  ( -105.9879088449591933, 31.00000000000000355, -0.3807199291576673361 ) ) ;
#10045=CARTESIAN_POINT ( 'NONE',  ( 30.72743980831337751, 31.00000000000000355, -90.12673907452091271 ) ) ;
#10065=CARTESIAN_POINT ( 'NONE',  ( 10.63353083439206870, 31.00000000000000355, -31.33693976183458219 ) ) ;
#10071=CARTESIAN_POINT ( 'NONE',  ( -20.88694679984194380, 40.00000000000000000, -36.15586224631631751 ) ) ;
#10073=CARTESIAN_POINT ( 'NONE',  ( -32.45554871466747215, 40.00000000000000000, -28.56710966684967090 ) ) ;
#10097=CARTESIAN_POINT ( 'NONE',  ( 64.47787635702036368, 31.00000000000000000, -17.16423577041365789 ) ) ;
#10104=CARTESIAN_POINT ( 'NONE',  ( 86.24314314301659579, 39.99999999999999289, -11.24622374122959201 ) ) ;
#10113=CARTESIAN_POINT ( 'NONE',  ( -15.99999999999997691, 40.00000000000000000, 5.571627607371296764E-15 ) ) ;
#10114=VERTEX_POINT ( 'NONE', #35220 ) ;
#10118=CARTESIAN_POINT ( 'NONE',  ( 46.64447153568531945, 31.00000000000000355, 60.78881617101084345 ) ) ;
#10134=ORIENTED_EDGE ( 'NONE', *, *, #5750, .F. ) ;
#10150=CARTESIAN_POINT ( 'NONE',  ( -31.89861325429239258, 31.00000000000000355, 2.042328591206914012 ) ) ;
#10156=CARTESIAN_POINT ( 'NONE',  ( -105.9879088449591933, 40.00000000000000000, -0.3807199291576673361 ) ) ;
#10157=CARTESIAN_POINT ( 'NONE',  ( -16.19793102918200134, 40.00000000000000000, 47.43702525406639836 ) ) ;
#10171=CARTESIAN_POINT ( 'NONE',  ( 34.77048308403384169, 31.00000000000000355, 30.48958026498159768 ) ) ;
#10181=CARTESIAN_POINT ( 'NONE',  ( 25.17870271038170316, 31.00000000000000355, 93.97695291299892517 ) ) ;
#10185=CARTESIAN_POINT ( 'NONE',  ( -61.81085491475939619, 31.00000000000000711, 35.57109242551294415 ) ) ;
#10186=CARTESIAN_POINT ( 'NONE',  ( -71.72626536479072001, 40.00000000000000711, -9.557116936239163252 ) ) ;
#10195=VERTEX_POINT ( 'NONE', #42404 ) ;
#10202=CARTESIAN_POINT ( 'NONE',  ( 85.10416666585589951, 39.99999999999999289, 5.563236982362346872 ) ) ;
#10213=DIRECTION ( 'NONE',  ( 1.000000000000000000, 0.000000000000000000, 0.000000000000000000 ) ) ;
#10217=CARTESIAN_POINT ( 'NONE',  ( 8.075107282079295956, 40.00000000000000000, -23.73893940452291318 ) ) ;
#10220=FACE_OUTER_BOUND ( 'NONE', #42871, .T. ) ;
#10227=( NAMED_UNIT ( * ) SI_UNIT ( $, .STERADIAN. ) SOLID_ANGLE_UNIT ( ) );
#10238=CARTESIAN_POINT ( 'NONE',  ( -4.417864660710832503, 31.00000000000000355, 67.60416666563759236 ) ) ;
#10242=CARTESIAN_POINT ( 'NONE',  ( 47.09643503919448193, 31.00000000000000355, 3.164684800459845349 ) ) ;
#10244=CARTESIAN_POINT ( 'NONE',  ( 73.00591898829820536, 39.99999999999999289, 19.54754034098114701 ) ) ;
#10254=CARTESIAN_POINT ( 'NONE',  ( -29.22812062908682051, 40.00000000000000000, 50.62729764625685647 ) ) ;
#10272=CARTESIAN_POINT ( 'NONE',  ( -41.44813913998980581, 31.00000000000000355, -84.33308812960441969 ) ) ;
#10291=CARTESIAN_POINT ( 'NONE',  ( -39.95047694894377344, 31.00000000000000355, -5.256506769647570465 ) ) ;
#10299=CARTESIAN_POINT ( 'NONE',  ( -40.58740609958903889, 40.00000000000000000, -31.12922691583434798 ) ) ;
#10301=CARTESIAN_POINT ( 'NONE',  ( -14.09736097164574709, 40.00000000000000000, -41.75563764761122343 ) ) ;
#10310=CARTESIAN_POINT ( 'NONE',  ( 20.70971545910534672, 40.00000000000000000, 15.87948211774388518 ) ) ;
#10320=EDGE_CURVE ( 'NONE', #7063, #33075, #19973, .T. ) ;
#10329=CARTESIAN_POINT ( 'NONE',  ( -41.78821403078461572, 31.00000000000000355, -47.79414628086201589 ) ) ;
#10339=CARTESIAN_POINT ( 'NONE',  ( 58.29702017945731995, 39.99999999999999289, 66.63806913872475945 ) ) ;
#10351=CARTESIAN_POINT ( 'NONE',  ( 6.054110834496887250, 31.00000000000000355, -92.60416666599778068 ) ) ;
#10380=CARTESIAN_POINT ( 'NONE',  ( 4.597210615069569961, 31.00000000000000355, -34.47704375836577384 ) ) ;
#10388=CARTESIAN_POINT ( 'NONE',  ( 50.14038141241296387, 40.00000000000000000, 29.06424286984033145 ) ) ;
#10392=DIRECTION ( 'NONE',  ( 0.9247238835424299586, 4.035472873002398249E-16, 0.3806385939525924744 ) ) ;
#10401=CARTESIAN_POINT ( 'NONE',  ( -16.10381281257427943, 31.00000000000000355, -60.09637020943575436 ) ) ;
#10406=CARTESIAN_POINT ( 'NONE',  ( 94.89583333399441756, 31.00000000000000000, -6.217735451874103703 ) ) ;
#10410=CARTESIAN_POINT ( 'NONE',  ( -35.65230965298280097, 31.00000000000000355, 72.05959145978816593 ) ) ;
#10411=CARTESIAN_POINT ( 'NONE',  ( -82.09281090897877675, 40.00000000000000711, -5.486092462564050365 ) ) ;
#10429=CARTESIAN_POINT ( 'NONE',  ( 84.24376206367318787, 39.99999999999999289, -11.10575268747775901 ) ) ;
#10432=LINE ( 'NONE', #36819, #33853 ) ;
#10460=CARTESIAN_POINT ( 'NONE',  ( 4.745113895470035814, 31.00000000000000355, -72.60416666572081112 ) ) ;
#10463=CARTESIAN_POINT ( 'NONE',  ( -20.27214883179046367, 31.00000000000000355, 34.96734655410254788 ) ) ;
#10464=CARTESIAN_POINT ( 'NONE',  ( -40.93297376624923345, 40.00000000000000000, -70.86912620794510076 ) ) ;
#10472=CARTESIAN_POINT ( 'NONE',  ( -57.67632858778466698, 40.00000000000000711, 15.45560639130400205 ) ) ;
#10501=LINE ( 'NONE', #6561, #18716 ) ;
#10505=CARTESIAN_POINT ( 'NONE',  ( 34.94781834021004840, 31.00000000000000355, -26.81980329959834108 ) ) ;
#10516=CARTESIAN_POINT ( 'NONE',  ( -49.88601606984090608, 40.00000000000000000, -6.565487524765669214 ) ) ;
#10517=CARTESIAN_POINT ( 'NONE',  ( 5.928665350384931365, 40.00000000000000000, -44.40877992885556580 ) ) ;
#10519=ORIENTED_EDGE ( 'NONE', *, *, #9450, .F. ) ;
#10524=CARTESIAN_POINT ( 'NONE',  ( -21.73352778766994575, 40.00000000000000000, 19.07242603999910457 ) ) ;
#10537=ORIENTED_EDGE ( 'NONE', *, *, #5889, .F. ) ;
#10541=CARTESIAN_POINT ( 'NONE',  ( -62.09442273006147417, 31.00000000000000711, -4.163950221635984938 ) ) ;
#10548=CYLINDRICAL_SURFACE ( 'NONE', #14080, 1.999999999999998668 ) ;
#10550=CARTESIAN_POINT ( 'NONE',  ( -21.69137426901471954, 40.00000000000000000, -81.42030341110599068 ) ) ;
#10563=CARTESIAN_POINT ( 'NONE',  ( -23.88228986782336349, 31.00000000000000355, -89.13686966975919290 ) ) ;
#10592=CARTESIAN_POINT ( 'NONE',  ( -27.06829236441750552, 31.00000000000000355, 15.58100167312263018 ) ) ;
#10600=CARTESIAN_POINT ( 'NONE',  ( 35.58199112951898968, 40.00000000000000000, 46.53705319855855294 ) ) ;
#10602=CARTESIAN_POINT ( 'NONE',  ( -101.1532682021072134, 31.00000000000000355, -3.256983028635321187 ) ) ;
#10612=CARTESIAN_POINT ( 'NONE',  ( 47.00375723443311671, 31.00000000000000355, -27.15133022689256137 ) ) ;
#10622=CARTESIAN_POINT ( 'NONE',  ( 63.67823170517923614, 31.00000000000000000, 72.58713758494482704 ) ) ;
#10626=CARTESIAN_POINT ( 'NONE',  ( -64.10496366466531981, 31.00000000000000711, 31.48763712508877077 ) ) ;
#10627=CARTESIAN_POINT ( 'NONE',  ( -48.39074809477736494, 40.00000000000000000, -55.33250407649475733 ) ) ;
#10643=CARTESIAN_POINT ( 'NONE',  ( 81.15556025174309696, 39.99999999999999289, 27.54985289775053658 ) ) ;
#10652=EDGE_LOOP ( 'NONE', ( #37736, #1145, #21815, #20558 ) ) ;
#10653=CARTESIAN_POINT ( 'NONE',  ( -14.30682334061562422, 40.00000000000000000, -18.65445469299709202 ) ) ;
#10663=CARTESIAN_POINT ( 'NONE',  ( -29.44516979616424024, 31.00000000000000355, -7.879824757621473275 ) ) ;
#10673=CARTESIAN_POINT ( 'NONE',  ( 9.510694223897102617, 31.00000000000000355, -72.24097909213479340 ) ) ;
#10676=CARTESIAN_POINT ( 'NONE',  ( -16.19793102917653371, 31.00000000000000355, 47.43702525407732651 ) ) ;
#10677=CARTESIAN_POINT ( 'NONE',  ( 73.03870520561201829, 39.99999999999999289, -42.18585045165268355 ) ) ;
#10689=CARTESIAN_POINT ( 'NONE',  ( 3.436116956419347002, 40.00000000000000000, -52.60416666537189911 ) ) ;
#10720=CARTESIAN_POINT ( 'NONE',  ( 33.03432996520027132, 31.00000000000000355, -28.98482729919588863 ) ) ;
#10722=DIRECTION ( 'NONE',  ( 0.000000000000000000, 1.000000000000000000, -1.060184893785364939E-15 ) ) ;
#10726=CARTESIAN_POINT ( 'NONE',  ( -31.39472673864601049, 40.00000000000000000, -40.91112553188754930 ) ) ;
#10728=CARTESIAN_POINT ( 'NONE',  ( -61.89998375879795844, 40.00000000000000711, 3.952486745199417673 ) ) ;
#10740=CARTESIAN_POINT ( 'NONE',  ( 3.579113344806025054, 40.00000000000000000, 27.11441211503905535 ) ) ;
#10759=CARTESIAN_POINT ( 'NONE',  ( 57.21690105881322097, 31.00000000000000000, -50.04162206024282966 ) ) ;
#10769=CARTESIAN_POINT ( 'NONE',  ( -87.75478321342750121, 40.00000000000000711, -29.92102470460831753 ) ) ;
#10782=CARTESIAN_POINT ( 'NONE',  ( 55.27058341129635721, 31.00000000000000000, -63.02248852588876105 ) ) ;
#10816=CARTESIAN_POINT ( 'NONE',  ( -35.75974951333986240, 31.00000000000000355, 20.56794350806610794 ) ) ;
#10826=CARTESIAN_POINT ( 'NONE',  ( -26.77709713318651552, 40.00000000000000000, 54.08981485145582724 ) ) ;
#10837=CARTESIAN_POINT ( 'NONE',  ( -54.58798567973315841, 31.00000000000000355, -26.90590473539369754 ) ) ;
#10845=CARTESIAN_POINT ( 'NONE',  ( 76.36724925129128394, 31.00000000000000000, 58.57876755120444301 ) ) ;
#10850=CARTESIAN_POINT ( 'NONE',  ( 25.34170449640226508, 31.00000000000000355, 74.97748276543396173 ) ) ;
#10852=CARTESIAN_POINT ( 'NONE',  ( -25.88810397297939403, 40.00000000000000000, 75.89534075015936310 ) ) ;
#10865=CARTESIAN_POINT ( 'NONE',  ( -61.13902149641835138, 40.00000000000000000, -53.61851653479526902 ) ) ;
#10882=CARTESIAN_POINT ( 'NONE',  ( 15.59370980024836051, 40.00000000000000000, -20.29731371384565364 ) ) ;
#10896=CARTESIAN_POINT ( 'NONE',  ( 17.96659372829068246, 31.00000000000000355, -15.76829228678407624 ) ) ;
#10902=CARTESIAN_POINT ( 'NONE',  ( 4.417864660711233959, 31.00000000000000355, 67.39583333436242185 ) ) ;
#10906=CARTESIAN_POINT ( 'NONE',  ( -30.82418422902937039, 31.00000000000000355, 26.94311707098126618 ) ) ;
#10908=CARTESIAN_POINT ( 'NONE',  ( 10.81967497908702214, 40.00000000000000000, -82.17651821321413763 ) ) ;
#10922=CARTESIAN_POINT ( 'NONE',  ( 53.64558601427197004, 40.00000000000000000, 14.36188897069615500 ) ) ;
#10934=EDGE_CURVE ( 'NONE', #5066, #15357, #18325, .T. ) ;
#10957=CARTESIAN_POINT ( 'NONE',  ( -23.50435451693408950, 31.00000000000000355, 30.64856077952424940 ) ) ;
#10958=ORIENTED_EDGE ( 'NONE', *, *, #8735, .F. ) ;
#10960=DIRECTION ( 'NONE',  ( 0.000000000000000000, 0.000000000000000000, 1.000000000000000000 ) ) ;
#10965=CARTESIAN_POINT ( 'NONE',  ( -33.94102792873697183, 40.00000000000000000, -38.68473105385043453 ) ) ;
#10966=CARTESIAN_POINT ( 'NONE',  ( -32.53655534684257589, 40.00000000000000000, -42.55839752837238166 ) ) ;
#10967=DIRECTION ( 'NONE',  ( 0.000000000000000000, -1.000000000000000000, 5.297542245118643184E-16 ) ) ;
#10974=CARTESIAN_POINT ( 'NONE',  ( 17.42035916340572399, 40.00000000000000000, 19.85006075799527991 ) ) ;
#10994=CARTESIAN_POINT ( 'NONE',  ( 34.80713033128647993, 31.00000000000000355, 70.84796410819511436 ) ) ;
#11002=CARTESIAN_POINT ( 'NONE',  ( 92.49871336443506209, 39.99999999999999289, 31.53380891771211125 ) ) ;
#11015=CARTESIAN_POINT ( 'NONE',  ( -86.71682804797315214, 31.00000000000000711, 23.23408344657299196 ) ) ;
#11019=CARTESIAN_POINT ( 'NONE',  ( -19.81637295874436333, 40.00000000000000000, -11.44243563873878777 ) ) ;
#11033=AXIS2_PLACEMENT_3D ( 'NONE', #27554, #40827, #5694 ) ;
#11048=CARTESIAN_POINT ( 'NONE',  ( 36.21668514974006570, 31.00000000000000355, 31.87730689759005287 ) ) ;
#11055=CARTESIAN_POINT ( 'NONE',  ( 25.95756378415974908, 40.00000000000000000, 52.86556711864420066 ) ) ;
#11062=( NAMED_UNIT ( * ) PLANE_ANGLE_UNIT ( ) SI_UNIT ( $, .RADIAN. ) );
#11065=CARTESIAN_POINT ( 'NONE',  ( -40.54929543462775143, 31.00000000000000355, -46.21859917192507794 ) ) ;
#11072=CARTESIAN_POINT ( 'NONE',  ( -18.92511213055653130, 40.00000000000000000, 21.58621387822740090 ) ) ;
#11078=CARTESIAN_POINT ( 'NONE',  ( 57.21690105881322097, 31.00000000000000000, -50.04162206024282966 ) ) ;
#11079=CARTESIAN_POINT ( 'NONE',  ( 37.84579180138899090, 40.00000000000000000, -65.31998993212283722 ) ) ;
#11092=CARTESIAN_POINT ( 'NONE',  ( 91.55691129138550366, 39.99999999999999289, -24.53049628908797430 ) ) ;
#11093=CARTESIAN_POINT ( 'NONE',  ( -15.99999999999997691, 31.00000000000000000, -4.499999999999995559 ) ) ;
#11105=CARTESIAN_POINT ( 'NONE',  ( -31.36635120280305955, 40.00000000000000000, -8.451140850655482595 ) ) ;
#11116=CARTESIAN_POINT ( 'NONE',  ( -28.63582912838407069, 31.00000000000000355, 7.677129336082076705 ) ) ;
#11122=CARTESIAN_POINT ( 'NONE',  ( 65.81435062899562638, 31.00000000000000000, 37.99825742654716976 ) ) ;
#11127=CARTESIAN_POINT ( 'NONE',  ( -35.75974951333986240, 31.00000000000000355, 20.56794350806610794 ) ) ;
#11130=CARTESIAN_POINT ( 'NONE',  ( 24.81019160154284720, 40.00000000000000000, 73.04493173762017477 ) ) ;
#11140=CARTESIAN_POINT ( 'NONE',  ( -58.48566925782336057, 40.00000000000000711, -15.65830181329500803 ) ) ;
#11167=CARTESIAN_POINT ( 'NONE',  ( -36.61132647064156487, 31.00000000000000355, -18.04288060775211378 ) ) ;
#11177=CARTESIAN_POINT ( 'NONE',  ( -21.36651465564686703, 40.00000000000000000, 43.35257367405362317 ) ) ;
#11178=CARTESIAN_POINT ( 'NONE',  ( -13.93478910046542829, 40.00000000000000000, -52.37520058408175316 ) ) ;
#11186=EDGE_CURVE ( 'NONE', #6140, #25968, #6383, .T. ) ;
#11190=CARTESIAN_POINT ( 'NONE',  ( -20.07939870814534089, 40.00000000000000000, -2.638545259751242877 ) ) ;
#11203=CARTESIAN_POINT ( 'NONE',  ( 74.15939217261870908, 31.00000000000000000, -19.75058139460982432 ) ) ;
#11214=CARTESIAN_POINT ( 'NONE',  ( -55.31949386280459180, 40.00000000000000711, 71.91600076662652441 ) ) ;
#11224=CARTESIAN_POINT ( 'NONE',  ( -55.79431841392906222, 31.00000000000000355, -72.71543055464235294 ) ) ;
#11228=CARTESIAN_POINT ( 'NONE',  ( 19.49047152472583022, 40.00000000000000000, -17.07028940128360617 ) ) ;
#11254=DIRECTION ( 'NONE',  ( 0.000000000000000000, 0.000000000000000000, 1.000000000000000000 ) ) ;
#11256=CARTESIAN_POINT ( 'NONE',  ( 27.84166646522859878, 31.00000000000000355, -36.16032403484085478 ) ) ;
#11263=CARTESIAN_POINT ( 'NONE',  ( -48.52617905696451572, 40.00000000000000000, 37.10499320822106029 ) ) ;
#11273=CARTESIAN_POINT ( 'NONE',  ( -57.67632858778466698, 31.00000000000000711, 15.45560639130400205 ) ) ;
#11278=CARTESIAN_POINT ( 'NONE',  ( -14.08558183832706234, 40.00000000000000000, -28.55406316770863739 ) ) ;
#11283=CARTESIAN_POINT ( 'NONE',  ( 86.90011881125596460, 31.00000000000000000, -5.573058087428397478 ) ) ;
#11284=CARTESIAN_POINT ( 'NONE',  ( 82.09539989320980169, 39.99999999999999289, -27.75477508813643723 ) ) ;
#11299=CARTESIAN_POINT ( 'NONE',  ( 70.70367055548476287, 39.99999999999999289, -62.02616482874480397 ) ) ;
#11314=CARTESIAN_POINT ( 'NONE',  ( -27.06829236441420861, 40.00000000000000000, 15.58100167311933149 ) ) ;
#11325=CARTESIAN_POINT ( 'NONE',  ( 23.22631124480444598, 31.00000000000000355, -7.893869537065737241 ) ) ;
#11332=CARTESIAN_POINT ( 'NONE',  ( 41.75688748258168914, 31.00000000000000355, -72.32308762158416471 ) ) ;
#11335=CARTESIAN_POINT ( 'NONE',  ( -7.911223860809958097, 31.00000000000000355, 59.30865348673673765 ) ) ;
#11337=CARTESIAN_POINT ( 'NONE',  ( -85.90019077458921970, 40.00000000000000711, -29.16093118951848240 ) ) ;
#11350=CARTESIAN_POINT ( 'NONE',  ( -4.090615425948576522, 40.00000000000000000, -62.39583333438447710 ) ) ;
#11370=CARTESIAN_POINT ( 'NONE',  ( -22.00000000000000000, 40.00000000000000000, 1.283214542831021765 ) ) ;
#11381=CARTESIAN_POINT ( 'NONE',  ( -44.11856065373272173, 31.00000000000000355, -25.46949057303769948 ) ) ;
#11388=CARTESIAN_POINT ( 'NONE',  ( 55.68207322487837274, 39.99999999999999289, -32.16283696846894458 ) ) ;
#11389=CARTESIAN_POINT ( 'NONE',  ( 53.62204311759386854, 40.00000000000000000, -18.10832464707264577 ) ) ;
#11399=CARTESIAN_POINT ( 'NONE',  ( 28.66079171547214699, 40.00000000000000000, 21.97938003711830035 ) ) ;
#11401=CARTESIAN_POINT ( 'NONE',  ( -101.1532682021072134, 40.00000000000000000, -3.256983028635321187 ) ) ;
#11402=MECHANICAL_DESIGN_GEOMETRIC_PRESENTATION_REPRESENTATION('',(#40632),#5123);
#11414=CARTESIAN_POINT ( 'NONE',  ( 19.52887458859586545, 31.00000000000000355, -72.48875405280207929 ) ) ;
#11426=CARTESIAN_POINT ( 'NONE',  ( 91.58570893733640617, 39.99999999999999289, -30.97307622143650718 ) ) ;
#11427=CARTESIAN_POINT ( 'NONE',  ( -87.85203729262056527, 40.00000000000000711, 50.59313708112332364 ) ) ;
#11438=CARTESIAN_POINT ( 'NONE',  ( -100.0000000000000568, 31.00000000000000355, 2.687086664288074189E-12 ) ) ;
#11442=CARTESIAN_POINT ( 'NONE',  ( -7.718844055051848230, 40.00000000000000000, -22.75659427661715384 ) ) ;
#11466=VERTEX_POINT ( 'NONE', #17754 ) ;
#11469=CARTESIAN_POINT ( 'NONE',  ( -38.37160831357631707, 31.00000000000000355, -19.00137192356237392 ) ) ;
#11480=CARTESIAN_POINT ( 'NONE',  ( -58.36801134196149832, 40.00000000000000711, 19.71467013091580256 ) ) ;
#11484=DIRECTION ( 'NONE',  ( 0.000000000000000000, 1.000000000000000000, 0.000000000000000000 ) ) ;
#11492=CARTESIAN_POINT ( 'NONE',  ( -65.92798595308768483, 31.00000000000000711, 22.39357416381200849 ) ) ;
#11500=CARTESIAN_POINT ( 'NONE',  ( -77.35014290652780744, 31.00000000000000711, 26.14598721591455543 ) ) ;
#11501=CARTESIAN_POINT ( 'NONE',  ( -91.90012763196534706, 40.00000000000000711, 5.898218105444796855 ) ) ;
#11512=ORIENTED_EDGE ( 'NONE', *, *, #14083, .T. ) ;
#11516=CIRCLE ( 'NONE', #26829, 2.500000000000000444 ) ;
#11517=CARTESIAN_POINT ( 'NONE',  ( 72.43982367323130234, 39.99999999999999289, 63.53091779346544143 ) ) ;
#11530=CARTESIAN_POINT ( 'NONE',  ( 34.63398384099732397, 40.00000000000000000, -11.69655689657770559 ) ) ;
#11545=CARTESIAN_POINT ( 'NONE',  ( 14.35450763783260797, 31.00000000000000355, -18.72194639494853874 ) ) ;
#11551=CARTESIAN_POINT ( 'NONE',  ( -5.399612364985466151, 31.00000000000000355, -82.39583333413678190 ) ) ;
#11553=CARTESIAN_POINT ( 'NONE',  ( 42.13926417418816328, 31.00000000000000355, -36.83769365847010846 ) ) ;
#11554=CARTESIAN_POINT ( 'NONE',  ( 29.96647033545507455, 40.00000000000000000, -88.27250603610892199 ) ) ;
#11570=CARTESIAN_POINT ( 'NONE',  ( -54.58798567973315841, 40.00000000000000000, -26.90590473539369754 ) ) ;
#11586=DIRECTION ( 'NONE',  ( 0.000000000000000000, 1.541976423090494844E-15, 1.000000000000000000 ) ) ;
#11602=CARTESIAN_POINT ( 'NONE',  ( -3.108867721649295035, 31.00000000000000355, 47.60416666525765095 ) ) ;
#11611=CARTESIAN_POINT ( 'NONE',  ( -57.43240763726046794, 40.00000000000000000, -19.49446143887317717 ) ) ;
#11612=CARTESIAN_POINT ( 'NONE',  ( 51.84393115708665079, 40.00000000000000000, 25.66707601012906537 ) ) ;
#11619=CARTESIAN_POINT ( 'NONE',  ( 11.68784703496123711, 31.00000000000000355, -20.25319168173327355 ) ) ;
#11621=CARTESIAN_POINT ( 'NONE',  ( 14.71924655979513297, 40.00000000000000000, -29.87007926703815741 ) ) ;
#11638=CARTESIAN_POINT ( 'NONE',  ( -4.660665814385270167, 31.00000000000000355, 69.59371722956201722 ) ) ;
#11647=CARTESIAN_POINT ( 'NONE',  ( 59.96221986557397088, 40.00000000000000000, 78.35452998770438171 ) ) ;
#11649=CARTESIAN_POINT ( 'NONE',  ( 25.13348990051749254, 31.00000000000000355, -8.510361017572021680 ) ) ;
#11659=CARTESIAN_POINT ( 'NONE',  ( -60.10374203099167545, 31.00000000000000711, 78.35501831527777483 ) ) ;
#11664=CARTESIAN_POINT ( 'NONE',  ( 16.96065435355295392, 40.00000000000000000, -19.31014141889295743 ) ) ;
#11695=CARTESIAN_POINT ( 'NONE',  ( -21.81649963859176822, 31.00000000000000355, -37.93159502954523532 ) ) ;
#11707=CARTESIAN_POINT ( 'NONE',  ( 43.45541166192411708, 40.00000000000000000, -49.38773770141698805 ) ) ;
#11713=DIRECTION ( 'NONE',  ( 0.000000000000000000, 0.000000000000000000, 1.000000000000000000 ) ) ;
#11722=CARTESIAN_POINT ( 'NONE',  ( 28.01378275134445772, 31.00000000000000355, -56.83506808085938644 ) ) ;
#11730=CARTESIAN_POINT ( 'NONE',  ( -49.21613380539480431, 31.00000000000000355, 63.96793098899347996 ) ) ;
#11731=CARTESIAN_POINT ( 'NONE',  ( 76.16439905403352384, 39.99999999999999289, 44.11546174421767574 ) ) ;
#11732=ADVANCED_FACE ( 'NONE', ( #12260 ), #36718, .F. ) ;
#11755=CARTESIAN_POINT ( 'NONE',  ( -30.61154013076161107, 31.00000000000001776, 25.77968906985393716 ) ) ;
#11763=CARTESIAN_POINT ( 'NONE',  ( -28.46928290085317670, 40.00000000000000000, -16.49637127829624106 ) ) ;
#11778=CARTESIAN_POINT ( 'NONE',  ( 2.781618486875130358, 31.00000000000000355, -42.60416666509636485 ) ) ;
#11782=CARTESIAN_POINT ( 'NONE',  ( -62.77658523491555798, 31.00000000000000711, 48.16944601536268777 ) ) ;
#11784=CARTESIAN_POINT ( 'NONE',  ( 53.62204311759385433, 31.00000000000000355, -18.10832464707264577 ) ) ;
#11786=CARTESIAN_POINT ( 'NONE',  ( 81.87674480462379734, 39.99999999999999289, -21.93767060400471891 ) ) ;
#11800=CARTESIAN_POINT ( 'NONE',  ( 48.10206620145878276, 40.00000000000000000, -42.20136231105875879 ) ) ;
#11807=LINE ( 'NONE', #25131, #20098 ) ;
#11827=CARTESIAN_POINT ( 'NONE',  ( 34.77048308403384169, 31.00000000000000355, 30.48958026498159768 ) ) ;
#11832=CARTESIAN_POINT ( 'NONE',  ( -48.53848235557606472, 40.00000000000000000, -37.22912483484027035 ) ) ;
#11838=CARTESIAN_POINT ( 'NONE',  ( -20.07939870814534089, 31.00000000000000355, -2.638545259751242877 ) ) ;
#11841=CARTESIAN_POINT ( 'NONE',  ( 32.11716166826300167, 40.00000000000000000, 15.82712457579038912 ) ) ;
#11858=CARTESIAN_POINT ( 'NONE',  ( 5.085823974618866039, 31.00000000000000355, 79.40009828669005287 ) ) ;
#11866=CARTESIAN_POINT ( 'NONE',  ( 25.73918080462996372, 31.00000000000000355, -6.871072672212910959 ) ) ;
#11879=CARTESIAN_POINT ( 'NONE',  ( -12.78314611188302052, 31.00000000000000355, 97.07982689498881257 ) ) ;
#11882=CARTESIAN_POINT ( 'NONE',  ( 24.14050371820133023, 40.00000000000000000, 13.97356841391088444 ) ) ;
#11901=ORIENTED_EDGE ( 'NONE', *, *, #1846, .T. ) ;
#11910=CARTESIAN_POINT ( 'NONE',  ( 56.43498182460272972, 31.00000000000000355, -7.339809665447901921 ) ) ;
#11918=CARTESIAN_POINT ( 'NONE',  ( -56.48168293059611500, 40.00000000000000711, 43.19841958066528065 ) ) ;
#11932=CARTESIAN_POINT ( 'NONE',  ( -30.22953878324074495, 31.00000000000000355, 61.32923288305941867 ) ) ;
#11941=CARTESIAN_POINT ( 'NONE',  ( -50.81742119984753714, 31.00000000000000355, -66.42451308377114572 ) ) ;
#11942=CARTESIAN_POINT ( 'NONE',  ( 69.92891852059224789, 39.99999999999999289, 53.79372986807582180 ) ) ;
#11971=CARTESIAN_POINT ( 'NONE',  ( -3.925388345520635536, 40.00000000000000000, 29.51202942214662173 ) ) ;
#11981=ORIENTED_EDGE ( 'NONE', *, *, #23649, .T. ) ;
#11988=CARTESIAN_POINT ( 'NONE',  ( -10.91816144241376563, 31.00000000000000355, -40.73603723627661566 ) ) ;
#11990=SURFACE_STYLE_FILL_AREA ( #6258 ) ;
#11993=CARTESIAN_POINT ( 'NONE',  ( 21.49215960483416410, 31.00000000000000355, -80.26604385357094884 ) ) ;
#11995=CARTESIAN_POINT ( 'NONE',  ( 27.80911911935152503, 31.00000000000000355, -47.97225535896787108 ) ) ;
#11996=CARTESIAN_POINT ( 'NONE',  ( 43.43872713698582544, 40.00000000000000000, 75.20828420317944563 ) ) ;
#12000=AXIS2_PLACEMENT_3D ( 'NONE', #10156, #37200, #17181 ) ;
#12010=CARTESIAN_POINT ( 'NONE',  ( -69.34045338167970840, 40.00000000000000711, 9.142281554609933636 ) ) ;
#12015=CARTESIAN_POINT ( 'NONE',  ( -31.37281731866679024, 17.11489954122029289, 27.62913683693880174 ) ) ;
#12042=CARTESIAN_POINT ( 'NONE',  ( 36.61186797162192619, 31.00000000000000355, 28.07927795628900469 ) ) ;
#12044=ORIENTED_EDGE ( 'NONE', *, *, #33329, .F. ) ;
#12048=CARTESIAN_POINT ( 'NONE',  ( -53.27196957865878346, 40.00000000000000711, 26.27224001323269320 ) ) ;
#12054=CARTESIAN_POINT ( 'NONE',  ( -24.68525358734468611, 40.00000000000000000, -18.92943107747915832 ) ) ;
#12067=CARTESIAN_POINT ( 'NONE',  ( 52.26791824981292223, 31.00000000000000355, -67.94187691988643962 ) ) ;
#12077=CARTESIAN_POINT ( 'NONE',  ( 15.59370980024835696, 31.00000000000000355, -20.29731371384564653 ) ) ;
#12088=CARTESIAN_POINT ( 'NONE',  ( 72.43982367323130234, 31.00000000000000000, 63.53091779346544143 ) ) ;
#12092=CARTESIAN_POINT ( 'NONE',  ( -7.231618336280544845, 40.00000000000000000, 27.02512817425793656 ) ) ;
#12093=CARTESIAN_POINT ( 'NONE',  ( 12.49611804805956439, 40.00000000000000000, 37.00809541493615740 ) ) ;
#12119=CARTESIAN_POINT ( 'NONE',  ( -33.53193138075044999, 31.00000000000000355, 38.09769221459629307 ) ) ;
#12126=CARTESIAN_POINT ( 'NONE',  ( 72.60479858918233731, 39.99999999999999289, -24.53750584076950858 ) ) ;
#12138=CARTESIAN_POINT ( 'NONE',  ( 17.40022565512299479, 31.00000000000000355, 64.93645345284011228 ) ) ;
#12148=CARTESIAN_POINT ( 'NONE',  ( 5.650912336215120568, 31.00000000000000355, -84.59266001507907617 ) ) ;
#12149=CARTESIAN_POINT ( 'NONE',  ( -21.69137426901471954, 40.00000000000000000, -81.42030341110599068 ) ) ;
#12180=CARTESIAN_POINT ( 'NONE',  ( -11.35616125661516307, 40.00000000000000000, -42.69191301636733726 ) ) ;
#12192=CARTESIAN_POINT ( 'NONE',  ( 34.56606645648713538, 31.00000000000000355, -4.560848911255810378 ) ) ;
#12198=CARTESIAN_POINT ( 'NONE',  ( 64.90595555533579386, 31.00000000000000000, 56.92265028768127166 ) ) ;
#12202=CARTESIAN_POINT ( 'NONE',  ( -50.71442127988192539, 31.00000000000000355, -13.67646662467867991 ) ) ;
#12204=CARTESIAN_POINT ( 'NONE',  ( 57.06996419936330511, 39.99999999999999289, 65.05326946697847745 ) ) ;
#12219=CARTESIAN_POINT ( 'NONE',  ( -75.41724699911947027, 40.00000000000000711, 25.61573074746135248 ) ) ;
#12244=CARTESIAN_POINT ( 'NONE',  ( -44.28363997456384737, 31.00000000000000355, 21.84072794957603492 ) ) ;
#12250=CARTESIAN_POINT ( 'NONE',  ( -46.07128526072433772, 40.00000000000000000, -40.40198152342698990 ) ) ;
#12260=FACE_OUTER_BOUND ( 'NONE', #13491, .T. ) ;
#12264=CARTESIAN_POINT ( 'NONE',  ( -19.19493090124598922, 40.00000000000000000, -25.00897302100653263 ) ) ;
#12277=CARTESIAN_POINT ( 'NONE',  ( 87.09251733236551729, 31.00000000000000000, 5.815661930448015937 ) ) ;
#12287=CARTESIAN_POINT ( 'NONE',  ( 1.888402776346428835, 31.00000000000000355, 29.39821258742166066 ) ) ;
#12303=CARTESIAN_POINT ( 'NONE',  ( 20.70971545910534672, 40.00000000000000000, 15.87948211774388518 ) ) ;
#12304=CARTESIAN_POINT ( 'NONE',  ( -20.36888183406675168, 40.00000000000000000, -26.63352584488937325 ) ) ;
#12328=CARTESIAN_POINT ( 'NONE',  ( -49.27414759474276451, 40.00000000000000711, 85.34056160678568403 ) ) ;
#12336=CARTESIAN_POINT ( 'NONE',  ( 50.14038141241295676, 31.00000000000000355, 29.06424286984032435 ) ) ;
#12343=CARTESIAN_POINT ( 'NONE',  ( 19.52887458859586900, 40.00000000000000000, -72.48875405283516216 ) ) ;
#12358=CARTESIAN_POINT ( 'NONE',  ( 63.32575250126041055, 31.00000000000000000, 16.95471465585521997 ) ) ;
#12368=CARTESIAN_POINT ( 'NONE',  ( -89.42636861580037078, 31.00000000000000711, -24.07434901466544730 ) ) ;
#12369=CARTESIAN_POINT ( 'NONE',  ( -56.91377077966711084, 40.00000000000000000, -74.37798324515208037 ) ) ;
#12390=CARTESIAN_POINT ( 'NONE',  ( -14.30682334061562067, 31.00000000000000355, -18.65445469299708492 ) ) ;
#12397=CARTESIAN_POINT ( 'NONE',  ( 5.076274692535532651, 40.00000000000000000, 39.04542013319162663 ) ) ;
#12408=CARTESIAN_POINT ( 'NONE',  ( -32.63632984357925437, 31.00000000000000355, -25.02932899672474676 ) ) ;
#12417=CARTESIAN_POINT ( 'NONE',  ( 89.65113856817994531, 31.00000000000000000, -30.44896562292877462 ) ) ;
#12422=CARTESIAN_POINT ( 'NONE',  ( 60.82800096162477388, 31.00000000000000000, 30.10617641798563682 ) ) ;
#12423=CARTESIAN_POINT ( 'NONE',  ( -22.66037885604484359, 40.00000000000000000, 66.40833514169634100 ) ) ;
#12424=CARTESIAN_POINT ( 'NONE',  ( -65.18298466990795248, 40.00000000000000711, 74.32329070269128124 ) ) ;
#12436=CARTESIAN_POINT ( 'NONE',  ( -35.92146702467432817, 40.00000000000000000, -62.19081021767443218 ) ) ;
#12467=CARTESIAN_POINT ( 'NONE',  ( -52.79687664379660816, 31.00000000000000355, -30.48099731442381710 ) ) ;
#12472=CARTESIAN_POINT ( 'NONE',  ( -67.35649507452052376, 40.00000000000000711, 18.04843207638801772 ) ) ;
#12481=CARTESIAN_POINT ( 'NONE',  ( -25.29482881991252086, 40.00000000000000000, -32.96004927633274662 ) ) ;
#12491=CARTESIAN_POINT ( 'NONE',  ( -21.03271207055027503, 17.11489954122026447, 3.044856699593507354 ) ) ;
#12492=CARTESIAN_POINT ( 'NONE',  ( 74.83201185292551827, 31.00000000000000000, -43.08100868842220166 ) ) ;
#12512=CARTESIAN_POINT ( 'NONE',  ( 13.36968668718156295, 31.00000000000000355, 23.13838826010315941 ) ) ;
#12518=CARTESIAN_POINT ( 'NONE',  ( 8.699408683037360035, 40.00000000000000000, 25.59862650653646909 ) ) ;
#12519=CARTESIAN_POINT ( 'NONE',  ( 2.319640971205140900, 40.00000000000000000, -34.59922639972668890 ) ) ;
#12538=CARTESIAN_POINT ( 'NONE',  ( -72.39171112334068425, 40.00000000000000711, -55.52881859171880308 ) ) ;
#12546=CARTESIAN_POINT ( 'NONE',  ( -35.18788409414197815, 31.00000000000000355, -40.25400722681192178 ) ) ;
#12551=CARTESIAN_POINT ( 'NONE',  ( 47.76959191294547935, 40.00000000000000000, 62.44753968353898443 ) ) ;
#12560=DIRECTION ( 'NONE',  ( 0.000000000000000000, 1.000000000000000000, 0.000000000000000000 ) ) ;
#12565=CARTESIAN_POINT ( 'NONE',  ( -10.77850749866037816, 31.00000000000000355, -81.75987728344749428 ) ) ;
#12574=CARTESIAN_POINT ( 'NONE',  ( -83.29221842953128885, 31.00000000000000711, -41.19657635674187190 ) ) ;
#12575=CARTESIAN_POINT ( 'NONE',  ( -12.22491041697691294, 40.00000000000000000, -93.69500887688228374 ) ) ;
#12599=CARTESIAN_POINT ( 'NONE',  ( 2.511863649308039736, 40.00000000000000000, 39.39933062585536305 ) ) ;
#12615=CARTESIAN_POINT ( 'NONE',  ( 10.63353083439206870, 31.00000000000000355, -31.33693976183458219 ) ) ;
#12621=CARTESIAN_POINT ( 'NONE',  ( 12.12865573427490062, 31.00000000000000355, -92.11205733446308841 ) ) ;
#12625=CARTESIAN_POINT ( 'NONE',  ( 57.47007747236072817, 31.00000000000000000, -33.06854485811727784 ) ) ;
#12626=CARTESIAN_POINT ( 'NONE',  ( 49.67886955981430219, 40.00000000000000000, -43.43868092391004865 ) ) ;
#12639=CARTESIAN_POINT ( 'NONE',  ( 44.85399723358655422, 40.00000000000000000, -58.47732767552992073 ) ) ;
#12669=CARTESIAN_POINT ( 'NONE',  ( 53.64558601427197004, 31.00000000000000355, 14.36188897069615500 ) ) ;
#12675=CARTESIAN_POINT ( 'NONE',  ( -24.93870012978733541, 31.00000000000000355, -21.94074674037795702 ) ) ;
#12677=CARTESIAN_POINT ( 'NONE',  ( 65.10416666562252885, 39.99999999999999289, 4.254240043327690124 ) ) ;
#12685=CARTESIAN_POINT ( 'NONE',  ( -49.89583333467011528, 40.00000000000000000, 3.272492339034415831 ) ) ;
#12700=CARTESIAN_POINT ( 'NONE',  ( -77.35014290652780744, 31.00000000000000711, 26.14598721591455543 ) ) ;
#12710=CARTESIAN_POINT ( 'NONE',  ( -44.52253807734693680, 40.00000000000000000, 90.03212995793734308 ) ) ;
#12718=CARTESIAN_POINT ( 'NONE',  ( -4.233603722440171246, 31.00000000000000355, -32.08218167604271542 ) ) ;
#12725=CARTESIAN_POINT ( 'NONE',  ( 28.66079171547214699, 40.00000000000000000, 21.97938003711830035 ) ) ;
#12726=CARTESIAN_POINT ( 'NONE',  ( -28.46928290085317670, 40.00000000000000000, -16.49637127829624106 ) ) ;
#12732=VECTOR ( 'NONE', #31371, 1000.000000000000114 ) ;
#12755=CARTESIAN_POINT ( 'NONE',  ( -13.93478910046839125, 31.00000000000000355, -52.37520058406987999 ) ) ;
#12762=CARTESIAN_POINT ( 'NONE',  ( -9.228224334387265415, 40.00000000000000000, 69.24269282083176336 ) ) ;
#12775=CARTESIAN_POINT ( 'NONE',  ( -10.16518460146908787, 31.00000000000000355, 77.20874865269769316 ) ) ;
#12783=CARTESIAN_POINT ( 'NONE',  ( -68.52217190868857699, 31.00000000000000711, 59.94826526066079708 ) ) ;
#12784=CARTESIAN_POINT ( 'NONE',  ( -61.42214656771047743, 40.00000000000000711, 79.86467493626639680 ) ) ;
#12803=CARTESIAN_POINT ( 'NONE',  ( -22.00000000000000000, 31.00000000000000355, 0.000000000000000000 ) ) ;
#12811=CARTESIAN_POINT ( 'NONE',  ( -19.32876798325328949, 40.00000000000000000, -39.37500834187648735 ) ) ;
#12824=CARTESIAN_POINT ( 'NONE',  ( 45.10416666515585860, 31.00000000000000355, 2.945243104263102651 ) ) ;
#12825=( LENGTH_UNIT ( ) NAMED_UNIT ( * ) SI_UNIT ( .MILLI., .METRE. ) );
#12829=CARTESIAN_POINT ( 'NONE',  ( -72.39171112334068425, 31.00000000000000711, -55.52881859171880308 ) ) ;
#12833=CARTESIAN_POINT ( 'NONE',  ( 4.437437895627577511, 31.00000000000000355, 69.40004907510417809 ) ) ;
#12834=CARTESIAN_POINT ( 'NONE',  ( -72.09351246578157202, 40.00000000000000711, -4.825959690424619808 ) ) ;
#12835=CARTESIAN_POINT ( 'NONE',  ( -89.22528799552154055, 40.00000000000000711, 43.99828826784794700 ) ) ;
#12850=CARTESIAN_POINT ( 'NONE',  ( 73.00591898829820536, 39.99999999999999289, 19.54754034098114701 ) ) ;
#12881=CARTESIAN_POINT ( 'NONE',  ( -27.38011802910879311, 31.00000000000000355, -55.51905197969063011 ) ) ;
#12885=CARTESIAN_POINT ( 'NONE',  ( 10.06970066534735331, 31.00000000000000355, 37.84957806120349488 ) ) ;
#12886=CARTESIAN_POINT ( 'NONE',  ( 66.75446398494719347, 39.99999999999999289, -32.91950810868348043 ) ) ;
#12898=CARTESIAN_POINT ( 'NONE',  ( 38.32544124395173668, 40.00000000000000000, -22.13982348525413002 ) ) ;
#12914=CARTESIAN_POINT ( 'NONE',  ( -12.22491041698737746, 31.00000000000000355, -93.69500887688226953 ) ) ;
#12918=CARTESIAN_POINT ( 'NONE',  ( -105.9879088449591933, 40.00000000000000000, -0.3807199291576673361 ) ) ;
#12928=CIRCLE ( 'NONE', #38692, 2.500000000000002665 ) ;
#12931=CARTESIAN_POINT ( 'NONE',  ( -25.30796725786148826, 31.00000000000000355, 14.62256337265529815 ) ) ;
#12942=CARTESIAN_POINT ( 'NONE',  ( 27.23661496637203427, 40.00000000000000000, 23.88131275951389654 ) ) ;
#12943=CARTESIAN_POINT ( 'NONE',  ( -2.659806967433698599, 40.00000000000000000, 39.59793253468611596 ) ) ;
#12973=CARTESIAN_POINT ( 'NONE',  ( 32.82854187708761629, 31.00000000000000355, -56.64543409046200395 ) ) ;
#12975=EDGE_CURVE ( 'NONE', #1383, #42412, #29627, .T. ) ;
#12984=CARTESIAN_POINT ( 'NONE',  ( -5.321195512787074478, 40.00000000000000000, 79.59297073838583003 ) ) ;
#12994=CARTESIAN_POINT ( 'NONE',  ( -76.41092972884307244, 31.00000000000000711, -25.93877460596726436 ) ) ;
#13009=CARTESIAN_POINT ( 'NONE',  ( 91.58570893733639195, 31.00000000000000000, -30.97307622143650363 ) ) ;
#13011=CARTESIAN_POINT ( 'NONE',  ( -24.28006566513952791, 40.00000000000000000, -91.10131089348455191 ) ) ;
#13029=CARTESIAN_POINT ( 'NONE',  ( 23.62253089228586234, 31.00000000000000355, -11.62353008834390167 ) ) ;
#13040=CARTESIAN_POINT ( 'NONE',  ( -25.29816761084670063, 40.00000000000000000, 43.63644233508315295 ) ) ;
#13053=CARTESIAN_POINT ( 'NONE',  ( 13.85568741775851542, 31.00000000000000355, -40.82620080729295609 ) ) ;
#13062=CARTESIAN_POINT ( 'NONE',  ( -68.67288961433401084, 31.00000000000000711, -60.22678404055071155 ) ) ;
#13065=CARTESIAN_POINT ( 'NONE',  ( 30.38134496340387969, 31.00000000000000355, 61.85720693093856681 ) ) ;
#13066=CARTESIAN_POINT ( 'NONE',  ( 63.11376326756305843, 39.99999999999999289, -21.32174659672108774 ) ) ;
#13068=CARTESIAN_POINT ( 'NONE',  ( 95.10416666600561086, 39.99999999999999289, 6.217735451873073416 ) ) ;
#13083=CARTESIAN_POINT ( 'NONE',  ( -4.745113895469965648, 40.00000000000000000, -72.39583333427917466 ) ) ;
#13112=CARTESIAN_POINT ( 'NONE',  ( 28.01378275134445772, 31.00000000000000355, -56.83506808085938644 ) ) ;
#13116=CARTESIAN_POINT ( 'NONE',  ( -24.64063138600606351, 31.00000000000000355, 18.85097431369995746 ) ) ;
#13117=CARTESIAN_POINT ( 'NONE',  ( -31.81163009274181519, 40.00000000000000000, -64.50738158386226928 ) ) ;
#13118=EDGE_CURVE ( 'NONE', #6230, #9181, #25945, .T. ) ;
#13128=CARTESIAN_POINT ( 'NONE',  ( 44.91824650936478491, 40.00000000000000000, 5.910997147197376123 ) ) ;
#13132=ORIENTED_EDGE ( 'NONE', *, *, #21035, .T. ) ;
#13141=CARTESIAN_POINT ( 'NONE',  ( -82.08563009789774867, 31.00000000000000711, 40.34115885382633593 ) ) ;
#13157=CARTESIAN_POINT ( 'NONE',  ( 25.50046184691807483, 31.00000000000000355, -22.37655979312362931 ) ) ;
#13164=CARTESIAN_POINT ( 'NONE',  ( 34.28525303991722240, 40.00000000000000000, 9.176237600273646322 ) ) ;
#13165=CARTESIAN_POINT ( 'NONE',  ( 12.64472494877221997, 40.00000000000000000, 47.53373494968590762 ) ) ;
#13167=ORIENTED_EDGE ( 'NONE', *, *, #13118, .T. ) ;
#13178=CARTESIAN_POINT ( 'NONE',  ( -105.9879088449591933, 31.00000000000000355, -0.3807199291576673361 ) ) ;
#13194=CARTESIAN_POINT ( 'NONE',  ( 64.03668805592332092, 31.00000000000000000, 21.85318084035846198 ) ) ;
#13201=CARTESIAN_POINT ( 'NONE',  ( 34.80713033128647993, 40.00000000000000000, 70.84796410819511436 ) ) ;
#13210=CARTESIAN_POINT ( 'NONE',  ( -49.69442049507403425, 31.00000000000000355, -64.76435429890716478 ) ) ;
#13217=VECTOR ( 'NONE', #36691, 999.9999999999998863 ) ;
#13225=CARTESIAN_POINT ( 'NONE',  ( 12.51314706078824912, 31.00000000000000355, -94.07914177284597201 ) ) ;
#13239=PLANE ( 'NONE',  #1998 ) ;
#13242=CARTESIAN_POINT ( 'NONE',  ( 23.40755275317545880, 31.00000000000000355, 30.61714766194360138 ) ) ;
#13248=CYLINDRICAL_SURFACE ( 'NONE', #17522, 4.500000000000000888 ) ;
#13253=CARTESIAN_POINT ( 'NONE',  ( -3.331996295684063636, 40.00000000000000000, 49.59602437329134972 ) ) ;
#13262=CARTESIAN_POINT ( 'NONE',  ( -40.58740609958903889, 31.00000000000000355, -31.12922691583434798 ) ) ;
#13268=CARTESIAN_POINT ( 'NONE',  ( 10.28773449565296083, 40.00000000000000000, -20.88174966193524895 ) ) ;
#13276=CARTESIAN_POINT ( 'NONE',  ( -59.63693792270941429, 31.00000000000000711, 15.87187584493272929 ) ) ;
#13277=CARTESIAN_POINT ( 'NONE',  ( 16.92944795087012722, 40.00000000000000000, -62.81076020707057950 ) ) ;
#13290=CARTESIAN_POINT ( 'NONE',  ( -77.37786320076959612, 40.00000000000000711, 44.69160382239309115 ) ) ;
#13306=CARTESIAN_POINT ( 'NONE',  ( -3.169834189307653816, 40.00000000000000000, -24.13593742708953727 ) ) ;
#13318=CARTESIAN_POINT ( 'NONE',  ( -20.10416666680962550, 31.00000000000000355, -1.308996940106889273 ) ) ;
#13324=CARTESIAN_POINT ( 'NONE',  ( -35.70415035507907930, 31.00000000000000355, 46.55071329160319493 ) ) ;
#13327=CARTESIAN_POINT ( 'NONE',  ( 2.319640971205256363, 31.00000000000000355, -34.59922639972668179 ) ) ;
#13328=CARTESIAN_POINT ( 'NONE',  ( -4.417864660710832503, 40.00000000000000000, 67.60416666563759236 ) ) ;
#13338=CARTESIAN_POINT ( 'NONE',  ( -2.781618486875174767, 40.00000000000000000, -42.39583333490362804 ) ) ;
#13354=CARTESIAN_POINT ( 'NONE',  ( 92.49871336439160530, 31.00000000000000000, 31.53380891771210415 ) ) ;
#13370=CARTESIAN_POINT ( 'NONE',  ( -2.127120017302697619, 31.00000000000000355, -32.39583333539214038 ) ) ;
#13378=CARTESIAN_POINT ( 'NONE',  ( 33.03432996520027132, 40.00000000000000000, -28.98482729919588863 ) ) ;
#13379=CARTESIAN_POINT ( 'NONE',  ( -28.59133019391067165, 40.00000000000000000, -32.71076623427350683 ) ) ;
#13404=CARTESIAN_POINT ( 'NONE',  ( -26.77709713317330653, 31.00000000000000355, 54.08981485145582013 ) ) ;
#13413=CARTESIAN_POINT ( 'NONE',  ( 52.26791824981292933, 40.00000000000000000, -67.94187691988643962 ) ) ;
#13417=CARTESIAN_POINT ( 'NONE',  ( -101.6738636939643357, 31.00000000000000000, -5.192942712545359107 ) ) ;
#13425=CARTESIAN_POINT ( 'NONE',  ( 71.66629920589342362, 31.00000000000000000, 24.32769631419027689 ) ) ;
#13456=CARTESIAN_POINT ( 'NONE',  ( 28.62564328229763788, 31.00000000000000355, -21.88780996306212501 ) ) ;
#13467=CARTESIAN_POINT ( 'NONE',  ( -46.12092335263332643, 40.00000000000000000, 22.64177125690310177 ) ) ;
#13476=CARTESIAN_POINT ( 'NONE',  ( 44.89583333484414140, 31.00000000000000355, -2.945243104263157274 ) ) ;
#13482=CARTESIAN_POINT ( 'NONE',  ( -19.47536345555549886, 40.00000000000000000, -6.605835105517199324 ) ) ;
#13487=CARTESIAN_POINT ( 'NONE',  ( 50.06853320191206791, 31.00000000000000000, -56.91684085115753078 ) ) ;
#13488=CARTESIAN_POINT ( 'NONE',  ( -60.98551593176824070, 40.00000000000000711, 53.34359504439791522 ) ) ;
#13491=EDGE_LOOP ( 'NONE', ( #10134, #7032, #35893, #41611 ) ) ;
#13502=CARTESIAN_POINT ( 'NONE',  ( 74.49266661913014786, 39.99999999999999289, 43.00976416799198176 ) ) ;
#13516=CARTESIAN_POINT ( 'NONE',  ( -19.81637295874436333, 40.00000000000000000, -11.44243563873878777 ) ) ;
#13529=ORIENTED_EDGE ( 'NONE', *, *, #42224, .T. ) ;
#13534=CARTESIAN_POINT ( 'NONE',  ( 43.85342918759069164, 31.00000000000000355, 49.98553323097543455 ) ) ;
#13538=CARTESIAN_POINT ( 'NONE',  ( 25.29542371717656835, 31.00000000000000355, 28.93716311998947788 ) ) ;
#13541=CARTESIAN_POINT ( 'NONE',  ( 46.64447153568531945, 40.00000000000000000, 60.78881617101084345 ) ) ;
#13550=CARTESIAN_POINT ( 'NONE',  ( 26.72236725836960147, 40.00000000000000000, -46.28813965123160301 ) ) ;
#13552=AXIS2_PLACEMENT_3D ( 'NONE', #3852, #14597, #10213 ) ;
#13566=CARTESIAN_POINT ( 'NONE',  ( 73.86091552538547944, 31.00000000000000000, 64.94433634442138725 ) ) ;
#13578=LINE ( 'NONE', #36890, #33783 ) ;
#13584=CARTESIAN_POINT ( 'NONE',  ( -5.542584477697039880, 31.00000000000000355, -42.01772079774592328 ) ) ;
#13592=CARTESIAN_POINT ( 'NONE',  ( 38.32544124395173668, 40.00000000000000000, -22.13982348525413002 ) ) ;
#13594=CARTESIAN_POINT ( 'NONE',  ( 46.49836147156941735, 40.00000000000000000, -6.043767708841586206 ) ) ;
#13604=CARTESIAN_POINT ( 'NONE',  ( 10.28773449565296083, 40.00000000000000000, -20.88174966193524895 ) ) ;
#13620=CARTESIAN_POINT ( 'NONE',  ( 8.570044366903687205, 31.00000000000000355, -64.27561742005508449 ) ) ;
#13622=CARTESIAN_POINT ( 'NONE',  ( -100.0589655806010967, 31.00000000000001421, 21.59728106529621172 ) ) ;
#13629=CARTESIAN_POINT ( 'NONE',  ( -50.81742119984753714, 40.00000000000000000, -66.42451308377114572 ) ) ;
#13636=ORIENTED_EDGE ( 'NONE', *, *, #25433, .F. ) ;
#13642=CARTESIAN_POINT ( 'NONE',  ( -40.67465422008825726, 31.00000000000000355, -82.48404079236435393 ) ) ;
#13671=CARTESIAN_POINT ( 'NONE',  ( -9.709369018688816411, 31.00000000000000355, 28.47525938324675820 ) ) ;
#13679=CARTESIAN_POINT ( 'NONE',  ( 17.81483206086863191, 40.00000000000000000, -52.17936214187551514 ) ) ;
#13688=AXIS2_PLACEMENT_3D ( 'NONE', #37604, #17375, #7722 ) ;
#13692=CARTESIAN_POINT ( 'NONE',  ( -21.36651465564686703, 31.00000000000000355, 43.35257367405362317 ) ) ;
#13701=CARTESIAN_POINT ( 'NONE',  ( 6.381360069253262601, 31.00000000000000355, 97.39583333395333398 ) ) ;
#13704=CARTESIAN_POINT ( 'NONE',  ( -63.15125318179580205, 31.00000000000000711, -36.59163237598400542 ) ) ;
#13705=CARTESIAN_POINT ( 'NONE',  ( -81.27520743796613090, 40.00000000000000711, 10.59408403753070083 ) ) ;
#13724=CARTESIAN_POINT ( 'NONE',  ( 66.75212336275305347, 39.99999999999999289, -51.21939497476837744 ) ) ;
#13737=CARTESIAN_POINT ( 'NONE',  ( 19.49047152472583022, 40.00000000000000000, -17.07028940128360617 ) ) ;
#13756=CARTESIAN_POINT ( 'NONE',  ( 52.51402048354923835, 31.00000000000000355, 40.27907379435107060 ) ) ;
#13760=CARTESIAN_POINT ( 'NONE',  ( 29.49207856985708176, 31.00000000000000355, 38.57905506995707867 ) ) ;
#13762=CARTESIAN_POINT ( 'NONE',  ( 74.89583333416871369, 39.99999999999999289, -4.908738512848213276 ) ) ;
#13764=ADVANCED_FACE ( 'NONE', ( #7280 ), #4000, .F. ) ;
#13773=CARTESIAN_POINT ( 'NONE',  ( 40.56819808336118882, 40.00000000000000000, -35.59309480518532354 ) ) ;
#13792=CARTESIAN_POINT ( 'NONE',  ( -61.59955500562279695, 31.00000000000000711, -70.40623950599746195 ) ) ;
#13810=CARTESIAN_POINT ( 'NONE',  ( -2.781618486875174767, 31.00000000000000355, -42.39583333490362804 ) ) ;
#13817=CARTESIAN_POINT ( 'NONE',  ( 42.89889459577944564, 40.00000000000000000, -32.91970121835214513 ) ) ;
#13819=CARTESIAN_POINT ( 'NONE',  ( 30.22238470470974292, 40.00000000000000000, -34.33595424619393555 ) ) ;
#13829=CARTESIAN_POINT ( 'NONE',  ( 8.699408683037360035, 40.00000000000000000, 25.59862650653646909 ) ) ;
#13843=CARTESIAN_POINT ( 'NONE',  ( -59.29355402628473115, 31.00000000000000355, -20.23837177251482800 ) ) ;
#13857=CARTESIAN_POINT ( 'NONE',  ( -37.02054590706428172, 40.00000000000000000, -75.34311506435015815 ) ) ;
#13867=CARTESIAN_POINT ( 'NONE',  ( 36.87680687886029318, 31.00000000000000355, -74.81172728975037955 ) ) ;
#13891=CARTESIAN_POINT ( 'NONE',  ( 21.72498709342646706, 31.00000000000000355, -28.22316639787266013 ) ) ;
#13897=UNCERTAINTY_MEASURE_WITH_UNIT (LENGTH_MEASURE( 1.000000000000000082E-05 ), #159, 'distance_accuracy_value', 'NONE');
#13900=CARTESIAN_POINT ( 'NONE',  ( -33.53193138075045709, 40.00000000000000000, 38.09769221459629307 ) ) ;
#13913=CARTESIAN_POINT ( 'NONE',  ( 52.83624534446448706, 31.00000000000000355, -14.15919354876300318 ) ) ;
#13918=CARTESIAN_POINT ( 'NONE',  ( 23.22631124480444598, 40.00000000000000000, -7.893869537065737241 ) ) ;
#13919=ORIENTED_EDGE ( 'NONE', *, *, #31879, .F. ) ;
#13922=CARTESIAN_POINT ( 'NONE',  ( -68.78002826185903018, 31.00000000000000711, -23.46745878763085358 ) ) ;
#13923=CARTESIAN_POINT ( 'NONE',  ( 76.30724621505197547, 39.99999999999999289, -9.942258256684034734 ) ) ;
#13938=CARTESIAN_POINT ( 'NONE',  ( 26.74431375183570481, 40.00000000000000000, -78.78324499025107741 ) ) ;
#13964=CARTESIAN_POINT ( 'NONE',  ( 11.86982580658625075, 31.00000000000000355, 24.05989836594520526 ) ) ;
#13969=CARTESIAN_POINT ( 'NONE',  ( 62.17703816010947548, 31.00000000000000000, 21.10553973062999589 ) ) ;
#13971=CARTESIAN_POINT ( 'NONE',  ( 14.57966847436265212, 31.00000000000000355, -42.69519604896471776 ) ) ;
#13972=CARTESIAN_POINT ( 'NONE',  ( 26.74431375183570481, 40.00000000000000000, -78.78324499025107741 ) ) ;
#13983=CARTESIAN_POINT ( 'NONE',  ( 7.506055610550203205, 40.00000000000000000, 56.92102948000351148 ) ) ;
#14016=CARTESIAN_POINT ( 'NONE',  ( 2.454369252093185239, 31.00000000000000355, 37.39583333513270702 ) ) ;
#14021=AXIS2_PLACEMENT_3D ( 'NONE', #17673, #14376, #40729 ) ;
#14027=CARTESIAN_POINT ( 'NONE',  ( -32.14164714139042189, 40.00000000000000000, 36.65395011347077059 ) ) ;
#14028=CARTESIAN_POINT ( 'NONE',  ( -55.11358496761538106, 40.00000000000000711, 27.06326608206703099 ) ) ;
#14038=CARTESIAN_POINT ( 'NONE',  ( 17.96659372829068246, 40.00000000000000000, -15.76829228678407624 ) ) ;
#14049=DIRECTION ( 'NONE',  ( 0.000000000000000000, 1.000000000000000000, 0.000000000000000000 ) ) ;
#14056=CARTESIAN_POINT ( 'NONE',  ( -63.15125318179580205, 31.00000000000000711, -36.59163237598400542 ) ) ;
#14064=CARTESIAN_POINT ( 'NONE',  ( -11.85673204381699364, 40.00000000000000000, 89.11174773313419450 ) ) ;
#14076=CARTESIAN_POINT ( 'NONE',  ( 5.726861599741335240, 31.00000000000000355, 87.39583333411552246 ) ) ;
#14080=AXIS2_PLACEMENT_3D ( 'NONE', #23241, #17355, #30635 ) ;
#14083=EDGE_CURVE ( 'NONE', #20422, #5066, #34590, .T. ) ;
#14097=DIRECTION ( 'NONE',  ( 0.3211947320043981313, 0.000000000000000000, 0.9470131699890043109 ) ) ;
#14108=CARTESIAN_POINT ( 'NONE',  ( 11.33656872182281816, 31.00000000000000355, -33.21392199183605243 ) ) ;
#14115=CARTESIAN_POINT ( 'NONE',  ( 65.23019871244166268, 39.99999999999999289, 17.57949444736078703 ) ) ;
#14126=CARTESIAN_POINT ( 'NONE',  ( -60.10416666555506993, 31.00000000000000711, -3.926990808566252156 ) ) ;
#14128=EDGE_LOOP ( 'NONE', ( #17641, #9148, #19832, #25654 ) ) ;
#14131=CARTESIAN_POINT ( 'NONE',  ( -14.11622541012940601, 40.00000000000000000, -16.08312669853564358 ) ) ;
#14135=CARTESIAN_POINT ( 'NONE',  ( -48.39074809477736494, 31.00000000000000355, -55.33250407651094349 ) ) ;
#14136=CARTESIAN_POINT ( 'NONE',  ( -63.15125318177969405, 40.00000000000000711, -36.59163237596791163 ) ) ;
#14153=CARTESIAN_POINT ( 'NONE',  ( -70.15350862410126354, 40.00000000000000711, -40.50401079722123399 ) ) ;
#14164=CARTESIAN_POINT ( 'NONE',  ( -21.70016380022027391, 40.00000000000000000, -5.809120511592388958 ) ) ;
#14174=CARTESIAN_POINT ( 'NONE',  ( 19.70274684888802952, 31.00000000000000355, 17.27304525429847359 ) ) ;
#14176=CARTESIAN_POINT ( 'NONE',  ( -16.80298683001096904, 17.11489954122026447, -2.367532924972506336 ) ) ;
#14180=CARTESIAN_POINT ( 'NONE',  ( -56.48955861152074220, 31.00000000000000711, -43.32902275382048174 ) ) ;
#14182=CARTESIAN_POINT ( 'NONE',  ( 30.22238470471967631, 31.00000000000000355, -34.33595424619392844 ) ) ;
#14184=CARTESIAN_POINT ( 'NONE',  ( -53.76583044639610165, 40.00000000000000000, -61.28633540801820345 ) ) ;
#14198=CARTESIAN_POINT ( 'NONE',  ( -25.79802671946675474, 40.00000000000000000, 52.34090327860478453 ) ) ;
#14227=CARTESIAN_POINT ( 'NONE',  ( 43.15607885788778475, 31.00000000000000355, -11.56636786368396486 ) ) ;
#14230=CARTESIAN_POINT ( 'NONE',  ( -15.99999999999997691, 40.00000000000000000, 5.571627607371296764E-15 ) ) ;
#14234=CARTESIAN_POINT ( 'NONE',  ( 44.50160557815096496, 40.00000000000000000, -5.869829666507492050 ) ) ;
#14236=CARTESIAN_POINT ( 'NONE',  ( -45.80426865613544862, 40.00000000000000000, -26.55377233850569141 ) ) ;
#14244=CARTESIAN_POINT ( 'NONE',  ( -14.19360040536685830, 40.00000000000000000, 24.59234967646941783 ) ) ;
#14261=CARTESIAN_POINT ( 'NONE',  ( 39.32569335900156204, 31.00000000000000355, 68.32161714268157482 ) ) ;
#14268=CARTESIAN_POINT ( 'NONE',  ( 93.52153384685561832, 39.99999999999999289, -24.92737483788710762 ) ) ;
#14280=CARTESIAN_POINT ( 'NONE',  ( -58.57471716409879292, 31.00000000000000711, 66.78942258476980953 ) ) ;
#14282=ORIENTED_EDGE ( 'NONE', *, *, #22573, .F. ) ;
#14283=ADVANCED_FACE ( 'NONE', ( #14895 ), #28195, .F. ) ;
#14284=CARTESIAN_POINT ( 'NONE',  ( 26.10672890669277990, 40.00000000000000000, 8.893381768402427667 ) ) ;
#14289=CARTESIAN_POINT ( 'NONE',  ( -61.42214656768812375, 31.00000000000000711, 79.86467493626638259 ) ) ;
#14312=CARTESIAN_POINT ( 'NONE',  ( -32.45554871466278968, 31.00000000000000355, -28.56710966684966380 ) ) ;
#14320=CARTESIAN_POINT ( 'NONE',  ( 49.67886955981430219, 40.00000000000000000, -43.43868092391004865 ) ) ;
#14333=CARTESIAN_POINT ( 'NONE',  ( 23.58227068755204314, 31.00000000000000355, -47.84673847638903510 ) ) ;
#14341=CARTESIAN_POINT ( 'NONE',  ( 25.10416666396844576, 40.00000000000000000, 1.636246165087044124 ) ) ;
#14347=CARTESIAN_POINT ( 'NONE',  ( 33.43413415811954081, 31.00000000000000355, -67.56680175473152872 ) ) ;
#14349=CARTESIAN_POINT ( 'NONE',  ( 9.885896071376818028, 40.00000000000000000, -74.20985814143865866 ) ) ;
#14362=CARTESIAN_POINT ( 'NONE',  ( -12.78314611188302052, 40.00000000000000000, 97.07982689498881257 ) ) ;
#14374=CARTESIAN_POINT ( 'NONE',  ( -20.28213647683248766, 40.00000000000000000, 23.06128528321566051 ) ) ;
#14376=DIRECTION ( 'NONE',  ( 0.000000000000000000, 1.000000000000000000, -1.060184893785364939E-15 ) ) ;
#14391=CARTESIAN_POINT ( 'NONE',  ( 25.04716826810500763, 31.00000000000000355, 3.293035637142270655 ) ) ;
#14397=CARTESIAN_POINT ( 'NONE',  ( 66.75212336275305347, 31.00000000000000000, -51.21939497476837744 ) ) ;
#14401=CARTESIAN_POINT ( 'NONE',  ( -41.92568936860566708, 31.00000000000000355, -5.596851440150872214 ) ) ;
#14403=CARTESIAN_POINT ( 'NONE',  ( -49.69442049507403425, 40.00000000000000000, -64.76435429890716478 ) ) ;
#14417=CARTESIAN_POINT ( 'NONE',  ( 34.44467569804516671, 40.00000000000000000, 44.88666365967159777 ) ) ;
#14452=CARTESIAN_POINT ( 'NONE',  ( 27.23661496637203427, 31.00000000000000355, 23.88131275951389654 ) ) ;
#14461=CARTESIAN_POINT ( 'NONE',  ( -15.46676570949300000, 40.00000000000000000, 45.57083133015776610 ) ) ;
#14462=CARTESIAN_POINT ( 'NONE',  ( -51.85848278221650531, 40.00000000000000000, -6.921372802089502230 ) ) ;
#14471=CARTESIAN_POINT ( 'NONE',  ( 25.04716826810500763, 40.00000000000000000, 3.293035637142270655 ) ) ;
#14487=CARTESIAN_POINT ( 'NONE',  ( -56.48168293059611500, 31.00000000000000711, 43.19841958068096233 ) ) ;
#14496=CARTESIAN_POINT ( 'NONE',  ( -45.36921519482122989, 40.00000000000000711, 78.33339762292068542 ) ) ;
#14509=CARTESIAN_POINT ( 'NONE',  ( 11.43299787627070607, 31.00000000000000355, 86.72764684403134083 ) ) ;
#14513=CARTESIAN_POINT ( 'NONE',  ( 12.70938237924789860, 40.00000000000000000, -21.97768283340562689 ) ) ;
#14543=CARTESIAN_POINT ( 'NONE',  ( -2.659806967433831382, 31.00000000000000355, 39.59793253467758944 ) ) ;
#14550=CARTESIAN_POINT ( 'NONE',  ( 67.09393615765254992, 39.99999999999999289, 4.495243625008655819 ) ) ;
#14561=CARTESIAN_POINT ( 'NONE',  ( 44.56294422764113250, 31.00000000000000355, 34.17917587534974189 ) ) ;
#14570=CARTESIAN_POINT ( 'NONE',  ( -29.59829689555773058, 40.00000000000000000, 3.906358533625565954 ) ) ;
#14574=CARTESIAN_POINT ( 'NONE',  ( -29.11455967534192979, 31.00000000000000355, 85.38284731564058916 ) ) ;
#14575=CARTESIAN_POINT ( 'NONE',  ( -72.38966680857410552, 40.00000000000000711, 55.38960906678870799 ) ) ;
#14589=CARTESIAN_POINT ( 'NONE',  ( -89.22528799552154055, 40.00000000000000711, 43.99828826784794700 ) ) ;
#14597=DIRECTION ( 'NONE',  ( 0.000000000000000000, 0.000000000000000000, 1.000000000000000000 ) ) ;
#14604=CARTESIAN_POINT ( 'NONE',  ( 36.56095242094649933, 40.00000000000000000, -4.755136101395176951 ) ) ;
#14616=CARTESIAN_POINT ( 'NONE',  ( -15.87544005811639458, 31.00000000000000355, -27.47754625559162989 ) ) ;
#14621=CARTESIAN_POINT ( 'NONE',  ( -40.93297376624923345, 31.00000000000000355, -70.86912620794510076 ) ) ;
#14625=CARTESIAN_POINT ( 'NONE',  ( -26.81486728382429519, 31.00000000000000355, -46.61672233255472975 ) ) ;
#14626=CARTESIAN_POINT ( 'NONE',  ( -78.83182461418512332, 40.00000000000000711, -45.51551753872077910 ) ) ;
#14640=CARTESIAN_POINT ( 'NONE',  ( -57.43240763726046794, 40.00000000000000000, -19.49446143887317717 ) ) ;
#14650=VECTOR ( 'NONE', #36128, 1000.000000000000000 ) ;
#14654=CARTESIAN_POINT ( 'NONE',  ( -76.05825820879897492, 31.00000000000000711, 66.55365856249082412 ) ) ;
#14668=CARTESIAN_POINT ( 'NONE',  ( 35.44578089419255917, 31.00000000000000355, -40.42088417236866604 ) ) ;
#14675=CARTESIAN_POINT ( 'NONE',  ( -48.80550277073417931, 40.00000000000000000, -13.06547612810710035 ) ) ;
#14676=CARTESIAN_POINT ( 'NONE',  ( -7.015336270754768400, 40.00000000000000000, -53.95087245962636047 ) ) ;
#14688=CARTESIAN_POINT ( 'NONE',  ( -15.87544005811639458, 40.00000000000000000, -27.47754625559162989 ) ) ;
#14702=CARTESIAN_POINT ( 'NONE',  ( -44.72205690102930475, 31.00000000000000355, -58.47036224961646411 ) ) ;
#14711=CARTESIAN_POINT ( 'NONE',  ( -40.08783408682389648, 40.00000000000000000, 81.04563091341927361 ) ) ;
#14714=CARTESIAN_POINT ( 'NONE',  ( 27.10182830755124428, 31.00000000000000355, 1.799748011963437033 ) ) ;
#14726=CARTESIAN_POINT ( 'NONE',  ( 12.74197863150380883, 31.00000000000000355, 96.66318596537892915 ) ) ;
#14729=CARTESIAN_POINT ( 'NONE',  ( 20.65150112226537260, 40.00000000000000000, -15.81946110361252877 ) ) ;
#14757=VERTEX_POINT ( 'NONE', #2499 ) ;
#14759=CARTESIAN_POINT ( 'NONE',  ( -41.03896728213481992, 31.00000000000000355, -11.06873348903806864 ) ) ;
#14765=CARTESIAN_POINT ( 'NONE',  ( -53.12901929299007975, 40.00000000000000000, 30.56653509229933263 ) ) ;
#14778=CARTESIAN_POINT ( 'NONE',  ( -19.97695672607123640, 31.00000000000000355, -58.81104016858105155 ) ) ;
#14787=CARTESIAN_POINT ( 'NONE',  ( 78.79907178683629354, 31.00000000000000000, 38.97904116289377185 ) ) ;
#14788=CARTESIAN_POINT ( 'NONE',  ( -91.21105805184879500, 40.00000000000000711, 11.89862498596346718 ) ) ;
#14791=EDGE_LOOP ( 'NONE', ( #34249, #39366, #27113, #21073 ) ) ;
#14802=CARTESIAN_POINT ( 'NONE',  ( -40.67465422008825726, 40.00000000000000000, -82.48404079236435393 ) ) ;
#14817=CARTESIAN_POINT ( 'NONE',  ( 9.106956811744730373, 40.00000000000000000, -33.78410985268681799 ) ) ;
#14828=CARTESIAN_POINT ( 'NONE',  ( 23.79574588541966662, 31.00000000000000355, -6.380716493563439506 ) ) ;
#14835=CARTESIAN_POINT ( 'NONE',  ( -47.90394619311608437, 31.00000000000000355, 62.45286580340285099 ) ) ;
#14838=CARTESIAN_POINT ( 'NONE',  ( 24.55685208794459129, 31.00000000000000355, -49.59815698162134368 ) ) ;
#14840=CARTESIAN_POINT ( 'NONE',  ( 84.73112319332513209, 39.99999999999999289, -41.78253223598262167 ) ) ;
#14853=CARTESIAN_POINT ( 'NONE',  ( 62.51641183113888900, 39.99999999999999289, -16.75201923384928548 ) ) ;
#14885=CARTESIAN_POINT ( 'NONE',  ( 17.07784400123870938, 31.00000000000000355, -50.31546185293520779 ) ) ;
#14892=CARTESIAN_POINT ( 'NONE',  ( -60.10416666555506993, 40.00000000000000711, -3.926990808566252156 ) ) ;
#14893=CARTESIAN_POINT ( 'NONE',  ( 7.251580242022520828, 40.00000000000000000, -54.34182998362662431 ) ) ;
#14895=FACE_OUTER_BOUND ( 'NONE', #32661, .T. ) ;
#14902=CARTESIAN_POINT ( 'NONE',  ( 34.56606645648713538, 40.00000000000000000, -4.560848911255810378 ) ) ;
#14917=CARTESIAN_POINT ( 'NONE',  ( 22.12550800842194931, 31.00000000000000355, 65.48657384636695156 ) ) ;
#14927=CARTESIAN_POINT ( 'NONE',  ( -5.980347265640406640, 40.00000000000000000, 89.59238221261722401 ) ) ;
#14928=CARTESIAN_POINT ( 'NONE',  ( 12.72035051019680729, 31.00000000000000355, 25.87482915247129611 ) ) ;
#14946=CARTESIAN_POINT ( 'NONE',  ( -1.587008504153756938, 40.00000000000000000, -24.39691638390478090 ) ) ;
#14973=CARTESIAN_POINT ( 'NONE',  ( -32.60815990948594134, 31.00000000000000355, 24.92795611697640368 ) ) ;
#14981=CARTESIAN_POINT ( 'NONE',  ( -31.81746463534672387, 40.00000000000000000, -55.29958784370776925 ) ) ;
#14988=CARTESIAN_POINT ( 'NONE',  ( -15.99999999999997691, 31.00000000000000711, 4.500000000000005329 ) ) ;
#14994=CARTESIAN_POINT ( 'NONE',  ( -63.57631528421845957, 31.00000000000000711, -31.33741679916209222 ) ) ;
#15004=CARTESIAN_POINT ( 'NONE',  ( 84.58694138809386232, 31.00000000000000000, 22.77597867319729374 ) ) ;
#15005=CARTESIAN_POINT ( 'NONE',  ( 86.90011881125597881, 39.99999999999999289, -5.573058087428396590 ) ) ;
#15017=PLANE ( 'NONE',  #31685 ) ;
#15021=CARTESIAN_POINT ( 'NONE',  ( 92.36625196220676060, 39.99999999999999289, 24.73319171124347093 ) ) ;
#15032=DIRECTION ( 'NONE',  ( 0.000000000000000000, 1.000000000000000000, 0.000000000000000000 ) ) ;
#15033=CARTESIAN_POINT ( 'NONE',  ( -31.59164309906362078, 40.00000000000000000, 4.115917706318550806 ) ) ;
#15049=CARTESIAN_POINT ( 'NONE',  ( 28.66079171547214699, 31.00000000000000355, 21.97938003711830035 ) ) ;
#15057=CARTESIAN_POINT ( 'NONE',  ( -20.19574676229028043, 31.00000000000000355, 75.42596061005518493 ) ) ;
#15060=CARTESIAN_POINT ( 'NONE',  ( -32.53655534684842365, 31.00000000000000355, -42.55839752837237455 ) ) ;
#15061=CARTESIAN_POINT ( 'NONE',  ( -60.37409795221152109, 40.00000000000000711, -68.82020352599361956 ) ) ;
#15074=CARTESIAN_POINT ( 'NONE',  ( -48.53848235557606472, 40.00000000000000000, -37.22912483484027035 ) ) ;
#15107=DIRECTION ( 'NONE',  ( 0.000000000000000000, 1.000000000000000000, 0.000000000000000000 ) ) ;
#15108=CARTESIAN_POINT ( 'NONE',  ( -22.94860596549062848, 31.00000000000000355, -46.53072237555588231 ) ) ;
#15117=CARTESIAN_POINT ( 'NONE',  ( -59.40491426035100631, 40.00000000000000711, 7.833300799371349932 ) ) ;
#15118=CARTESIAN_POINT ( 'NONE',  ( -9.228224334387265415, 40.00000000000000000, 69.24269282083176336 ) ) ;
#15119=CARTESIAN_POINT ( 'NONE',  ( -15.99999999999997691, 17.11489954122026447, 5.571627607371296764E-15 ) ) ;
#15123=CARTESIAN_POINT ( 'NONE',  ( 24.63052733448982323, 31.00000000000000355, -3.251868155982907904 ) ) ;
#15125=CARTESIAN_POINT ( 'NONE',  ( 32.71557229150619861, 40.00000000000000000, -11.11602612089219910 ) ) ;
#15143=AXIS2_PLACEMENT_3D ( 'NONE', #16886, #10967, #33633 ) ;
#15145=CARTESIAN_POINT ( 'NONE',  ( 66.32976035609178211, 31.00000000000000000, 58.33333674018341952 ) ) ;
#15155=CARTESIAN_POINT ( 'NONE',  ( 11.19416946702030735, 31.00000000000000355, -22.66942529387728555 ) ) ;
#15170=CARTESIAN_POINT ( 'NONE',  ( 7.507699080470448649, 40.00000000000000000, 28.16210111025598906 ) ) ;
#15203=CARTESIAN_POINT ( 'NONE',  ( -23.74678488967455436, 31.00000000000000355, -48.36925102894097961 ) ) ;
#15214=CARTESIAN_POINT ( 'NONE',  ( -48.39074809477736494, 40.00000000000000000, -55.33250407649475733 ) ) ;
#15226=CARTESIAN_POINT ( 'NONE',  ( 57.13603463884887645, 31.00000000000000355, 32.98675068510902264 ) ) ;
#15235=CARTESIAN_POINT ( 'NONE',  ( 83.84057477258951963, 31.00000000000000000, -22.33845567675551180 ) ) ;
#15236=CARTESIAN_POINT ( 'NONE',  ( -65.95487968126425926, 40.00000000000000711, -50.74205456615700882 ) ) ;
#15267=CARTESIAN_POINT ( 'NONE',  ( 32.80084743084300669, 40.00000000000000000, 19.01436317119532760 ) ) ;
#15281=CARTESIAN_POINT ( 'NONE',  ( 18.38119342899891961, 31.00000000000000355, 31.81670425098764099 ) ) ;
#15282=VERTEX_POINT ( 'NONE', #2441 ) ;
#15284=CARTESIAN_POINT ( 'NONE',  ( -21.28946418274055929, 31.00000000000000355, -79.45670318283352174 ) ) ;
#15286=CARTESIAN_POINT ( 'NONE',  ( -51.85848278221650531, 31.00000000000000355, -6.921372802086644072 ) ) ;
#15287=CARTESIAN_POINT ( 'NONE',  ( -40.67465422008825726, 40.00000000000000000, -82.48404079236435393 ) ) ;
#15302=CARTESIAN_POINT ( 'NONE',  ( -54.82550897924149069, 40.00000000000000711, 42.06954809655981364 ) ) ;
#15306=DIRECTION ( 'NONE',  ( -0.06345332152672161774, 1.058048417131579272E-15, 0.9979848074931934043 ) ) ;
#15311=LINE ( 'NONE', #39659, #17753 ) ;
#15327=CARTESIAN_POINT ( 'NONE',  ( -6.238242335983215092, 31.00000000000000355, 47.40213128959678102 ) ) ;
#15334=CARTESIAN_POINT ( 'NONE',  ( 42.30435120181500963, 40.00000000000000000, 37.09784777058769123 ) ) ;
#15341=CARTESIAN_POINT ( 'NONE',  ( -19.20510714644778361, 40.00000000000000000, 33.27066566623395261 ) ) ;
#15355=CARTESIAN_POINT ( 'NONE',  ( -35.65230965298280097, 31.00000000000000355, 72.05959145978816593 ) ) ;
#15357=VERTEX_POINT ( 'NONE', #9441 ) ;
#15363=CARTESIAN_POINT ( 'NONE',  ( 26.62151981922249533, 31.00000000000000355, -3.482817046706074393 ) ) ;
#15375=CARTESIAN_POINT ( 'NONE',  ( 29.96647033545507455, 31.00000000000000355, -88.27250603610892199 ) ) ;
#15382=CARTESIAN_POINT ( 'NONE',  ( 32.71557229150619861, 40.00000000000000000, -11.11602612089219910 ) ) ;
#15383=CARTESIAN_POINT ( 'NONE',  ( -41.89947471387619515, 40.00000000000000000, 2.670153906482984230 ) ) ;
#15409=CARTESIAN_POINT ( 'NONE',  ( -51.85848278221650531, 31.00000000000000355, -6.921372802086644072 ) ) ;
#15417=CARTESIAN_POINT ( 'NONE',  ( 33.43413415811954792, 40.00000000000000000, -67.56680175473154293 ) ) ;
#15427=CARTESIAN_POINT ( 'NONE',  ( 52.51402048354923835, 31.00000000000000355, 40.27907379435107060 ) ) ;
#15440=CARTESIAN_POINT ( 'NONE',  ( 68.41293481155882716, 31.00000000000000000, -52.34142988146868447 ) ) ;
#15441=CARTESIAN_POINT ( 'NONE',  ( 52.26791824981292933, 40.00000000000000000, -67.94187691988643962 ) ) ;
#15466=CARTESIAN_POINT ( 'NONE',  ( -28.59133019391067165, 40.00000000000000000, -32.71076623427350683 ) ) ;
#15478=CARTESIAN_POINT ( 'NONE',  ( -39.53383601736616271, 31.00000000000000355, 5.215339288884301538 ) ) ;
#15485=EDGE_CURVE ( 'NONE', #6578, #36284, #36260, .T. ) ;
#15487=CARTESIAN_POINT ( 'NONE',  ( -40.67465422008825726, 31.00000000000000355, -82.48404079236435393 ) ) ;
#15489=CARTESIAN_POINT ( 'NONE',  ( -49.80813925210023996, 31.00000000000000355, -17.00652635548579994 ) ) ;
#15490=CARTESIAN_POINT ( 'NONE',  ( 84.24376206367318787, 39.99999999999999289, -11.10575268747775901 ) ) ;
#15503=CARTESIAN_POINT ( 'NONE',  ( -21.91107887650263564, 40.00000000000000000, 64.54935342160338507 ) ) ;
#15530=CARTESIAN_POINT ( 'NONE',  ( 20.73284993368543638, 31.00000000000000355, 42.03655757353646294 ) ) ;
#15536=CARTESIAN_POINT ( 'NONE',  ( 48.10206620145878276, 40.00000000000000000, -42.20136231105875879 ) ) ;
#15545=CARTESIAN_POINT ( 'NONE',  ( 26.99674208481366833, 40.00000000000000000, -20.71990538090019029 ) ) ;
#15558=CARTESIAN_POINT ( 'NONE',  ( -10.92011822083620309, 31.00000000000000355, -83.75917815547792600 ) ) ;
#15566=CARTESIAN_POINT ( 'NONE',  ( -76.05825820879898913, 40.00000000000000711, 66.55365856249082412 ) ) ;
#15580=CARTESIAN_POINT ( 'NONE',  ( 11.86982580658625075, 40.00000000000000000, 24.05989836594520526 ) ) ;
#15581=CARTESIAN_POINT ( 'NONE',  ( -24.78443185004241656, 40.00000000000000000, 32.19086620116434005 ) ) ;
#15606=CARTESIAN_POINT ( 'NONE',  ( -16.19793102917653371, 31.00000000000000355, 47.43702525407732651 ) ) ;
#15613=CARTESIAN_POINT ( 'NONE',  ( 76.69346925290108175, 39.99999999999999289, 10.21457306974340007 ) ) ;
#15624=CARTESIAN_POINT ( 'NONE',  ( -4.417864660710832503, 31.00000000000000355, 67.60416666563759236 ) ) ;
#15636=CARTESIAN_POINT ( 'NONE',  ( -6.060882879309181348, 31.00000000000000355, -94.40013096059719544 ) ) ;
#15637=CARTESIAN_POINT ( 'NONE',  ( -32.34013556242301490, 40.00000000000000000, 94.87070470178476000 ) ) ;
#15639=EDGE_CURVE ( 'NONE', #39440, #6140, #24318, .T. ) ;
#15662=EDGE_CURVE ( 'NONE', #42412, #42546, #31039, .T. ) ;
#15670=CARTESIAN_POINT ( 'NONE',  ( 5.928665350384931365, 40.00000000000000000, -44.40877992885556580 ) ) ;
#15680=CARTESIAN_POINT ( 'NONE',  ( -39.89583333501392559, 31.00000000000000355, 2.617993869485681468 ) ) ;
#15688=CARTESIAN_POINT ( 'NONE',  ( 57.05379307149791401, 31.00000000000000000, -74.37948018729004218 ) ) ;
#15693=CARTESIAN_POINT ( 'NONE',  ( 65.23019871247133494, 31.00000000000000000, 17.57949444736449252 ) ) ;
#15707=CARTESIAN_POINT ( 'NONE',  ( -53.60515337853228601, 40.00000000000000000, -47.01024902908782366 ) ) ;
#15735=CARTESIAN_POINT ( 'NONE',  ( 52.68777711438346500, 31.00000000000000355, 17.88338314711659294 ) ) ;
#15743=CARTESIAN_POINT ( 'NONE',  ( -17.60292107714122878, 40.00000000000000000, 65.74579412301164894 ) ) ;
#15755=CARTESIAN_POINT ( 'NONE',  ( -49.46937513889707105, 40.00000000000000000, 6.524320044134898744 ) ) ;
#15766=CARTESIAN_POINT ( 'NONE',  ( 10.26812810425290579, 31.00000000000000355, 78.79123036457541218 ) ) ;
#15775=CARTESIAN_POINT ( 'NONE',  ( -98.36195137680903144, 40.00000000000000711, 26.22212808230024805 ) ) ;
#15787=CARTESIAN_POINT ( 'NONE',  ( 34.56606645648713538, 31.00000000000000355, -4.560848911255810378 ) ) ;
#15792=CARTESIAN_POINT ( 'NONE',  ( -30.01493782828161017, 40.00000000000000000, -3.947526014606304035 ) ) ;
#15793=CARTESIAN_POINT ( 'NONE',  ( -16.82630558382439290, 40.00000000000000000, -29.24196894321155682 ) ) ;
#15815=CARTESIAN_POINT ( 'NONE',  ( 61.87885091699251916, 39.99999999999999289, -70.55635664373320992 ) ) ;
#15818=DIRECTION ( 'NONE',  ( 0.000000000000000000, 1.000000000000000000, -1.060184893785364939E-15 ) ) ;
#15823=CARTESIAN_POINT ( 'NONE',  ( 6.367266499441480043, 31.00000000000000355, 48.98256792610027333 ) ) ;
#15829=ORIENTED_EDGE ( 'NONE', *, *, #36398, .F. ) ;
#15830=CARTESIAN_POINT ( 'NONE',  ( 61.98103557012430542, 39.99999999999999289, 47.69015029125304039 ) ) ;
#15833=CARTESIAN_POINT ( 'NONE',  ( -17.44537629401976631, 31.00000000000000000, -4.261559264950514958 ) ) ;
#15837=CARTESIAN_POINT ( 'NONE',  ( -105.9879088449591933, 17.11489954122026447, -0.3807199291576673361 ) ) ;
#15843=CARTESIAN_POINT ( 'NONE',  ( 8.815036365794538753, 31.00000000000000355, 66.85656860134390911 ) ) ;
#15858=CARTESIAN_POINT ( 'NONE',  ( -91.59543978412355614, 31.00000000000000711, -12.18496625896582231 ) ) ;
#15859=CARTESIAN_POINT ( 'NONE',  ( 31.77777543000702565, 40.00000000000000000, 93.95825142774114624 ) ) ;
#15883=CARTESIAN_POINT ( 'NONE',  ( -105.9879088449591933, 40.00000000000000000, -0.3807199291576673361 ) ) ;
#15884=ORIENTED_EDGE ( 'NONE', *, *, #21035, .F. ) ;
#15888=CARTESIAN_POINT ( 'NONE',  ( 46.89194940766294906, 40.00000000000000000, 6.259973086888630078 ) ) ;
#15900=CARTESIAN_POINT ( 'NONE',  ( 34.89583333524210218, 31.00000000000000355, -2.290744634698907767 ) ) ;
#15907=CARTESIAN_POINT ( 'NONE',  ( -11.47416535668642723, 31.00000000000000355, 87.14428777381637303 ) ) ;
#15914=CARTESIAN_POINT ( 'NONE',  ( -59.29355402628473115, 31.00000000000000355, -20.23837177251482800 ) ) ;
#15916=CARTESIAN_POINT ( 'NONE',  ( -53.44803860755722269, 40.00000000000000000, 46.73995993581220176 ) ) ;
#15927=CARTESIAN_POINT ( 'NONE',  ( -23.19911330973958030, 40.00000000000000000, -68.30030121463531145 ) ) ;
#15957=CARTESIAN_POINT ( 'NONE',  ( 42.05404839982585941, 31.00000000000000355, -47.95475229022623864 ) ) ;
#15964=CARTESIAN_POINT ( 'NONE',  ( -31.99444157862340532, 31.00000000000000355, -4.262017635501121227 ) ) ;
#15967=CARTESIAN_POINT ( 'NONE',  ( 4.745113895470035814, 40.00000000000000000, -72.60416666572081112 ) ) ;
#15974=CARTESIAN_POINT ( 'NONE',  ( -32.14164714139042189, 40.00000000000000000, 36.65395011347077059 ) ) ;
#15985=CARTESIAN_POINT ( 'NONE',  ( -71.82650799747224823, 31.00000000000000711, -41.60779115368423220 ) ) ;
#15986=EDGE_LOOP ( 'NONE', ( #10519, #22040, #41423, #3032 ) ) ;
#15996=CARTESIAN_POINT ( 'NONE',  ( -101.9959696149863788, 40.00000000000000711, -0.1269066430510139010 ) ) ;
#16002=CARTESIAN_POINT ( 'NONE',  ( -14.19360040536685830, 31.00000000000000355, 24.59234967646941783 ) ) ;
#16009=CARTESIAN_POINT ( 'NONE',  ( -4.929261580875707871, 40.00000000000000000, 37.46659216873931797 ) ) ;
#16010=CARTESIAN_POINT ( 'NONE',  ( 23.59836588144746017, 40.00000000000000000, -26.81698947917456621 ) ) ;
#16038=CARTESIAN_POINT ( 'NONE',  ( 15.70068437845899290, 31.00000000000000355, 46.50252577710988078 ) ) ;
#16044=CARTESIAN_POINT ( 'NONE',  ( -4.761419979751499554, 40.00000000000000000, -74.40007767863900767 ) ) ;
#16056=CARTESIAN_POINT ( 'NONE',  ( 65.81435062899562638, 31.00000000000000000, 37.99825742654716976 ) ) ;
#16065=CARTESIAN_POINT ( 'NONE',  ( -80.50242771303932443, 31.00000000000000711, -46.62292012068298419 ) ) ;
#16066=CARTESIAN_POINT ( 'NONE',  ( -6.638544827991895048, 40.00000000000000000, 99.59190654106264162 ) ) ;
#16074=FACE_OUTER_BOUND ( 'NONE', #28252, .T. ) ;
#16078=CARTESIAN_POINT ( 'NONE',  ( -105.0363123600777442, 31.00000000000000355, -2.692529638013756443 ) ) ;
#16087=CARTESIAN_POINT ( 'NONE',  ( -11.85532105537472525, 31.00000000000000355, -20.54123584193516550 ) ) ;
#16096=CARTESIAN_POINT ( 'NONE',  ( -39.38196478160931946, 40.00000000000000000, 13.29643045357694753 ) ) ;
#16109=CARTESIAN_POINT ( 'NONE',  ( -38.53741714288415210, 31.00000000000000355, -33.79371401777069650 ) ) ;
#16114=CARTESIAN_POINT ( 'NONE',  ( 41.30831894254264824, 31.00000000000000355, -83.80005689411834169 ) ) ;
#16118=CARTESIAN_POINT ( 'NONE',  ( 17.81064159971323946, 31.00000000000000355, 66.89829513328324140 ) ) ;
#16119=CARTESIAN_POINT ( 'NONE',  ( -69.31868535678037802, 40.00000000000000711, 18.45717643660483986 ) ) ;
#16120=CARTESIAN_POINT ( 'NONE',  ( -25.38139813252123034, 40.00000000000000000, 94.78629358389331117 ) ) ;
#16124=DIRECTION ( 'NONE',  ( 0.000000000000000000, -1.000000000000000000, 5.297542245118643184E-16 ) ) ;
#16125=DIRECTION ( 'NONE',  ( 0.3211947320043982423, 1.004009057038134257E-15, 0.9470131699890044219 ) ) ;
#16131=CARTESIAN_POINT ( 'NONE',  ( 23.52215716829092074, 40.00000000000000000, -69.29398394448777765 ) ) ;
#16161=CARTESIAN_POINT ( 'NONE',  ( -25.79802671946675474, 31.00000000000000355, 52.34090327860478453 ) ) ;
#16167=CARTESIAN_POINT ( 'NONE',  ( 11.33656872182281816, 31.00000000000000355, -33.21392199183605243 ) ) ;
#16169=CARTESIAN_POINT ( 'NONE',  ( 55.63593431945896839, 39.99999999999999289, -48.80962981700470493 ) ) ;
#16179=CARTESIAN_POINT ( 'NONE',  ( -36.61132647064156487, 40.00000000000000000, -18.04288060775211378 ) ) ;
#16181=FACE_OUTER_BOUND ( 'NONE', #36526, .T. ) ;
#16192=CARTESIAN_POINT ( 'NONE',  ( -6.060882879309181348, 31.00000000000000355, -94.40013096059719544 ) ) ;
#16210=CARTESIAN_POINT ( 'NONE',  ( -29.89583333557403222, 31.00000000000000355, 1.963495399902740690 ) ) ;
#16216=CARTESIAN_POINT ( 'NONE',  ( 26.55430347651023837, 40.00000000000000000, -34.62409890758566178 ) ) ;
#16217=CARTESIAN_POINT ( 'NONE',  ( -22.00208165626150603, 40.00000000000000000, -25.16137218361809857 ) ) ;
#16246=CARTESIAN_POINT ( 'NONE',  ( 45.08926718328532246, 31.00000000000000355, 51.56349680124436219 ) ) ;
#16256=CARTESIAN_POINT ( 'NONE',  ( -54.99468034528496929, 40.00000000000000000, -62.86974495748533087 ) ) ;
#16267=EDGE_CURVE ( 'NONE', #41658, #25259, #11807, .T. ) ;
#16268=CARTESIAN_POINT ( 'NONE',  ( -77.84600223180727596, 31.00000000000000711, -20.84395318355897686 ) ) ;
#16275=CARTESIAN_POINT ( 'NONE',  ( -82.08563009789774867, 31.00000000000000711, 40.34115885382633593 ) ) ;
#16276=CARTESIAN_POINT ( 'NONE',  ( 96.56285295106285105, 39.99999999999999289, 12.84127866192819312 ) ) ;
#16294=CARTESIAN_POINT ( 'NONE',  ( 22.71825314374493487, 31.00000000000000355, -13.09499307598873585 ) ) ;
#16303=CARTESIAN_POINT ( 'NONE',  ( -5.720710522143956034, 40.00000000000000000, -44.01410879001467436 ) ) ;
#16305=VECTOR ( 'NONE', #21078, 999.9999999999998863 ) ;
#16316=CARTESIAN_POINT ( 'NONE',  ( -38.92335646797288717, 31.00000000000000355, 29.86975225897632313 ) ) ;
#16320=CARTESIAN_POINT ( 'NONE',  ( 82.68608547523962216, 31.00000000000000000, 22.14036602612658200 ) ) ;
#16324=CARTESIAN_POINT ( 'NONE',  ( -18.22940504111061344, 31.00000000000000355, 67.64968002090884625 ) ) ;
#16325=CARTESIAN_POINT ( 'NONE',  ( 17.81064159970942384, 40.00000000000000000, 66.89829513328324140 ) ) ;
#16326=CARTESIAN_POINT ( 'NONE',  ( -78.67873774631718220, 40.00000000000000711, 60.36924185307643143 ) ) ;
#16340=CARTESIAN_POINT ( 'NONE',  ( -25.13323546007955045, 40.00000000000000000, 74.03861446737784036 ) ) ;
#16343=CARTESIAN_POINT ( 'NONE',  ( -105.9879088449591933, 17.11489954122026447, -0.3807199291576673361 ) ) ;
#16375=CARTESIAN_POINT ( 'NONE',  ( -57.67632858778466698, 31.00000000000000711, 15.45560639130400205 ) ) ;
#16377=CARTESIAN_POINT ( 'NONE',  ( 2.511863649308172519, 31.00000000000000355, 39.39933062586388957 ) ) ;
#16378=CARTESIAN_POINT ( 'NONE',  ( -23.19911330973958030, 40.00000000000000000, -68.30030121463531145 ) ) ;
#16389=CARTESIAN_POINT ( 'NONE',  ( -21.36651465564686703, 40.00000000000000000, 43.35257367405362317 ) ) ;
#16406=CARTESIAN_POINT ( 'NONE',  ( -87.75478321338633236, 31.00000000000000711, -29.92102470462889130 ) ) ;
#16409=CARTESIAN_POINT ( 'NONE',  ( -15.99999999999997691, 17.11489954122026447, 5.571627607371296764E-15 ) ) ;
#16425=CARTESIAN_POINT ( 'NONE',  ( -15.87544005811639458, 31.00000000000000355, -27.47754625559162989 ) ) ;
#16433=CARTESIAN_POINT ( 'NONE',  ( -39.12533628356670334, 40.00000000000000000, -10.47265044290268499 ) ) ;
#16434=CARTESIAN_POINT ( 'NONE',  ( -5.720710522143956034, 40.00000000000000000, -44.01410879001467436 ) ) ;
#16446=VERTEX_POINT ( 'NONE', #3823 ) ;
#16465=CARTESIAN_POINT ( 'NONE',  ( 21.04585062970478759, 31.00000000000000355, -61.66509230325024049 ) ) ;
#16476=CARTESIAN_POINT ( 'NONE',  ( 78.79907178679739843, 39.99999999999999289, 38.97904116291323362 ) ) ;
#16487=CARTESIAN_POINT ( 'NONE',  ( -79.69263343296167079, 31.00000000000000711, -10.49242979028127820 ) ) ;
#16503=CARTESIAN_POINT ( 'NONE',  ( 76.36627019853398224, 31.00000000000000000, -58.43797548692494814 ) ) ;
#16523=CARTESIAN_POINT ( 'NONE',  ( -28.12618851199096781, 31.00000000000000355, 13.81902982503210708 ) ) ;
#16533=CARTESIAN_POINT ( 'NONE',  ( -45.80426865613544862, 40.00000000000000000, -26.55377233850569141 ) ) ;
#16547=CARTESIAN_POINT ( 'NONE',  ( -46.94946386092573221, 31.00000000000000355, 15.94926099647653928 ) ) ;
#16548=CARTESIAN_POINT ( 'NONE',  ( -99.91857577502598531, 40.00000000000000000, -1.280628618496984839 ) ) ;
#16553=CARTESIAN_POINT ( 'NONE',  ( -9.654069774896838041, 40.00000000000000000, -19.56573356436190636 ) ) ;
#16558=CARTESIAN_POINT ( 'NONE',  ( -31.81746463534672387, 31.00000000000000355, -55.29958784370775504 ) ) ;
#16559=CARTESIAN_POINT ( 'NONE',  ( 64.47787635702036368, 39.99999999999999289, -17.16423577040998438 ) ) ;
#16562=CARTESIAN_POINT ( 'NONE',  ( -99.99999999999997158, 40.00000000000000711, 2.428179185498535730E-12 ) ) ;
#16580=CARTESIAN_POINT ( 'NONE',  ( 48.66231590555653241, 39.99999999999999289, -55.48862040801123641 ) ) ;
#16592=CARTESIAN_POINT ( 'NONE',  ( -7.718844055051848230, 40.00000000000000000, -22.75659427661715384 ) ) ;
#16612=PRODUCT_CONTEXT ( 'NONE', #39502, 'mechanical' ) ;
#16614=CARTESIAN_POINT ( 'NONE',  ( 7.506055610550203205, 31.00000000000000355, 56.92102948000351148 ) ) ;
#16617=CARTESIAN_POINT ( 'NONE',  ( -16.82630558382797403, 31.00000000000000355, -29.24196894321154971 ) ) ;
#16619=CARTESIAN_POINT ( 'NONE',  ( 9.510694223897102617, 40.00000000000000000, -72.24097909213479340 ) ) ;
#16630=CARTESIAN_POINT ( 'NONE',  ( 39.78947517253659072, 40.00000000000000000, -19.62497191778171413 ) ) ;
#16645=CARTESIAN_POINT ( 'NONE',  ( 93.52153384689862037, 31.00000000000000000, -24.92737483788710406 ) ) ;
#16662=CARTESIAN_POINT ( 'NONE',  ( -18.92511213055653130, 31.00000000000000355, 21.58621387822740090 ) ) ;
#16668=CARTESIAN_POINT ( 'NONE',  ( 4.888094100070568437, 40.00000000000000000, 37.04995123692341252 ) ) ;
#16670=CARTESIAN_POINT ( 'NONE',  ( 36.21668514975058173, 40.00000000000000000, 31.87730689759005287 ) ) ;
#16697=CARTESIAN_POINT ( 'NONE',  ( -47.50570208456527155, 31.00000000000000355, -41.80188021843024160 ) ) ;
#16703=CARTESIAN_POINT ( 'NONE',  ( -73.09555549758189841, 40.00000000000000711, 35.91380138263622257 ) ) ;
#16713=CARTESIAN_POINT ( 'NONE',  ( 18.89933391970155085, 31.00000000000000355, -70.58587736658564893 ) ) ;
#16721=CARTESIAN_POINT ( 'NONE',  ( -22.10416666678001718, 40.00000000000000000, -1.441157586896875564 ) ) ;
#16725=CARTESIAN_POINT ( 'NONE',  ( -96.33078216555148288, 31.00000000000000711, 32.58251675337926656 ) ) ;
#16744=CARTESIAN_POINT ( 'NONE',  ( -18.66214908251421534, 31.00000000000000355, 24.25811346063288454 ) ) ;
#16749=ORIENTED_EDGE ( 'NONE', *, *, #38185, .F. ) ;
#16753=CARTESIAN_POINT ( 'NONE',  ( 57.09498703527649610, 40.00000000000000000, 3.831922229401318880 ) ) ;
#16758=CARTESIAN_POINT ( 'NONE',  ( -31.37281731866679024, 40.00000000000002842, 27.62913683693880174 ) ) ;
#16767=CARTESIAN_POINT ( 'NONE',  ( 26.55430347651023837, 31.00000000000000355, -34.62409890758566178 ) ) ;
#16772=CARTESIAN_POINT ( 'NONE',  ( -74.47060461443528823, 31.00000000000000711, 65.33029858165178894 ) ) ;
#16778=CARTESIAN_POINT ( 'NONE',  ( 9.885896071376816252, 31.00000000000000355, -74.20985814147174153 ) ) ;
#16779=CARTESIAN_POINT ( 'NONE',  ( -9.616483412535155040, 40.00000000000000000, -73.82325415887568454 ) ) ;
#16789=EDGE_LOOP ( 'NONE', ( #41836, #9650, #7610, #34032 ) ) ;
#16793=CARTESIAN_POINT ( 'NONE',  ( -79.69263343296167079, 40.00000000000000711, -10.49242979028127820 ) ) ;
#16805=CARTESIAN_POINT ( 'NONE',  ( -6.237032369604346371, 40.00000000000000000, -23.31551866006812901 ) ) ;
#16828=CARTESIAN_POINT ( 'NONE',  ( 74.30822294231431613, 31.00000000000000000, -9.796771932235298408 ) ) ;
#16831=CARTESIAN_POINT ( 'NONE',  ( 4.597210615069569961, 31.00000000000000355, -34.47704375836577384 ) ) ;
#16832=CARTESIAN_POINT ( 'NONE',  ( -26.42126989340051324, 40.00000000000000000, -77.78956226056263290 ) ) ;
#16845=CARTESIAN_POINT ( 'NONE',  ( 17.07784400123870938, 40.00000000000000000, -50.31546185293520779 ) ) ;
#16858=CARTESIAN_POINT ( 'NONE',  ( -70.09526419939506070, 31.00000000000000711, -61.63891210113990837 ) ) ;
#16875=CARTESIAN_POINT ( 'NONE',  ( -25.53337963587170023, 31.00000000000000355, 29.12008199578403023 ) ) ;
#16883=CARTESIAN_POINT ( 'NONE',  ( 13.85568741775851542, 40.00000000000000000, -40.82620080729295609 ) ) ;
#16884=CARTESIAN_POINT ( 'NONE',  ( 41.46880187714432253, 40.00000000000000000, 24.04226233541896107 ) ) ;
#16886=CARTESIAN_POINT ( 'NONE',  ( -15.99999999999997691, 31.00000000000000355, 5.571627607371296764E-15 ) ) ;
#16890=CARTESIAN_POINT ( 'NONE',  ( 23.79574588541966662, 40.00000000000000000, -6.380716493563439506 ) ) ;
#16892=LINE ( 'NONE', #19, #8309 ) ;
#16902=CARTESIAN_POINT ( 'NONE',  ( -100.0000000000000568, 40.00000000000000000, 2.687954026026062593E-12 ) ) ;
#16909=CARTESIAN_POINT ( 'NONE',  ( 54.03410584561684260, 31.00000000000000355, 41.58544482236945328 ) ) ;
#16916=CARTESIAN_POINT ( 'NONE',  ( 87.09251733236553150, 39.99999999999999289, 5.815661930448016825 ) ) ;
#16926=CARTESIAN_POINT ( 'NONE',  ( -28.35539204363714205, 31.00000000000000355, 83.52787551312086123 ) ) ;
#16954=CARTESIAN_POINT ( 'NONE',  ( -30.84436395684956977, 31.00000000000000355, -10.52363363425319243 ) ) ;
#16964=CARTESIAN_POINT ( 'NONE',  ( -47.35250803175856049, 40.00000000000000000, -23.44639516808875257 ) ) ;
#16975=CARTESIAN_POINT ( 'NONE',  ( 15.14372185054182651, 31.00000000000000355, 44.57714859939663654 ) ) ;
#16982=CARTESIAN_POINT ( 'NONE',  ( -43.52407497442469264, 31.00000000000000355, 88.29422169633753015 ) ) ;
#16985=CARTESIAN_POINT ( 'NONE',  ( 20.39742982868580157, 31.00000000000000355, 76.57971376064386959 ) ) ;
#16986=CARTESIAN_POINT ( 'NONE',  ( 39.32569335900156915, 40.00000000000000000, 68.32161714264680086 ) ) ;
#17000=ORIENTED_EDGE ( 'NONE', *, *, #28095, .T. ) ;
#17002=CARTESIAN_POINT ( 'NONE',  ( -77.84600223180727596, 40.00000000000000711, -20.84395318355897686 ) ) ;
#17014=CARTESIAN_POINT ( 'NONE',  ( 25.73918080462997082, 40.00000000000000000, -6.871072672212912735 ) ) ;
#17033=CARTESIAN_POINT ( 'NONE',  ( -69.75709431192164800, 31.00000000000000711, -9.183449035091399537 ) ) ;
#17036=CARTESIAN_POINT ( 'NONE',  ( -26.44890248586417414, 31.00000000000000355, -34.59877114778963403 ) ) ;
#17038=CARTESIAN_POINT ( 'NONE',  ( 74.30822294231431613, 39.99999999999999289, -9.796771932235298408 ) ) ;
#17050=CARTESIAN_POINT ( 'NONE',  ( -6.851565232941113415, 40.00000000000000000, -51.95325991929587417 ) ) ;
#17065=CARTESIAN_POINT ( 'NONE',  ( -91.59543978412355614, 31.00000000000000711, -12.18496625896582231 ) ) ;
#17083=CARTESIAN_POINT ( 'NONE',  ( -2.454369252093152376, 31.00000000000000355, 37.60416666486730009 ) ) ;
#17089=CARTESIAN_POINT ( 'NONE',  ( 40.56819808336118882, 40.00000000000000000, -35.59309480518532354 ) ) ;
#17091=CARTESIAN_POINT ( 'NONE',  ( -40.32452739091078797, 40.00000000000000000, -13.76986825753265720 ) ) ;
#17104=CARTESIAN_POINT ( 'NONE',  ( 1.472621547668719444, 40.00000000000000000, -22.60416666365413718 ) ) ;
#17120=CARTESIAN_POINT ( 'NONE',  ( -54.47698434024490410, 31.00000000000000355, -31.57393205620728693 ) ) ;
#17129=CARTESIAN_POINT ( 'NONE',  ( -26.95034633362163845, 40.00000000000000000, -79.72278128421112342 ) ) ;
#17130=AXIS2_PLACEMENT_3D ( 'NONE', #28144, #25532, #8922 ) ;
#17142=CARTESIAN_POINT ( 'NONE',  ( -90.10416666596678681, 31.00000000000000711, -5.890486217120279200 ) ) ;
#17150=CARTESIAN_POINT ( 'NONE',  ( -101.9001375416480499, 31.00000000000000711, 6.549163350515033954 ) ) ;
#17175=CARTESIAN_POINT ( 'NONE',  ( 32.62694724487210607, 31.00000000000000355, -16.02036196159510339 ) ) ;
#17181=DIRECTION ( 'NONE',  ( 0.000000000000000000, 1.541976423090494253E-15, 1.000000000000000000 ) ) ;
#17182=CARTESIAN_POINT ( 'NONE',  ( 43.74200748489512591, 40.00000000000000000, 38.49442098324160355 ) ) ;
#17197=CARTESIAN_POINT ( 'NONE',  ( 26.72236725836960147, 31.00000000000000355, -46.28813965123160301 ) ) ;
#17201=ORIENTED_EDGE ( 'NONE', *, *, #15662, .T. ) ;
#17205=CARTESIAN_POINT ( 'NONE',  ( -99.89583333318432778, 31.00000000000000711, 6.544984695199788760 ) ) ;
#17209=CARTESIAN_POINT ( 'NONE',  ( 58.79931003850258975, 31.00000000000000355, 51.72161244499935151 ) ) ;
#17210=CARTESIAN_POINT ( 'NONE',  ( -20.82795069772234342, 40.00000000000000000, 77.32795358076222669 ) ) ;
#17228=CARTESIAN_POINT ( 'NONE',  ( -80.10416666582359824, 40.00000000000000711, -5.235987747607834031 ) ) ;
#17242=CARTESIAN_POINT ( 'NONE',  ( 26.53203760875094019, 40.00000000000000000, 7.134992448515056651 ) ) ;
#17253=CARTESIAN_POINT ( 'NONE',  ( -27.62299686580952240, 31.00000000000000355, -13.61136854378590577 ) ) ;
#17263=CARTESIAN_POINT ( 'NONE',  ( 18.89933391970155085, 31.00000000000000355, -70.58587736658564893 ) ) ;
#17264=AXIS2_PLACEMENT_3D ( 'NONE', #15119, #4606, #37765 ) ;
#17265=CIRCLE ( 'NONE', #31872, 2.500000000000000444 ) ;
#17268=CARTESIAN_POINT ( 'NONE',  ( 3.148395399070833989, 31.00000000000000355, 49.39975974383467872 ) ) ;
#17269=CARTESIAN_POINT ( 'NONE',  ( -25.13323546007955045, 40.00000000000000000, 74.03861446737784036 ) ) ;
#17270=EDGE_CURVE ( 'NONE', #42546, #19619, #23476, .T. ) ;
#17280=CARTESIAN_POINT ( 'NONE',  ( 48.45771864870608425, 40.00000000000000000, 27.97524394371832202 ) ) ;
#17298=CARTESIAN_POINT ( 'NONE',  ( -26.02152878260477564, 31.00000000000000355, 96.68563202202810203 ) ) ;
#17316=CARTESIAN_POINT ( 'NONE',  ( 32.11716166826300167, 31.00000000000000355, 15.82712457579038912 ) ) ;
#17323=CARTESIAN_POINT ( 'NONE',  ( -49.46937513889707105, 40.00000000000000000, 6.524320044134898744 ) ) ;
#17325=CARTESIAN_POINT ( 'NONE',  ( -13.02511903071888533, 40.00000000000000000, 48.29538318457647961 ) ) ;
#17335=CARTESIAN_POINT ( 'NONE',  ( 2.965790448435745574, 40.00000000000000000, -22.56328348808469997 ) ) ;
#17336=ORIENTED_EDGE ( 'NONE', *, *, #10320, .T. ) ;
#17350=CARTESIAN_POINT ( 'NONE',  ( -23.73339997550686675, 31.00000000000000355, -70.23208777904191891 ) ) ;
#17355=DIRECTION ( 'NONE',  ( 0.000000000000000000, 1.000000000000000000, 0.000000000000000000 ) ) ;
#17357=CARTESIAN_POINT ( 'NONE',  ( 28.55926749299792178, 40.00000000000000000, 84.46800049165049984 ) ) ;
#17368=CARTESIAN_POINT ( 'NONE',  ( 38.45889818826288575, 31.00000000000000355, 77.98987599019784511 ) ) ;
#17375=DIRECTION ( 'NONE',  ( 0.000000000000000000, 1.000000000000000000, 0.000000000000000000 ) ) ;
#17397=CARTESIAN_POINT ( 'NONE',  ( -31.99444157862340532, 31.00000000000000355, -4.262017635501121227 ) ) ;
#17403=CARTESIAN_POINT ( 'NONE',  ( -30.89738163651703928, 40.00000000000000000, 40.13100860032159289 ) ) ;
#17415=CARTESIAN_POINT ( 'NONE',  ( -56.43872490705654599, 31.00000000000000711, 19.17141758013517716 ) ) ;
#17422=CARTESIAN_POINT ( 'NONE',  ( 31.25450476884064699, 31.00000000000000355, 92.02345382966369414 ) ) ;
#17428=CARTESIAN_POINT ( 'NONE',  ( -53.44803860757283331, 31.00000000000000355, 46.73995993579659114 ) ) ;
#17429=CARTESIAN_POINT ( 'NONE',  ( 47.76959191294547935, 40.00000000000000000, 62.44753968353898443 ) ) ;
#17444=CARTESIAN_POINT ( 'NONE',  ( -89.21153162435624040, 40.00000000000000711, 11.76024306507019901 ) ) ;
#17455=CARTESIAN_POINT ( 'NONE',  ( -10.52919346384764054, 40.00000000000000000, -21.36894910329525743 ) ) ;
#17468=CARTESIAN_POINT ( 'NONE',  ( 24.21999397792122366, 31.00000000000000355, 8.216913396989165008 ) ) ;
#17475=CARTESIAN_POINT ( 'NONE',  ( -30.22953878324074495, 31.00000000000000355, 61.32923288305941867 ) ) ;
#17477=CARTESIAN_POINT ( 'NONE',  ( 2.996940313443769099, 31.00000000000000355, -44.59688583547567475 ) ) ;
#17478=CARTESIAN_POINT ( 'NONE',  ( -51.96644965832453522, 40.00000000000000711, 59.25555446698126616 ) ) ;
#17488=CARTESIAN_POINT ( 'NONE',  ( 18.36587843422771016, 40.00000000000000000, 54.06640964556338957 ) ) ;
#17521=CARTESIAN_POINT ( 'NONE',  ( -35.44024466369167925, 31.00000000000000355, -20.45798383175513635 ) ) ;
#17522=AXIS2_PLACEMENT_3D ( 'NONE', #26539, #32649, #39607 ) ;
#17532=CARTESIAN_POINT ( 'NONE',  ( 44.89583333484414140, 40.00000000000000000, -2.945243104263157274 ) ) ;
#17533=CARTESIAN_POINT ( 'NONE',  ( -37.00582609754565766, 40.00000000000000000, 48.07482304778140758 ) ) ;
#17541=CARTESIAN_POINT ( 'NONE',  ( 23.12883206328222130, 40.00000000000000000, 11.39561251172168355 ) ) ;
#17548=CYLINDRICAL_SURFACE ( 'NONE', #11033, 2.000000000000000888 ) ;
#17561=CARTESIAN_POINT ( 'NONE',  ( 67.48878131082855703, 31.00000000000000000, 39.09986611101695786 ) ) ;
#17568=CARTESIAN_POINT ( 'NONE',  ( -83.29221842949013421, 40.00000000000000711, -41.19657635676244922 ) ) ;
#17579=CARTESIAN_POINT ( 'NONE',  ( 57.06996419934371545, 31.00000000000000000, 65.05326946699807422 ) ) ;
#17581=CARTESIAN_POINT ( 'NONE',  ( -19.99999999999999645, 31.00000000000000355, 1.283214542831033755 ) ) ;
#17583=CARTESIAN_POINT ( 'NONE',  ( 1.888402776346428613, 40.00000000000000000, 29.39821258742166776 ) ) ;
#17586=EDGE_LOOP ( 'NONE', ( #6757, #23459, #23691, #38903 ) ) ;
#17614=CARTESIAN_POINT ( 'NONE',  ( -14.09736097164098823, 31.00000000000000355, -41.75563764759219509 ) ) ;
#17621=CARTESIAN_POINT ( 'NONE',  ( 64.03668805593822810, 39.99999999999999289, 21.85318084037336561 ) ) ;
#17630=( NAMED_UNIT ( * ) SI_UNIT ( $, .STERADIAN. ) SOLID_ANGLE_UNIT ( ) );
#17634=CARTESIAN_POINT ( 'NONE',  ( 42.89889459577944564, 31.00000000000000355, -32.91970121835214513 ) ) ;
#17640=CARTESIAN_POINT ( 'NONE',  ( -8.325335757348113930, 40.00000000000000000, -31.05587074991522201 ) ) ;
#17641=ORIENTED_EDGE ( 'NONE', *, *, #14083, .F. ) ;
#17644=CARTESIAN_POINT ( 'NONE',  ( -71.72626536482266602, 31.00000000000000711, -9.557116936239163252 ) ) ;
#17645=CARTESIAN_POINT ( 'NONE',  ( 51.69257347811147696, 40.00000000000000000, 59.10123636508003386 ) ) ;
#17660=CARTESIAN_POINT ( 'NONE',  ( 42.89041025189590783, 40.00000000000000000, 86.97820559439793442 ) ) ;
#17672=CARTESIAN_POINT ( 'NONE',  ( -4.434938641671375414, 40.00000000000000000, -34.07637162044569834 ) ) ;
#17673=CARTESIAN_POINT ( 'NONE',  ( -15.99999999999997691, 40.00000000000000000, 5.571627607371296764E-15 ) ) ;
#17683=CARTESIAN_POINT ( 'NONE',  ( -14.19360040536685830, 31.00000000000000355, 24.59234967646941783 ) ) ;
#17689=CARTESIAN_POINT ( 'NONE',  ( 36.74538074116732389, 31.00000000000000355, -63.64477163140654170 ) ) ;
#17691=VERTEX_POINT ( 'NONE', #42152 ) ;
#17692=CARTESIAN_POINT ( 'NONE',  ( 40.10317558968866081, 31.00000000000000355, -23.06553963618950931 ) ) ;
#17693=CARTESIAN_POINT ( 'NONE',  ( 68.07048008643859305, 39.99999999999999289, 33.55317283102968418 ) ) ;
#17706=CARTESIAN_POINT ( 'NONE',  ( 54.43714469963884284, 40.00000000000000000, -7.178810421751046000 ) ) ;
#17737=CARTESIAN_POINT ( 'NONE',  ( -30.97228021248666607, 31.00000000000000355, 23.76985434021725041 ) ) ;
#17746=CARTESIAN_POINT ( 'NONE',  ( 6.892732713553924917, 40.00000000000000000, -52.36990085009771434 ) ) ;
#17748=CARTESIAN_POINT ( 'NONE',  ( 35.58199112951898968, 40.00000000000000000, 46.53705319855855294 ) ) ;
#17753=VECTOR ( 'NONE', #40076, 1000.000000000000000 ) ;
#17754=CARTESIAN_POINT ( 'NONE',  ( -105.9879088449591933, 40.00000000000000711, 4.119280070842334496 ) ) ;
#17757=CARTESIAN_POINT ( 'NONE',  ( -15.93581279029885422, 40.00000000000000000, -13.96891150189262021 ) ) ;
#17773=CARTESIAN_POINT ( 'NONE',  ( 33.43413415811954081, 31.00000000000000355, -67.56680175473152872 ) ) ;
#17780=CIRCLE ( 'NONE', #2347, 2.500000000000000444 ) ;
#17782=CARTESIAN_POINT ( 'NONE',  ( -82.08563009789774867, 40.00000000000000711, 40.34115885382633593 ) ) ;
#17793=CARTESIAN_POINT ( 'NONE',  ( -68.67288961433401084, 31.00000000000000711, -60.22678404055071155 ) ) ;
#17799=CARTESIAN_POINT ( 'NONE',  ( 22.71825314374767402, 40.00000000000000000, -13.09499307598873941 ) ) ;
#17824=FACE_OUTER_BOUND ( 'NONE', #38099, .T. ) ;
#17826=CARTESIAN_POINT ( 'NONE',  ( -5.720710522141557952, 31.00000000000000355, -44.01410879003383059 ) ) ;
#17833=CARTESIAN_POINT ( 'NONE',  ( 57.47007747233163144, 39.99999999999999289, -33.06854485814638878 ) ) ;
#17840=SURFACE_STYLE_FILL_AREA ( #36841 ) ;
#17845=CARTESIAN_POINT ( 'NONE',  ( -18.68892229297488683, 31.00000000000000355, 55.06009237583231197 ) ) ;
#17856=CARTESIAN_POINT ( 'NONE',  ( -29.89583333557403222, 40.00000000000000000, 1.963495399902740690 ) ) ;
#17861=CARTESIAN_POINT ( 'NONE',  ( -64.43604943162229404, 31.00000000000000711, 49.29347324003089881 ) ) ;
#17863=CARTESIAN_POINT ( 'NONE',  ( 66.32976035609178211, 39.99999999999999289, 58.33333674018342663 ) ) ;
#17873=ORIENTED_EDGE ( 'NONE', *, *, #2975, .T. ) ;
#17877=CARTESIAN_POINT ( 'NONE',  ( 86.04713929520032423, 39.99999999999999289, 42.41619695850760507 ) ) ;
#17891=CARTESIAN_POINT ( 'NONE',  ( -29.88476798293163128, 40.00000000000000000, 10.10044382456043266 ) ) ;
#17906=CARTESIAN_POINT ( 'NONE',  ( -19.19493090124598922, 31.00000000000000355, -25.00897302100653263 ) ) ;
#17915=CARTESIAN_POINT ( 'NONE',  ( -77.03666156126601550, 31.00000000000000711, 20.64125776147949409 ) ) ;
#17918=CARTESIAN_POINT ( 'NONE',  ( -24.78443185005114557, 31.00000000000000355, 32.19086620116432584 ) ) ;
#17920=CARTESIAN_POINT ( 'NONE',  ( -11.47416535668642723, 40.00000000000000000, 87.14428777381637303 ) ) ;
#17931=LINE ( 'NONE', #1289, #19813 ) ;
#17935=CARTESIAN_POINT ( 'NONE',  ( -30.90996028308246224, 40.00000000000000000, -53.51249422725337013 ) ) ;
#17967=CARTESIAN_POINT ( 'NONE',  ( 41.10549127292548377, 31.00000000000000355, 20.25863663968860706 ) ) ;
#17971=CIRCLE ( 'NONE', #38802, 2.500000000000002665 ) ;
#17973=ORIENTED_EDGE ( 'NONE', *, *, #6483, .T. ) ;
#17976=CARTESIAN_POINT ( 'NONE',  ( 15.14372185054182651, 40.00000000000000000, 44.57714859939663654 ) ) ;
#17977=CARTESIAN_POINT ( 'NONE',  ( -50.71442127988192539, 40.00000000000000000, -13.67646662467582352 ) ) ;
#17984=CARTESIAN_POINT ( 'NONE',  ( -15.93581279029885422, 31.00000000000000355, -13.96891150189262021 ) ) ;
#17988=CARTESIAN_POINT ( 'NONE',  ( -33.98628324864968420, 40.00000000000000000, 19.63407011443918293 ) ) ;
#18005=CARTESIAN_POINT ( 'NONE',  ( 74.90833963775308746, 31.00000000000000000, 20.17845691862754975 ) ) ;
#18015=CARTESIAN_POINT ( 'NONE',  ( 11.57239447660066567, 40.00000000000000000, 88.72710294830137912 ) ) ;
#18016=CARTESIAN_POINT ( 'NONE',  ( -6.237032369604345483, 31.00000000000000355, -23.31551866006812190 ) ) ;
#18019=PLANE ( 'NONE',  #22170 ) ;
#18020=DIRECTION ( 'NONE',  ( 0.000000000000000000, 0.000000000000000000, -1.000000000000000000 ) ) ;
#18030=CARTESIAN_POINT ( 'NONE',  ( 63.67823170517923614, 31.00000000000000000, 72.58713758494482704 ) ) ;
#18034=CARTESIAN_POINT ( 'NONE',  ( -32.09999204393464822, 40.00000000000000000, -2.147948991655045159 ) ) ;
#18061=CARTESIAN_POINT ( 'NONE',  ( -10.41556553088919834, 31.00000000000000355, 38.62046602036556209 ) ) ;
#18069=CARTESIAN_POINT ( 'NONE',  ( -4.113979049837106494, 40.00000000000000000, -64.40000927351898952 ) ) ;
#18078=CARTESIAN_POINT ( 'NONE',  ( -59.82155519080263417, 31.00000000000000711, -7.874468279917395286 ) ) ;
#18089=CARTESIAN_POINT ( 'NONE',  ( 56.68048384767583769, 31.00000000000000000, -64.44707192207098956 ) ) ;
#18090=CARTESIAN_POINT ( 'NONE',  ( 86.62806645044916820, 39.99999999999999289, 11.52843970785434990 ) ) ;
#18102=CARTESIAN_POINT ( 'NONE',  ( 41.30831894254264824, 40.00000000000000000, -83.80005689411834169 ) ) ;
#18120=CARTESIAN_POINT ( 'NONE',  ( -8.786317949316114095, 40.00000000000000000, -33.00646673686679833 ) ) ;
#18130=CARTESIAN_POINT ( 'NONE',  ( -14.08558183832706234, 31.00000000000000355, -28.55406316770863739 ) ) ;
#18132=DIRECTION ( 'NONE',  ( 0.000000000000000000, 1.000000000000000000, 0.000000000000000000 ) ) ;
#18136=CARTESIAN_POINT ( 'NONE',  ( -79.27599250299880396, 31.00000000000000711, 10.45126230984107707 ) ) ;
#18140=CARTESIAN_POINT ( 'NONE',  ( 56.89991739620084132, 31.00000000000000355, -3.630084216720528278 ) ) ;
#18141=CARTESIAN_POINT ( 'NONE',  ( -29.64342647699677613, 40.00000000000000000, -87.27882330658468391 ) ) ;
#18152=CARTESIAN_POINT ( 'NONE',  ( 38.75409931461306456, 40.00000000000000000, -50.52625141960567134 ) ) ;
#18168=CARTESIAN_POINT ( 'NONE',  ( -101.1468392227577340, 31.00000000000000711, 13.20405500233197671 ) ) ;
#18182=CARTESIAN_POINT ( 'NONE',  ( 52.83624534446448706, 31.00000000000000355, -14.15919354876300318 ) ) ;
#18189=CARTESIAN_POINT ( 'NONE',  ( 55.10416666547021691, 40.00000000000000000, 3.599741573803287853 ) ) ;
#18190=CARTESIAN_POINT ( 'NONE',  ( -40.14822235766499148, 40.00000000000000000, 45.62378674120105160 ) ) ;
#18198=CARTESIAN_POINT ( 'NONE',  ( 1.472621547668719444, 31.00000000000000355, -22.60416666365413718 ) ) ;
#18200=CARTESIAN_POINT ( 'NONE',  ( -20.72449291656876369, 40.00000000000000000, -23.61699481730619610 ) ) ;
#18213=CARTESIAN_POINT ( 'NONE',  ( -55.03444096782886419, 31.00000000000000355, -48.41538206856125015 ) ) ;
#18223=CARTESIAN_POINT ( 'NONE',  ( 39.23423008407738877, 40.00000000000000000, 79.83814995801118641 ) ) ;
#18226=CARTESIAN_POINT ( 'NONE',  ( -21.37212791037561388, 31.00000000000000355, -7.253704819187424491 ) ) ;
#18232=ADVANCED_FACE ( 'NONE', ( #8967 ), #18628, .T. ) ;
#18239=CARTESIAN_POINT ( 'NONE',  ( 48.45023387855729879, 31.00000000000000355, 83.88660019351674180 ) ) ;
#18240=CARTESIAN_POINT ( 'NONE',  ( -16.41266422346949128, 31.00000000000000355, -1.216702565357028698 ) ) ;
#18242=CARTESIAN_POINT ( 'NONE',  ( 12.72035051019986618, 40.00000000000000000, 25.87482915247129966 ) ) ;
#18269=CARTESIAN_POINT ( 'NONE',  ( 45.06603723660748528, 31.00000000000000355, 15.38899812203272788 ) ) ;
#18276=CARTESIAN_POINT ( 'NONE',  ( -47.50570208456527865, 40.00000000000000000, -41.80188021843024870 ) ) ;
#18287=CARTESIAN_POINT ( 'NONE',  ( 64.37268382102905662, 31.00000000000000000, -8.487791176987355968 ) ) ;
#18297=CARTESIAN_POINT ( 'NONE',  ( -40.08783408682389648, 31.00000000000000355, 81.04563091337925584 ) ) ;
#18298=CARTESIAN_POINT ( 'NONE',  ( -82.08563009789774867, 40.00000000000000711, 40.34115885382633593 ) ) ;
#18305=LINE ( 'NONE', #27889, #30461 ) ;
#18310=CARTESIAN_POINT ( 'NONE',  ( 81.71702119589899382, 39.99999999999999289, -47.19735719316410183 ) ) ;
#18325=LINE ( 'NONE', #35488, #40507 ) ;
#18327=CARTESIAN_POINT ( 'NONE',  ( 23.59836588144746017, 40.00000000000000000, -26.81698947917456621 ) ) ;
#18338=CARTESIAN_POINT ( 'NONE',  ( -13.53264355869793967, 31.00000000000000355, -39.83251807627727459 ) ) ;
#18342=CARTESIAN_POINT ( 'NONE',  ( 46.64447153568531945, 31.00000000000000355, 60.78881617101084345 ) ) ;
#18347=CARTESIAN_POINT ( 'NONE',  ( 38.48770111205617894, 31.00000000000000355, 44.02435964457617956 ) ) ;
#18351=CARTESIAN_POINT ( 'NONE',  ( -81.55297449308174862, 40.00000000000000711, -40.20044092665353475 ) ) ;
#18363=CARTESIAN_POINT ( 'NONE',  ( -37.49462465745612860, 40.00000000000000000, -48.86220178749748300 ) ) ;
#18364=LINE ( 'NONE', #35321, #6146 ) ;
#18389=LINE ( 'NONE', #41886, #237 ) ;
#18390=CARTESIAN_POINT ( 'NONE',  ( -15.46676570949300000, 31.00000000000000355, 45.57083133015776610 ) ) ;
#18400=CARTESIAN_POINT ( 'NONE',  ( -15.01009539198478748, 40.00000000000000000, 56.06562763604418365 ) ) ;
#18401=CARTESIAN_POINT ( 'NONE',  ( -7.911223860816524400, 40.00000000000000000, 59.30865348673674475 ) ) ;
#18410=CARTESIAN_POINT ( 'NONE',  ( -23.46968090759046888, 40.00000000000000000, -20.57717900685300449 ) ) ;
#18417=CYLINDRICAL_SURFACE ( 'NONE', #28993, 4.500000000000002665 ) ;
#18423=CARTESIAN_POINT ( 'NONE',  ( 39.23423008409712054, 31.00000000000000355, 79.83814995801117220 ) ) ;
#18434=CARTESIAN_POINT ( 'NONE',  ( 27.02985023942251175, 31.00000000000000355, 3.586895573513789071 ) ) ;
#18443=CARTESIAN_POINT ( 'NONE',  ( 91.55691129138550366, 31.00000000000000000, -24.53049628908797430 ) ) ;
#18449=CARTESIAN_POINT ( 'NONE',  ( 27.02985023942251885, 40.00000000000000000, 3.586895573513070090 ) ) ;
#18474=( GEOMETRIC_REPRESENTATION_CONTEXT ( 3 ) GLOBAL_UNCERTAINTY_ASSIGNED_CONTEXT ( ( #13897 ) ) GLOBAL_UNIT_ASSIGNED_CONTEXT ( ( #159, #11062, #10227 ) ) REPRESENTATION_CONTEXT ( 'NONE', 'WORKASPACE' ) );
#18478=CARTESIAN_POINT ( 'NONE',  ( -34.17541447290002310, 31.00000000000000355, -26.31327426976606176 ) ) ;
#18486=CARTESIAN_POINT ( 'NONE',  ( -60.39136959355892031, 40.00000000000000711, -16.27924862580663046 ) ) ;
#18496=CARTESIAN_POINT ( 'NONE',  ( 9.510694223897102617, 31.00000000000000355, -72.24097909213479340 ) ) ;
#18506=CARTESIAN_POINT ( 'NONE',  ( 87.09251733236551729, 31.00000000000000000, 5.815661930448015937 ) ) ;
#18507=CARTESIAN_POINT ( 'NONE',  ( -5.980347265640406640, 40.00000000000000000, 89.59238221261722401 ) ) ;
#18535=CARTESIAN_POINT ( 'NONE',  ( -105.9879088449591933, 40.00000000000000000, -0.3807199291576673361 ) ) ;
#18539=CARTESIAN_POINT ( 'NONE',  ( 36.95980244579788376, 40.00000000000000000, 4.931273285801174744 ) ) ;
#18554=CARTESIAN_POINT ( 'NONE',  ( -35.29531037056285214, 31.00000000000000355, 17.40921588598563119 ) ) ;
#18561=CARTESIAN_POINT ( 'NONE',  ( -49.69442049507403425, 31.00000000000000355, -64.76435429890716478 ) ) ;
#18563=CARTESIAN_POINT ( 'NONE',  ( -7.015336270751801884, 31.00000000000000355, -53.95087245963820521 ) ) ;
#18564=CARTESIAN_POINT ( 'NONE',  ( -77.37786320076959612, 40.00000000000000711, 44.69160382239309115 ) ) ;
#18581=CARTESIAN_POINT ( 'NONE',  ( 59.08215048199704711, 39.99999999999999289, 29.12166076727282515 ) ) ;
#18616=CARTESIAN_POINT ( 'NONE',  ( 30.63689417572177831, 31.00000000000000355, 34.91779699477408627 ) ) ;
#18624=CARTESIAN_POINT ( 'NONE',  ( 8.201713468707295007, 40.00000000000000000, -62.30543997111072940 ) ) ;
#18628=CYLINDRICAL_SURFACE ( 'NONE', #8873, 4.500000000000002665 ) ;
#18632=CARTESIAN_POINT ( 'NONE',  ( -13.09503298281258132, 31.00000000000000355, -17.05789676611946959 ) ) ;
#18634=CARTESIAN_POINT ( 'NONE',  ( 4.888094100070568437, 40.00000000000000000, 37.04995123692341252 ) ) ;
#18646=AXIS2_PLACEMENT_3D ( 'NONE', #18720, #11484, #11713 ) ;
#18651=CARTESIAN_POINT ( 'NONE',  ( -40.35386350238496789, 31.00000000000000355, 69.65762217234957632 ) ) ;
#18665=CARTESIAN_POINT ( 'NONE',  ( 23.62253089228586234, 31.00000000000000355, -11.62353008834390167 ) ) ;
#18675=CARTESIAN_POINT ( 'NONE',  ( 90.64482129758324902, 31.00000000000000000, 30.77200948131585889 ) ) ;
#18679=CARTESIAN_POINT ( 'NONE',  ( -28.96462450050677973, 40.00000000000000000, -9.827991688575851370 ) ) ;
#18680=CARTESIAN_POINT ( 'NONE',  ( -10.41556553088919834, 40.00000000000000000, 38.62046602037417387 ) ) ;
#18695=CARTESIAN_POINT ( 'NONE',  ( -15.99999999999997691, 39.99999999999999289, -4.499999999999995559 ) ) ;
#18707=CARTESIAN_POINT ( 'NONE',  ( -46.12092335262209986, 31.00000000000000355, 22.64177125690870795 ) ) ;
#18716=VECTOR ( 'NONE', #19925, 1000.000000000000000 ) ;
#18717=CARTESIAN_POINT ( 'NONE',  ( -32.59403919554602425, 40.00000000000000000, -66.35267222978370683 ) ) ;
#18720=CARTESIAN_POINT ( 'NONE',  ( -15.99999999999997691, 17.11489954122026447, 5.571627607371296764E-15 ) ) ;
#18722=DIRECTION ( 'NONE',  ( 0.000000000000000000, 0.000000000000000000, 1.000000000000000000 ) ) ;
#18729=CARTESIAN_POINT ( 'NONE',  ( -34.23962737045593485, 31.00000000000000355, 59.30561363632230609 ) ) ;
#18736=CARTESIAN_POINT ( 'NONE',  ( 28.55926749297819711, 31.00000000000000355, 84.46800049165048563 ) ) ;
#18737=CARTESIAN_POINT ( 'NONE',  ( 53.86549405311984628, 40.00000000000000000, 70.40131829845091715 ) ) ;
#18757=CARTESIAN_POINT ( 'NONE',  ( 26.62151981922249533, 31.00000000000000355, -3.482817046706074393 ) ) ;
#18765=CARTESIAN_POINT ( 'NONE',  ( 41.62382930722196051, 40.00000000000000000, -20.43270582883756248 ) ) ;
#18781=CARTESIAN_POINT ( 'NONE',  ( -35.44024466369167925, 31.00000000000000355, -20.45798383175513635 ) ) ;
#18786=CARTESIAN_POINT ( 'NONE',  ( 50.95389515256417923, 31.00000000000000355, -66.42840393140320998 ) ) ;
#18788=CARTESIAN_POINT ( 'NONE',  ( 35.58199112953183629, 31.00000000000000355, 46.53705319858424616 ) ) ;
#18789=CARTESIAN_POINT ( 'NONE',  ( 24.08498528996878107, 40.00000000000000000, -89.94621034038658536 ) ) ;
#18803=CARTESIAN_POINT ( 'NONE',  ( 49.83821931962687302, 40.00000000000000000, 43.70611527624207326 ) ) ;
#18831=CARTESIAN_POINT ( 'NONE',  ( 28.34477777927418529, 31.00000000000000355, 36.93558740410973229 ) ) ;
#18835=CARTESIAN_POINT ( 'NONE',  ( -19.97695672607123640, 40.00000000000000000, -58.81104016858105155 ) ) ;
#18843=CARTESIAN_POINT ( 'NONE',  ( -39.89583333501392559, 40.00000000000000000, 2.617993869485681468 ) ) ;
#18857=CARTESIAN_POINT ( 'NONE',  ( -64.43604943162229404, 31.00000000000000711, 49.29347324003089881 ) ) ;
#18865=CARTESIAN_POINT ( 'NONE',  ( -15.43003214871278139, 31.00000000000000355, -17.59684744742187945 ) ) ;
#18866=EDGE_CURVE ( 'NONE', #40502, #3181, #27771, .T. ) ;
#18878=CARTESIAN_POINT ( 'NONE',  ( -43.52407497442469264, 31.00000000000000355, 88.29422169633753015 ) ) ;
#18882=CARTESIAN_POINT ( 'NONE',  ( -30.10416666442597844, 40.00000000000000000, -1.963495399902747574 ) ) ;
#18883=CARTESIAN_POINT ( 'NONE',  ( -37.12595630543398073, 40.00000000000000000, 18.22532657727797911 ) ) ;
#18911=CARTESIAN_POINT ( 'NONE',  ( -49.95450512538511134, 31.00000000000000355, 13.28959769214884545 ) ) ;
#18919=CARTESIAN_POINT ( 'NONE',  ( -71.72626536479072001, 40.00000000000000711, -9.557116936239163252 ) ) ;
#18929=CARTESIAN_POINT ( 'NONE',  ( -56.48955861152074220, 31.00000000000000711, -43.32902275382048174 ) ) ;
#18940=CARTESIAN_POINT ( 'NONE',  ( 73.86091552538547944, 31.00000000000000000, 64.94433634442138725 ) ) ;
#18941=CARTESIAN_POINT ( 'NONE',  ( -26.02152878260477564, 40.00000000000000000, 96.68563202207252516 ) ) ;
#18944=AXIS2_PLACEMENT_3D ( 'NONE', #23496, #7294, #36756 ) ;
#18962=CARTESIAN_POINT ( 'NONE',  ( 18.71272080434062701, 31.00000000000000355, 21.38210947162711406 ) ) ;
#18970=CARTESIAN_POINT ( 'NONE',  ( -26.91141215548883991, 40.00000000000000000, 30.57553017915055449 ) ) ;
#18982=CARTESIAN_POINT ( 'NONE',  ( -29.26739590608564967, 31.00000000000000355, 25.68069354617348665 ) ) ;
#18984=FILL_AREA_STYLE_COLOUR ( '', #30206 ) ;
#18988=CARTESIAN_POINT ( 'NONE',  ( 29.96647033545507455, 31.00000000000000355, -88.27250603610892199 ) ) ;
#18991=CARTESIAN_POINT ( 'NONE',  ( 50.14038141241295676, 31.00000000000000355, 29.06424286984032435 ) ) ;
#18993=CARTESIAN_POINT ( 'NONE',  ( -74.47060461443528823, 40.00000000000000711, 65.33029858165178894 ) ) ;
#19006=CARTESIAN_POINT ( 'NONE',  ( 70.67261647610648367, 39.99999999999999289, -24.00465245562410743 ) ) ;
#19029=CARTESIAN_POINT ( 'NONE',  ( 48.45771864870608425, 31.00000000000000355, 27.97524394371832202 ) ) ;
#19035=CARTESIAN_POINT ( 'NONE',  ( -7.547223091130065953, 40.00000000000000000, 57.33767041057931380 ) ) ;
#19044=CARTESIAN_POINT ( 'NONE',  ( -47.99616210117395099, 40.00000000000000000, 12.86278070621785119 ) ) ;
#19058=CARTESIAN_POINT ( 'NONE',  ( 83.01093309086799366, 31.00000000000000000, 28.30804032755801458 ) ) ;
#19071=CARTESIAN_POINT ( 'NONE',  ( -16.73417733071809721, 31.00000000000000355, -12.82953315787133519 ) ) ;
#19080=CARTESIAN_POINT ( 'NONE',  ( 16.14498194198480618, 40.00000000000000000, 21.03343489346954698 ) ) ;
#19083=CARTESIAN_POINT ( 'NONE',  ( -42.09738266246711902, 40.00000000000000000, -2.828681863544772135 ) ) ;
#19104=ORIENTED_EDGE ( 'NONE', *, *, #26522, .F. ) ;
#19105=CARTESIAN_POINT ( 'NONE',  ( -29.64342647699677613, 40.00000000000000000, -87.27882330658468391 ) ) ;
#19112=CARTESIAN_POINT ( 'NONE',  ( -39.97893566998936166, 31.00000000000000355, -35.18630237794885574 ) ) ;
#19118=CARTESIAN_POINT ( 'NONE',  ( 73.52353481979008620, 39.99999999999999289, 25.08131146963209090 ) ) ;
#19130=CARTESIAN_POINT ( 'NONE',  ( -21.91107887650263564, 31.00000000000000355, 64.54935342160338507 ) ) ;
#19140=CARTESIAN_POINT ( 'NONE',  ( 30.72743980831337751, 31.00000000000000355, -90.12673907452091271 ) ) ;
#19141=CARTESIAN_POINT ( 'NONE',  ( 97.09201668843398636, 39.99999999999999289, 6.474068422258194566 ) ) ;
#19152=DIRECTION ( 'NONE',  ( 0.000000000000000000, 0.000000000000000000, -1.000000000000000000 ) ) ;
#19159=CARTESIAN_POINT ( 'NONE',  ( 26.53203760875093309, 31.00000000000000355, 7.134992448514335450 ) ) ;
#19160=EDGE_CURVE ( 'NONE', #11466, #7939, #31989, .T. ) ;
#19163=DIRECTION ( 'NONE',  ( 0.000000000000000000, 0.000000000000000000, 1.000000000000000000 ) ) ;
#19169=CARTESIAN_POINT ( 'NONE',  ( 47.09643503918425012, 40.00000000000000000, 3.164684800459844904 ) ) ;
#19184=CARTESIAN_POINT ( 'NONE',  ( -38.31599561464027914, 31.00000000000000355, 10.26995502114586678 ) ) ;
#19189=CARTESIAN_POINT ( 'NONE',  ( -12.08748825390017068, 31.00000000000000355, -91.69541640458645304 ) ) ;
#19193=CARTESIAN_POINT ( 'NONE',  ( 40.05902963217418744, 31.00000000000000355, -52.04757428483648596 ) ) ;
#19194=CARTESIAN_POINT ( 'NONE',  ( 58.81396797841472335, 40.00000000000000000, 34.08301911901634895 ) ) ;
#19196=CARTESIAN_POINT ( 'NONE',  ( 83.17098260925966713, 39.99999999999999289, 48.02127090943169208 ) ) ;
#19208=CARTESIAN_POINT ( 'NONE',  ( -79.27599250299880396, 40.00000000000000711, 10.45126230984107707 ) ) ;
#19235=CARTESIAN_POINT ( 'NONE',  ( 61.18335543008118549, 31.00000000000000000, -20.78249587198964576 ) ) ;
#19240=CARTESIAN_POINT ( 'NONE',  ( -31.36635120280995537, 31.00000000000000355, -8.451140850656344128 ) ) ;
#19241=CARTESIAN_POINT ( 'NONE',  ( 59.08215048199704711, 39.99999999999999289, 29.12166076727282515 ) ) ;
#19246=CARTESIAN_POINT ( 'NONE',  ( -105.9879088449591933, 17.11489954122026447, -0.3807199291576673361 ) ) ;
#19247=VECTOR ( 'NONE', #4432, 1000.000000000000000 ) ;
#19253=CARTESIAN_POINT ( 'NONE',  ( 6.197074855318628117, 40.00000000000000000, 46.98549035852928313 ) ) ;
#19261=VERTEX_POINT ( 'NONE', #18695 ) ;
#19264=CARTESIAN_POINT ( 'NONE',  ( 42.86165537668586722, 31.00000000000000355, -73.99543480067944756 ) ) ;
#19274=CARTESIAN_POINT ( 'NONE',  ( -96.33078216555149709, 40.00000000000000711, 32.58251675340183340 ) ) ;
#19285=CARTESIAN_POINT ( 'NONE',  ( 24.21999397792122366, 31.00000000000000355, 8.216913396989165008 ) ) ;
#19291=CARTESIAN_POINT ( 'NONE',  ( 34.56606645648713538, 40.00000000000000000, -4.560848911255810378 ) ) ;
#19292=CARTESIAN_POINT ( 'NONE',  ( 28.69597684714337049, 40.00000000000000000, 25.25520295781286251 ) ) ;
#19300=VECTOR ( 'NONE', #8525, 1000.000000000000114 ) ;
#19312=VECTOR ( 'NONE', #6647, 1000.000000000000114 ) ;
#19324=CARTESIAN_POINT ( 'NONE',  ( -26.81486728382429519, 31.00000000000000355, -46.61672233255472975 ) ) ;
#19332=CARTESIAN_POINT ( 'NONE',  ( -31.21560191380782712, 40.00000000000000000, 63.07420938637471863 ) ) ;
#19344=CARTESIAN_POINT ( 'NONE',  ( 64.36038921521112854, 31.00000000000000000, -37.17434371002195803 ) ) ;
#19348=EDGE_LOOP ( 'NONE', ( #33313, #10958, #8721, #13919 ) ) ;
#19356=CARTESIAN_POINT ( 'NONE',  ( -44.52253807734693680, 31.00000000000000355, 90.03212995789276363 ) ) ;
#19357=CARTESIAN_POINT ( 'NONE',  ( 92.49871336443506209, 39.99999999999999289, 31.53380891771211125 ) ) ;
#19359=VERTEX_POINT ( 'NONE', #3721 ) ;
#19364=EDGE_CURVE ( 'NONE', #14757, #35069, #20152, .T. ) ;
#19387=CARTESIAN_POINT ( 'NONE',  ( 36.21668514975058173, 40.00000000000000000, 31.87730689759005287 ) ) ;
#19399=EDGE_CURVE ( 'NONE', #40502, #19359, #16892, .T. ) ;
#19400=CARTESIAN_POINT ( 'NONE',  ( 30.63689417572177831, 31.00000000000000355, 34.91779699477408627 ) ) ;
#19406=CARTESIAN_POINT ( 'NONE',  ( -44.26264085333531995, 31.00000000000000711, 76.66224561662070869 ) ) ;
#19410=CARTESIAN_POINT ( 'NONE',  ( 67.09393615762301977, 31.00000000000000000, 4.495243625008654043 ) ) ;
#19411=CARTESIAN_POINT ( 'NONE',  ( -67.85934734800838442, 40.00000000000000711, 22.92939687791763248 ) ) ;
#19425=CARTESIAN_POINT ( 'NONE',  ( -18.69663849766352826, 40.00000000000000000, -69.77653669617104981 ) ) ;
#19449=EDGE_CURVE ( 'NONE', #6140, #19619, #43026, .T. ) ;
#19453=CARTESIAN_POINT ( 'NONE',  ( 16.30650823456882748, 31.00000000000000355, -60.90571087954511142 ) ) ;
#19458=CARTESIAN_POINT ( 'NONE',  ( 33.88265278290064941, 31.00000000000000355, 16.77599488388065652 ) ) ;
#19459=CARTESIAN_POINT ( 'NONE',  ( 52.51402048354923835, 40.00000000000000000, 40.27907379435107060 ) ) ;
#19469=CARTESIAN_POINT ( 'NONE',  ( 36.61186797162192619, 40.00000000000000000, 28.07927795628900469 ) ) ;
#19481=CARTESIAN_POINT ( 'NONE',  ( 58.37089435908782065, 31.00000000000000000, -75.89027429297952665 ) ) ;
#19485=FACE_OUTER_BOUND ( 'NONE', #16789, .T. ) ;
#19498=CARTESIAN_POINT ( 'NONE',  ( 16.14498194198480618, 31.00000000000000355, 21.03343489346954698 ) ) ;
#19504=CARTESIAN_POINT ( 'NONE',  ( -32.63632984357925437, 40.00000000000000000, -25.02932899672474676 ) ) ;
#19505=CARTESIAN_POINT ( 'NONE',  ( -14.91913624998189825, 40.00000000000000000, -30.37684071747814230 ) ) ;
#19533=CARTESIAN_POINT ( 'NONE',  ( 55.55275676652586725, 31.00000000000000355, 14.97830846782891356 ) ) ;
#19540=CARTESIAN_POINT ( 'NONE',  ( -79.00001692107187523, 40.00000000000000711, 21.04436337234429999 ) ) ;
#19550=DIRECTION ( 'NONE',  ( 0.000000000000000000, 1.000000000000000000, 0.000000000000000000 ) ) ;
#19552=CARTESIAN_POINT ( 'NONE',  ( -62.77658523491555798, 31.00000000000000711, 48.16944601536268777 ) ) ;
#19561=CARTESIAN_POINT ( 'NONE',  ( 63.29164158772582027, 31.00000000000000000, -71.97807289022838972 ) ) ;
#19562=CARTESIAN_POINT ( 'NONE',  ( 84.84057271799511568, 39.99999999999999289, 49.13019966419678752 ) ) ;
#19580=CARTESIAN_POINT ( 'NONE',  ( -99.67789407897798526, 39.99999999999999289, -5.066036069491909544 ) ) ;
#19583=CARTESIAN_POINT ( 'NONE',  ( -21.70016380022026681, 31.00000000000000355, -5.809120511592387182 ) ) ;
#19585=DIRECTION ( 'NONE',  ( 0.000000000000000000, 1.000000000000000000, -1.060184893785364939E-15 ) ) ;
#19590=CARTESIAN_POINT ( 'NONE',  ( -14.09736097164574709, 40.00000000000000000, -41.75563764761122343 ) ) ;
#19594=CARTESIAN_POINT ( 'NONE',  ( -99.99999999999997158, 35.50000000000000711, 2.428179185498535730E-12 ) ) ;
#19603=CIRCLE ( 'NONE', #14021, 4.500000000000000888 ) ;
#19604=CARTESIAN_POINT ( 'NONE',  ( 38.32544124395173668, 31.00000000000000355, -22.13982348525413002 ) ) ;
#19610=CARTESIAN_POINT ( 'NONE',  ( 57.06996419934371545, 31.00000000000000000, 65.05326946699807422 ) ) ;
#19615=CARTESIAN_POINT ( 'NONE',  ( 34.31975892712151222, 31.00000000000000355, 59.64049725130579560 ) ) ;
#19616=CARTESIAN_POINT ( 'NONE',  ( 60.82800096160986669, 39.99999999999999289, 30.10617641797072963 ) ) ;
#19619=VERTEX_POINT ( 'NONE', #11401 ) ;
#19627=ORIENTED_EDGE ( 'NONE', *, *, #13118, .F. ) ;
#19630=CARTESIAN_POINT ( 'NONE',  ( 74.30822294231431613, 39.99999999999999289, -9.796771932235298408 ) ) ;
#19662=CARTESIAN_POINT ( 'NONE',  ( 20.30000058474805869, 31.00000000000000355, -59.80472289869057789 ) ) ;
#19666=CARTESIAN_POINT ( 'NONE',  ( 9.106956811745659408, 31.00000000000000355, -33.78410985267935018 ) ) ;
#19668=CARTESIAN_POINT ( 'NONE',  ( -69.75709431192164800, 40.00000000000000711, -9.183449035091399537 ) ) ;
#19676=CARTESIAN_POINT ( 'NONE',  ( -3.108867721649295035, 40.00000000000000000, 47.60416666525765095 ) ) ;
#19690=CARTESIAN_POINT ( 'NONE',  ( 43.66223835209735427, 31.00000000000000355, 88.82794485014694885 ) ) ;
#19709=CARTESIAN_POINT ( 'NONE',  ( 24.89583333603155069, 31.00000000000000355, -1.636246165087041016 ) ) ;
#19716=CARTESIAN_POINT ( 'NONE',  ( -39.95047694894377344, 40.00000000000000000, -5.256506769647570465 ) ) ;
#19717=CARTESIAN_POINT ( 'NONE',  ( 46.89194940766294906, 40.00000000000000000, 6.259973086888630078 ) ) ;
#19739=ORIENTED_EDGE ( 'NONE', *, *, #19364, .F. ) ;
#19744=CARTESIAN_POINT ( 'NONE',  ( 3.791180027291366716, 31.00000000000000355, 59.39995347152935778 ) ) ;
#19751=CARTESIAN_POINT ( 'NONE',  ( -60.98551593176824070, 40.00000000000000711, 53.34359504439791522 ) ) ;
#19759=( GEOMETRIC_REPRESENTATION_CONTEXT ( 3 ) GLOBAL_UNCERTAINTY_ASSIGNED_CONTEXT ( ( #41772 ) ) GLOBAL_UNIT_ASSIGNED_CONTEXT ( ( #4708, #1636, #17630 ) ) REPRESENTATION_CONTEXT ( 'NONE', 'WORKASPACE' ) );
#19766=CARTESIAN_POINT ( 'NONE',  ( -36.24314215638268877, 31.00000000000000355, -73.49571118816069770 ) ) ;
#19776=CARTESIAN_POINT ( 'NONE',  ( -24.28006566512905451, 31.00000000000000355, -91.10131089348453770 ) ) ;
#19794=CARTESIAN_POINT ( 'NONE',  ( -29.88476798293162418, 31.00000000000000355, 10.10044382456042911 ) ) ;
#19802=CARTESIAN_POINT ( 'NONE',  ( -22.33566874673302038, 40.00000000000000000, 45.10700316350094141 ) ) ;
#19813=VECTOR ( 'NONE', #30972, 1000.000000000000000 ) ;
#19816=CARTESIAN_POINT ( 'NONE',  ( 28.34477777927418529, 31.00000000000000355, 36.93558740410973229 ) ) ;
#19824=CARTESIAN_POINT ( 'NONE',  ( 38.45889818826288575, 31.00000000000000355, 77.98987599019784511 ) ) ;
#19829=CARTESIAN_POINT ( 'NONE',  ( -30.31917247938466176, 31.00000000000000355, 52.30862930534038924 ) ) ;
#19830=CARTESIAN_POINT ( 'NONE',  ( -18.22940504111446458, 40.00000000000000000, 67.64968002090884625 ) ) ;
#19831=CARTESIAN_POINT ( 'NONE',  ( 42.89041025189590783, 40.00000000000000000, 86.97820559439793442 ) ) ;
#19832=ORIENTED_EDGE ( 'NONE', *, *, #35248, .F. ) ;
#19846=CARTESIAN_POINT ( 'NONE',  ( -68.16583574478268304, 40.00000000000000711, -18.25112749842637427 ) ) ;
#19854=CARTESIAN_POINT ( 'NONE',  ( 47.87658044097961607, 31.00000000000000000, -82.67148682534870829 ) ) ;
#19870=CARTESIAN_POINT ( 'NONE',  ( -7.088330391075835735, 31.00000000000000355, -20.85399598300688595 ) ) ;
#19879=CARTESIAN_POINT ( 'NONE',  ( 14.80739997004469366, 31.00000000000000355, 55.25628696611591550 ) ) ;
#19882=CARTESIAN_POINT ( 'NONE',  ( -10.89792128226954127, 31.00000000000000355, -32.25956908330170592 ) ) ;
#19884=CARTESIAN_POINT ( 'NONE',  ( -69.89583333424914713, 40.00000000000000711, 4.581489278091138040 ) ) ;
#19892=CARTESIAN_POINT ( 'NONE',  ( 42.20483333784007840, 40.00000000000000000, -14.33818270462009359 ) ) ;
#19910=CARTESIAN_POINT ( 'NONE',  ( 94.26586287999620595, 31.00000000000000000, 25.37251369639959364 ) ) ;
#19923=AXIS2_PLACEMENT_3D ( 'NONE', #27749, #40570, #7642 ) ;
#19925=DIRECTION ( 'NONE',  ( 0.000000000000000000, 1.000000000000000000, 0.000000000000000000 ) ) ;
#19930=CARTESIAN_POINT ( 'NONE',  ( -23.02120395722396395, 31.00000000000000355, 17.66995642160909696 ) ) ;
#19938=CARTESIAN_POINT ( 'NONE',  ( -5.542584477697039880, 40.00000000000000000, -42.01772079774592328 ) ) ;
#19939=CARTESIAN_POINT ( 'NONE',  ( 44.12914893502614433, 40.00000000000000000, -14.89880614700436645 ) ) ;
#19961=ORIENTED_EDGE ( 'NONE', *, *, #22006, .F. ) ;
#19965=CARTESIAN_POINT ( 'NONE',  ( -19.99999999999999645, 40.00000000000000000, 1.283214542831032867 ) ) ;
#19971=CARTESIAN_POINT ( 'NONE',  ( -40.14822235767833547, 31.00000000000000355, 45.62378674120104449 ) ) ;
#19973=LINE ( 'NONE', #13622, #40447 ) ;
#19979=CARTESIAN_POINT ( 'NONE',  ( 5.085823974618865151, 40.00000000000000000, 79.40009828669005287 ) ) ;
#19988=CARTESIAN_POINT ( 'NONE',  ( -34.66105084696506822, 31.00000000000000355, 70.31756248751102589 ) ) ;
#19997=FACE_OUTER_BOUND ( 'NONE', #17586, .T. ) ;
#20009=ORIENTED_EDGE ( 'NONE', *, *, #1846, .F. ) ;
#20024=CARTESIAN_POINT ( 'NONE',  ( 17.12248163736668261, 31.00000000000000355, 34.87662400048955647 ) ) ;
#20033=CARTESIAN_POINT ( 'NONE',  ( 54.79583221321230724, 40.00000000000000000, -14.58025558542526490 ) ) ;
#20046=CARTESIAN_POINT ( 'NONE',  ( -49.46937513889707105, 31.00000000000000355, 6.524320044134898744 ) ) ;
#20053=CARTESIAN_POINT ( 'NONE',  ( -1.472621547668719444, 40.00000000000000000, -22.39583333634585571 ) ) ;
#20057=CARTESIAN_POINT ( 'NONE',  ( -16.51797447735581059, 31.00000000000000355, -62.05742538355529803 ) ) ;
#20058=CARTESIAN_POINT ( 'NONE',  ( -60.39136959355892031, 40.00000000000000711, -16.27924862580663046 ) ) ;
#20077=CARTESIAN_POINT ( 'NONE',  ( 22.58587702529213104, 40.00000000000000000, 84.29678642628191199 ) ) ;
#20089=CARTESIAN_POINT ( 'NONE',  ( 25.13348990051749965, 40.00000000000000000, -8.510361017570636122 ) ) ;
#20098=VECTOR ( 'NONE', #21859, 1000.000000000000000 ) ;
#20103=ORIENTED_EDGE ( 'NONE', *, *, #23649, .F. ) ;
#20109=CARTESIAN_POINT ( 'NONE',  ( 70.67261647610648367, 31.00000000000000000, -24.00465245562410743 ) ) ;
#20112=CARTESIAN_POINT ( 'NONE',  ( -31.59164309906361368, 31.00000000000000355, 4.115917706319392799 ) ) ;
#20113=CARTESIAN_POINT ( 'NONE',  ( -21.91107887650263564, 40.00000000000000000, 64.54935342160338507 ) ) ;
#20123=CARTESIAN_POINT ( 'NONE',  ( 25.16436199730139123, 40.00000000000000000, 51.02488717759543135 ) ) ;
#20138=CARTESIAN_POINT ( 'NONE',  ( 24.72345498302141920, 31.00000000000000355, -91.84610802666480822 ) ) ;
#20152=CIRCLE ( 'NONE', #1291, 2.500000000000002665 ) ;
#20153=ORIENTED_EDGE ( 'NONE', *, *, #36812, .F. ) ;
#20154=CARTESIAN_POINT ( 'NONE',  ( -40.10416666498607441, 31.00000000000000355, -2.617993869485698344 ) ) ;
#20162=CARTESIAN_POINT ( 'NONE',  ( 33.70925502316616473, 40.00000000000000000, 11.43906998022225707 ) ) ;
#20163=CARTESIAN_POINT ( 'NONE',  ( 45.11287655886649617, 40.00000000000000000, -12.00022417491798521 ) ) ;
#20189=CARTESIAN_POINT ( 'NONE',  ( 65.23019871247133494, 31.00000000000000000, 17.57949444736449252 ) ) ;
#20196=CARTESIAN_POINT ( 'NONE',  ( 56.68048384767583769, 39.99999999999999289, -64.44707192207098956 ) ) ;
#20205=EDGE_CURVE ( 'NONE', #9994, #31505, #18364, .T. ) ;
#20206=CARTESIAN_POINT ( 'NONE',  ( 23.52215716829092074, 31.00000000000000355, -69.29398394448777765 ) ) ;
#20235=CARTESIAN_POINT ( 'NONE',  ( 27.04960320298028620, 31.00000000000000355, -23.64836272119223892 ) ) ;
#20239=CARTESIAN_POINT ( 'NONE',  ( -104.2750351721725650, 31.00000000000000000, -4.541977405098627685 ) ) ;
#20244=CARTESIAN_POINT ( 'NONE',  ( -49.80813925210025417, 40.00000000000000000, -17.00652635548005520 ) ) ;
#20246=DIRECTION ( 'NONE',  ( 0.000000000000000000, 1.000000000000000000, 0.000000000000000000 ) ) ;
#20252=CARTESIAN_POINT ( 'NONE',  ( -33.94102792873697183, 31.00000000000000355, -38.68473105385043453 ) ) ;
#20261=CARTESIAN_POINT ( 'NONE',  ( 95.10416666600561086, 31.00000000000000000, 6.217735451873073416 ) ) ;
#20267=CARTESIAN_POINT ( 'NONE',  ( 24.27443280711675300, 31.00000000000000355, -71.15176282235542260 ) ) ;
#20268=CARTESIAN_POINT ( 'NONE',  ( 4.991138515316659863, 40.00000000000000000, -74.59332054773635434 ) ) ;
#20281=CARTESIAN_POINT ( 'NONE',  ( -28.35539204363714205, 40.00000000000000000, 83.52787551312086123 ) ) ;
#20294=CARTESIAN_POINT ( 'NONE',  ( 24.91045342551595354, 40.00000000000000000, 12.31387362277309272 ) ) ;
#20306=LINE ( 'NONE', #40318, #23180 ) ;
#20314=CARTESIAN_POINT ( 'NONE',  ( 63.32575250126041055, 31.00000000000000000, 16.95471465585521997 ) ) ;
#20316=CARTESIAN_POINT ( 'NONE',  ( 41.46880187713386334, 31.00000000000000355, 24.04226233541373858 ) ) ;
#20317=CARTESIAN_POINT ( 'NONE',  ( 21.49215960483416410, 40.00000000000000000, -80.26604385357094884 ) ) ;
#20330=CARTESIAN_POINT ( 'NONE',  ( 52.68777711438346500, 40.00000000000000000, 17.88338314711659294 ) ) ;
#20342=CARTESIAN_POINT ( 'NONE',  ( -86.84058463553202500, 31.00000000000000711, 29.36381822872188607 ) ) ;
#20353=DIRECTION ( 'NONE',  ( -0.9470131699890049770, -3.405258028344997528E-16, -0.3211947320043963550 ) ) ;
#20360=CARTESIAN_POINT ( 'NONE',  ( 34.98270738856093232, 31.00000000000000355, 4.602016392115340970 ) ) ;
#20366=CARTESIAN_POINT ( 'NONE',  ( -13.51098712749246467, 40.00000000000000000, -50.41620372279128048 ) ) ;
#20367=CARTESIAN_POINT ( 'NONE',  ( 45.87644943786595064, 40.00000000000000000, 12.37342411884007731 ) ) ;
#20375=CARTESIAN_POINT ( 'NONE',  ( -16.73417733071809721, 40.00000000000000000, -12.82953315787133519 ) ) ;
#20395=CARTESIAN_POINT ( 'NONE',  ( -61.89998375878432313, 31.00000000000000711, 3.952486745199417673 ) ) ;
#20403=CARTESIAN_POINT ( 'NONE',  ( -81.90010630563853056, 40.00000000000000711, 5.248159452637418454 ) ) ;
#20415=CARTESIAN_POINT ( 'NONE',  ( -80.23695839127151430, 31.00000000000000711, 39.56677620416681407 ) ) ;
#20422=VERTEX_POINT ( 'NONE', #11093 ) ;
#20424=EDGE_CURVE ( 'NONE', #41658, #35069, #1013, .T. ) ;
#20432=PLANE ( 'NONE',  #35346 ) ;
#20443=CARTESIAN_POINT ( 'NONE',  ( 33.88265278290064941, 31.00000000000000355, 16.77599488388065652 ) ) ;
#20454=CARTESIAN_POINT ( 'NONE',  ( -50.71442127988192539, 40.00000000000000000, -13.67646662467582352 ) ) ;
#20465=CARTESIAN_POINT ( 'NONE',  ( 8.201713468707295007, 31.00000000000000355, -62.30543997111072940 ) ) ;
#20472=CARTESIAN_POINT ( 'NONE',  ( 19.04566582976364941, 40.00000000000000000, -14.62000746238684989 ) ) ;
#20477=CARTESIAN_POINT ( 'NONE',  ( 39.32569335900156204, 31.00000000000000355, 68.32161714268157482 ) ) ;
#20478=CARTESIAN_POINT ( 'NONE',  ( 58.79931003850258975, 40.00000000000000000, 51.72161244498203558 ) ) ;
#20493=CARTESIAN_POINT ( 'NONE',  ( -22.78857244739539212, 40.00000000000000000, 85.10612709700112077 ) ) ;
#20508=CARTESIAN_POINT ( 'NONE',  ( 26.10672890669277990, 40.00000000000000000, 8.893381768402427667 ) ) ;
#20518=CARTESIAN_POINT ( 'NONE',  ( -5.732510072307491988, 31.00000000000000355, -21.37570426403446078 ) ) ;
#20525=CARTESIAN_POINT ( 'NONE',  ( -35.92146702467432817, 31.00000000000000355, -62.19081021767443218 ) ) ;
#20528=CARTESIAN_POINT ( 'NONE',  ( 11.72132095739929625, 31.00000000000000355, -43.45763713126748229 ) ) ;
#20530=CARTESIAN_POINT ( 'NONE',  ( 5.399612364985509672, 40.00000000000000000, -82.60416666586320389 ) ) ;
#20536=PRODUCT_DEFINITION_FORMATION_WITH_SPECIFIED_SOURCE ( 'ANY', '', #30486, .NOT_KNOWN. ) ;
#20537=VECTOR ( 'NONE', #40805, 1000.000000000000000 ) ;
#20539=CARTESIAN_POINT ( 'NONE',  ( -49.88601606984090608, 40.00000000000000000, -6.565487524765669214 ) ) ;
#20558=ORIENTED_EDGE ( 'NONE', *, *, #19449, .T. ) ;
#20572=CARTESIAN_POINT ( 'NONE',  ( -32.63632984357925437, 31.00000000000000355, -25.02932899672474676 ) ) ;
#20579=CARTESIAN_POINT ( 'NONE',  ( 51.69409438402072965, 40.00000000000000000, -17.56033928829605273 ) ) ;
#20581=CARTESIAN_POINT ( 'NONE',  ( 3.148395399070833545, 40.00000000000000000, 49.39975974384547897 ) ) ;
#20592=CARTESIAN_POINT ( 'NONE',  ( -14.11622541012940601, 40.00000000000000000, -16.08312669853564358 ) ) ;
#20608=CARTESIAN_POINT ( 'NONE',  ( 57.47007747236072817, 31.00000000000000000, -33.06854485811727784 ) ) ;
#20619=CARTESIAN_POINT ( 'NONE',  ( -56.91377077966711084, 40.00000000000000000, -74.37798324515208037 ) ) ;
#20633=CARTESIAN_POINT ( 'NONE',  ( 84.24376206367318787, 31.00000000000000000, -11.10575268747775901 ) ) ;
#20667=CARTESIAN_POINT ( 'NONE',  ( -23.27229071023271700, 31.00000000000000355, 20.35677778009614869 ) ) ;
#20674=CARTESIAN_POINT ( 'NONE',  ( 3.148395399070833545, 40.00000000000000000, 49.39975974384547897 ) ) ;
#20687=CARTESIAN_POINT ( 'NONE',  ( 37.24516168167158270, 31.00000000000000355, 42.45166511289891531 ) ) ;
#20694=CARTESIAN_POINT ( 'NONE',  ( 12.74197863150380883, 31.00000000000000355, 96.66318596537892915 ) ) ;
#20696=ORIENTED_EDGE ( 'NONE', *, *, #5265, .T. ) ;
#20700=CARTESIAN_POINT ( 'NONE',  ( -65.32047834223114080, 31.00000000000000711, -32.32491738443057017 ) ) ;
#20701=CARTESIAN_POINT ( 'NONE',  ( -23.73339997550686675, 40.00000000000000000, -70.23208777907456124 ) ) ;
#20716=CARTESIAN_POINT ( 'NONE',  ( -11.47416535668642723, 40.00000000000000000, 87.14428777381637303 ) ) ;
#20742=CARTESIAN_POINT ( 'NONE',  ( -8.325335757348113930, 31.00000000000000355, -31.05587074991522201 ) ) ;
#20751=CARTESIAN_POINT ( 'NONE',  ( -63.57631528421845957, 31.00000000000000711, -31.33741679916209222 ) ) ;
#20758=CARTESIAN_POINT ( 'NONE',  ( -32.60815990948594134, 31.00000000000000355, 24.92795611697640368 ) ) ;
#20762=CARTESIAN_POINT ( 'NONE',  ( 72.19657831791809599, 39.99999999999999289, -19.34484491892447622 ) ) ;
#20772=CARTESIAN_POINT ( 'NONE',  ( -59.40491426035100631, 40.00000000000000711, 7.833300799371349932 ) ) ;
#20803=CARTESIAN_POINT ( 'NONE',  ( 5.583751958424166162, 31.00000000000000355, -42.43436172917101601 ) ) ;
#20813=CARTESIAN_POINT ( 'NONE',  ( -24.21661388771557100, 40.00000000000000000, 41.94898165618241137 ) ) ;
#20815=CARTESIAN_POINT ( 'NONE',  ( 3.665567271000699012, 40.00000000000000000, -54.59530427606813419 ) ) ;
#20827=CARTESIAN_POINT ( 'NONE',  ( -18.63466726053507472, 40.00000000000000000, -9.179856479542758407 ) ) ;
#20833=FACE_OUTER_BOUND ( 'NONE', #31308, .T. ) ;
#20836=DIRECTION ( 'NONE',  ( 0.000000000000000000, 1.000000000000000000, 0.000000000000000000 ) ) ;
#20842=CARTESIAN_POINT ( 'NONE',  ( -71.72626536482266602, 31.00000000000000711, -9.557116936239163252 ) ) ;
#20846=VECTOR ( 'NONE', #15306, 1000.000000000000114 ) ;
#20854=CARTESIAN_POINT ( 'NONE',  ( -91.90012763196534706, 40.00000000000000711, 5.898218105444796855 ) ) ;
#20863=CARTESIAN_POINT ( 'NONE',  ( 85.10416666585589951, 31.00000000000000000, 5.563236982362346872 ) ) ;
#20867=CARTESIAN_POINT ( 'NONE',  ( 24.91045342551595354, 40.00000000000000000, 12.31387362277309272 ) ) ;
#20894=CARTESIAN_POINT ( 'NONE',  ( -17.88900094061790469, 31.00000000000000355, 36.12696699725170646 ) ) ;
#20899=CARTESIAN_POINT ( 'NONE',  ( 4.329677741076332964, 40.00000000000000000, -64.59417075179260337 ) ) ;
#20912=CARTESIAN_POINT ( 'NONE',  ( -44.33513214241411760, 31.00000000000000355, 38.89722855811361768 ) ) ;
#20918=CARTESIAN_POINT ( 'NONE',  ( -3.620280825866593055, 40.00000000000000000, 27.53105304817175636 ) ) ;
#20922=CARTESIAN_POINT ( 'NONE',  ( 4.991138515316659863, 31.00000000000000355, -74.59332054773635434 ) ) ;
#20923=CARTESIAN_POINT ( 'NONE',  ( -19.10382689932985656, 40.00000000000000000, -71.73905014343321795 ) ) ;
#20938=CARTESIAN_POINT ( 'NONE',  ( 43.43872713698582544, 40.00000000000000000, 75.20828420317944563 ) ) ;
#20939=CARTESIAN_POINT ( 'NONE',  ( -31.37281731866679024, 31.00000000000001776, 27.62913683693880174 ) ) ;
#20949=CARTESIAN_POINT ( 'NONE',  ( 28.69597684714337049, 40.00000000000000000, 25.25520295781286251 ) ) ;
#20961=AXIS2_PLACEMENT_3D ( 'NONE', #12491, #29072, #35160 ) ;
#20962=CARTESIAN_POINT ( 'NONE',  ( 24.60508655230852781, 31.00000000000000355, 6.583411914924224284 ) ) ;
#20970=CARTESIAN_POINT ( 'NONE',  ( -34.23962737045593485, 31.00000000000000355, 59.30561363632230609 ) ) ;
#20972=CARTESIAN_POINT ( 'NONE',  ( -19.32876798325804302, 31.00000000000000355, -39.37500834189552279 ) ) ;
#20973=CARTESIAN_POINT ( 'NONE',  ( 38.42722039544141666, 40.00000000000000000, 66.52996821281629991 ) ) ;
#20986=CARTESIAN_POINT ( 'NONE',  ( -13.51098712749246467, 40.00000000000000000, -50.41620372279128048 ) ) ;
#20991=VECTOR ( 'NONE', #26537, 1000.000000000000000 ) ;
#21004=CARTESIAN_POINT ( 'NONE',  ( -32.34013556242301490, 31.00000000000000355, 94.87070470182929682 ) ) ;
#21020=CARTESIAN_POINT ( 'NONE',  ( 24.02862666965263116, 31.00000000000000355, 27.38392887651082575 ) ) ;
#21030=CARTESIAN_POINT ( 'NONE',  ( 26.72236725836960147, 40.00000000000000000, -46.28813965123160301 ) ) ;
#21031=CARTESIAN_POINT ( 'NONE',  ( -17.30549157494238344, 40.00000000000000000, -51.24895740946764988 ) ) ;
#21035=EDGE_CURVE ( 'NONE', #33113, #40305, #39516, .T. ) ;
#21040=CARTESIAN_POINT ( 'NONE',  ( 13.36968668718156295, 40.00000000000000000, 23.13838826010315941 ) ) ;
#21056=CARTESIAN_POINT ( 'NONE',  ( -72.09351246574976813, 31.00000000000000711, -4.825959690424619808 ) ) ;
#21057=ORIENTED_EDGE ( 'NONE', *, *, #517, .F. ) ;
#21067=CARTESIAN_POINT ( 'NONE',  ( -72.38966680857410552, 40.00000000000000711, 55.38960906678870799 ) ) ;
#21073=ORIENTED_EDGE ( 'NONE', *, *, #2272, .T. ) ;
#21077=CARTESIAN_POINT ( 'NONE',  ( -87.52616871875942195, 31.00000000000000711, -23.43677886868077209 ) ) ;
#21078=DIRECTION ( 'NONE',  ( -0.3211947320043981868, -5.016842274700473727E-16, -0.9470131699890044219 ) ) ;
#21080=CARTESIAN_POINT ( 'NONE',  ( -21.37212791037562098, 40.00000000000000000, -7.253704819186252983 ) ) ;
#21095=CARTESIAN_POINT ( 'NONE',  ( -16.41266422346948772, 17.11489954122026447, -1.216702565357022037 ) ) ;
#21106=CARTESIAN_POINT ( 'NONE',  ( 21.53706125532763593, 31.00000000000000355, 43.87245753946415761 ) ) ;
#21115=CARTESIAN_POINT ( 'NONE',  ( -56.33579487689732446, 40.00000000000000000, -27.88694065509425357 ) ) ;
#21127=CARTESIAN_POINT ( 'NONE',  ( -30.90996028308246224, 31.00000000000000355, -53.51249422725337013 ) ) ;
#21132=CARTESIAN_POINT ( 'NONE',  ( -26.30698076681265363, 40.00000000000000000, 12.97770382244945253 ) ) ;
#21136=CARTESIAN_POINT ( 'NONE',  ( -53.37462671637112521, 31.00000000000000711, 60.68184199296217685 ) ) ;
#21137=CARTESIAN_POINT ( 'NONE',  ( -86.84058463553202500, 40.00000000000000711, 29.36381822872188607 ) ) ;
#21151=CARTESIAN_POINT ( 'NONE',  ( -43.52407497442469264, 40.00000000000000000, 88.29422169633753015 ) ) ;
#21164=CARTESIAN_POINT ( 'NONE',  ( 27.04960320298795651, 40.00000000000000000, -23.64836272119224247 ) ) ;
#21167=CARTESIAN_POINT ( 'NONE',  ( -101.6738636939643357, 17.11489954122025736, -5.192942712545352890 ) ) ;
#21176=CARTESIAN_POINT ( 'NONE',  ( -23.02120395722396395, 31.00000000000000355, 17.66995642160909696 ) ) ;
#21182=CARTESIAN_POINT ( 'NONE',  ( 68.07048008643859305, 31.00000000000000000, 33.55317283102968418 ) ) ;
#21185=CARTESIAN_POINT ( 'NONE',  ( 27.84166646522859878, 31.00000000000000355, -36.16032403484085478 ) ) ;
#21186=CARTESIAN_POINT ( 'NONE',  ( 19.99305134020393382, 40.00000000000000000, 74.61661993947731730 ) ) ;
#21199=CARTESIAN_POINT ( 'NONE',  ( 43.85342918759069164, 40.00000000000000000, 49.98553323097543455 ) ) ;
#21231=CARTESIAN_POINT ( 'NONE',  ( -33.94102792873697183, 31.00000000000000355, -38.68473105385043453 ) ) ;
#21238=CARTESIAN_POINT ( 'NONE',  ( 30.63689417572177831, 40.00000000000000000, 34.91779699477408627 ) ) ;
#21240=CARTESIAN_POINT ( 'NONE',  ( 38.48770111205618605, 40.00000000000000000, 44.02435964457617956 ) ) ;
#21252=CARTESIAN_POINT ( 'NONE',  ( -29.89583333557403222, 40.00000000000000000, 1.963495399902740690 ) ) ;
#21263=CARTESIAN_POINT ( 'NONE',  ( -104.2750351721725650, 17.11489954122025736, -4.541977405098627685 ) ) ;
#21269=CARTESIAN_POINT ( 'NONE',  ( 37.84579180137232157, 31.00000000000000355, -65.31998993212283722 ) ) ;
#21278=CARTESIAN_POINT ( 'NONE',  ( 87.78546986784174067, 39.99999999999999289, 43.41392487578124815 ) ) ;
#21290=CARTESIAN_POINT ( 'NONE',  ( 21.49215960483416410, 31.00000000000000355, -80.26604385357094884 ) ) ;
#21295=CARTESIAN_POINT ( 'NONE',  ( -31.59164309906362078, 40.00000000000000000, 4.115917706318550806 ) ) ;
#21324=CARTESIAN_POINT ( 'NONE',  ( 45.87644943786595064, 31.00000000000000355, 12.37342411884007376 ) ) ;
#21331=DIRECTION ( 'NONE',  ( 0.000000000000000000, 1.000000000000000000, 0.000000000000000000 ) ) ;
#21332=CARTESIAN_POINT ( 'NONE',  ( 28.99662776679782539, 40.00000000000000000, -58.58186007941694129 ) ) ;
#21342=CARTESIAN_POINT ( 'NONE',  ( -25.79802671946675474, 31.00000000000000355, 52.34090327860478453 ) ) ;
#21348=CARTESIAN_POINT ( 'NONE',  ( -9.022452542771789652, 40.00000000000000000, 26.59230923919664491 ) ) ;
#21354=CARTESIAN_POINT ( 'NONE',  ( -70.49178429274641644, 31.00000000000000711, 40.57739572807859929 ) ) ;
#21355=CARTESIAN_POINT ( 'NONE',  ( 37.87019299813560025, 40.00000000000000000, -76.55254356380190472 ) ) ;
#21362=ORIENTED_EDGE ( 'NONE', *, *, #19449, .F. ) ;
#21372=CARTESIAN_POINT ( 'NONE',  ( -96.39699453480135105, 40.00000000000000711, 25.82690913164849889 ) ) ;
#21378=VECTOR ( 'NONE', #26709, 1000.000000000000114 ) ;
#21388=CARTESIAN_POINT ( 'NONE',  ( -16.82630558382439290, 40.00000000000000000, -29.24196894321155682 ) ) ;
#21403=CARTESIAN_POINT ( 'NONE',  ( 11.68784703496123711, 31.00000000000000355, -20.25319168173327355 ) ) ;
#21408=CARTESIAN_POINT ( 'NONE',  ( -10.16518460146908787, 31.00000000000000355, 77.20874865269769316 ) ) ;
#21410=CARTESIAN_POINT ( 'NONE',  ( -3.469229457552013507, 31.00000000000000355, -54.39987425099493379 ) ) ;
#21413=CARTESIAN_POINT ( 'NONE',  ( -89.21153162435624040, 40.00000000000000711, 11.76024306507019901 ) ) ;
#21428=CARTESIAN_POINT ( 'NONE',  ( 29.59587406094124873, 40.00000000000000000, 60.01321678176139329 ) ) ;
#21460=CARTESIAN_POINT ( 'NONE',  ( -42.66459923921424036, 31.00000000000000355, 24.64557685607233140 ) ) ;
#21467=CARTESIAN_POINT ( 'NONE',  ( 61.18335543008118549, 39.99999999999999289, -20.78249587198964576 ) ) ;
#21469=CARTESIAN_POINT ( 'NONE',  ( 15.22596115864829969, 40.00000000000000000, 57.21640888977480444 ) ) ;
#21479=CARTESIAN_POINT ( 'NONE',  ( -16.93500259178182432, 40.00000000000000000, 34.36424406943201149 ) ) ;
#21495=CARTESIAN_POINT ( 'NONE',  ( 8.965261019430212031, 31.00000000000000355, 68.85524230650666766 ) ) ;
#21502=CARTESIAN_POINT ( 'NONE',  ( 5.735608225908777946, 40.00000000000000000, 89.40012361736363289 ) ) ;
#21504=CARTESIAN_POINT ( 'NONE',  ( 18.71272080434062701, 31.00000000000000355, 21.38210947162711406 ) ) ;
#21519=CARTESIAN_POINT ( 'NONE',  ( 94.17930118497612568, 31.00000000000000000, -12.41473344271720691 ) ) ;
#21523=CARTESIAN_POINT ( 'NONE',  ( -27.06829236441420861, 40.00000000000000000, 15.58100167311933149 ) ) ;
#21550=CARTESIAN_POINT ( 'NONE',  ( 5.076274692534474831, 31.00000000000000355, 39.04542013319161953 ) ) ;
#21557=CARTESIAN_POINT ( 'NONE',  ( 18.91139405008128804, 40.00000000000000000, 55.99505798892768382 ) ) ;
#21567=ORIENTED_EDGE ( 'NONE', *, *, #34192, .T. ) ;
#21570=CARTESIAN_POINT ( 'NONE',  ( -4.745113895469965648, 31.00000000000000355, -72.39583333427917466 ) ) ;
#21580=CARTESIAN_POINT ( 'NONE',  ( 77.59064570035201314, 31.00000000000000000, -38.12735739514867817 ) ) ;
#21581=CARTESIAN_POINT ( 'NONE',  ( -54.99468034528496929, 40.00000000000000000, -62.86974495748533087 ) ) ;
#21594=CARTESIAN_POINT ( 'NONE',  ( 6.381360069253262601, 40.00000000000000000, 97.39583333395333398 ) ) ;
#21606=CARTESIAN_POINT ( 'NONE',  ( 4.597210615070504325, 40.00000000000000000, -34.47704375835832025 ) ) ;
#21619=CARTESIAN_POINT ( 'NONE',  ( 1.799870782497353439, 31.00000000000000355, 27.39583333577991908 ) ) ;
#21624=CARTESIAN_POINT ( 'NONE',  ( 50.46169669344906339, 31.00000000000000355, 57.51940134901310131 ) ) ;
#21628=CARTESIAN_POINT ( 'NONE',  ( 36.84045577241590763, 31.00000000000000355, -41.86038302678687018 ) ) ;
#21629=CARTESIAN_POINT ( 'NONE',  ( 82.68608547523962216, 39.99999999999999289, 22.14036602612658200 ) ) ;
#21641=CARTESIAN_POINT ( 'NONE',  ( 8.201713468707295007, 40.00000000000000000, -62.30543997111072940 ) ) ;
#21645=DIRECTION ( 'NONE',  ( 0.9247238835424298475, 0.000000000000000000, 0.3806385939525924744 ) ) ;
#21668=CARTESIAN_POINT ( 'NONE',  ( -21.03271207055027858, 31.00000000000000711, 3.044856699593506910 ) ) ;
#21669=CARTESIAN_POINT ( 'NONE',  ( -31.39472673864601049, 31.00000000000000355, -40.91112553188754930 ) ) ;
#21675=CARTESIAN_POINT ( 'NONE',  ( 48.45771864870608425, 40.00000000000000000, 27.97524394371832202 ) ) ;
#21676=CARTESIAN_POINT ( 'NONE',  ( 17.81483206086863191, 40.00000000000000000, -52.17936214187551514 ) ) ;
#21684=CARTESIAN_POINT ( 'NONE',  ( -1.472621547668719444, 31.00000000000000355, -22.39583333634585571 ) ) ;
#21686=CARTESIAN_POINT ( 'NONE',  ( -30.97228021248666607, 40.00000000000000000, 23.76985434021725041 ) ) ;
#21698=CARTESIAN_POINT ( 'NONE',  ( 53.86549405311983918, 31.00000000000000355, 70.40131829849023859 ) ) ;
#21712=CARTESIAN_POINT ( 'NONE',  ( -19.81637295874435978, 31.00000000000000355, -11.44243563873997793 ) ) ;
#21726=CARTESIAN_POINT ( 'NONE',  ( 58.84426737335365232, 31.00000000000000355, 76.69096868241209108 ) ) ;
#21730=CARTESIAN_POINT ( 'NONE',  ( -11.85532105537472880, 40.00000000000000000, -20.54123584193517260 ) ) ;
#21758=CARTESIAN_POINT ( 'NONE',  ( 47.09643503919448193, 31.00000000000000355, 3.164684800459845349 ) ) ;
#21764=EDGE_LOOP ( 'NONE', ( #6633, #17973, #20103, #20153 ) ) ;
#21766=CARTESIAN_POINT ( 'NONE',  ( 52.50410707185378811, 39.99999999999999289, -40.15145572477544533 ) ) ;
#21779=CARTESIAN_POINT ( 'NONE',  ( -69.75709431192164800, 31.00000000000000711, -9.183449035091399537 ) ) ;
#21789=CARTESIAN_POINT ( 'NONE',  ( -26.95034633362163845, 31.00000000000000355, -79.72278128421110921 ) ) ;
#21790=CARTESIAN_POINT ( 'NONE',  ( -41.82916961767931951, 40.00000000000000000, -72.66191475361131324 ) ) ;
#21808=DIRECTION ( 'NONE',  ( 0.000000000000000000, 1.000000000000000000, 0.000000000000000000 ) ) ;
#21815=ORIENTED_EDGE ( 'NONE', *, *, #15639, .T. ) ;
#21818=CARTESIAN_POINT ( 'NONE',  ( -32.09999204393464822, 40.00000000000000000, -2.147948991655045159 ) ) ;
#21823=CARTESIAN_POINT ( 'NONE',  ( -22.00000000000000000, 31.00000000000000355, 0.000000000000000000 ) ) ;
#21828=CARTESIAN_POINT ( 'NONE',  ( -30.97228021248666607, 31.00000000000000355, 23.76985434021725041 ) ) ;
#21834=CARTESIAN_POINT ( 'NONE',  ( 57.37208743749949491, 31.00000000000000355, 50.31438278193533620 ) ) ;
#21837=CARTESIAN_POINT ( 'NONE',  ( -44.44570800417318424, 31.00000000000000355, 25.56477902013656589 ) ) ;
#21839=CARTESIAN_POINT ( 'NONE',  ( 5.726861599741335240, 40.00000000000000000, 87.39583333411552246 ) ) ;
#21854=CARTESIAN_POINT ( 'NONE',  ( -34.23962737045593485, 40.00000000000000000, 59.30561363632230609 ) ) ;
#21859=DIRECTION ( 'NONE',  ( 0.000000000000000000, 1.000000000000000000, 0.000000000000000000 ) ) ;
#21877=CARTESIAN_POINT ( 'NONE',  ( -6.851565232941113415, 31.00000000000000355, -51.95325991929587417 ) ) ;
#21883=CARTESIAN_POINT ( 'NONE',  ( -8.160545988181935328, 40.00000000000000000, -61.88879904071598048 ) ) ;
#21890=CARTESIAN_POINT ( 'NONE',  ( -19.99999999999999645, 31.00000000000000355, 0.000000000000000000 ) ) ;
#21893=CARTESIAN_POINT ( 'NONE',  ( 22.24487986055951083, 40.00000000000000000, 28.98451114863597766 ) ) ;
#21906=PLANE ( 'NONE',  #20961 ) ;
#21908=CARTESIAN_POINT ( 'NONE',  ( -10.54315780145427617, 31.00000000000000355, 79.17709703063970039 ) ) ;
#21917=CARTESIAN_POINT ( 'NONE',  ( -7.718844055051848230, 31.00000000000000355, -22.75659427661714673 ) ) ;
#21929=CARTESIAN_POINT ( 'NONE',  ( 94.59594211465898184, 31.00000000000000000, 12.45590092308117569 ) ) ;
#21933=CARTESIAN_POINT ( 'NONE',  ( 36.56095242094649933, 40.00000000000000000, -4.755136101395176951 ) ) ;
#21961=CARTESIAN_POINT ( 'NONE',  ( 48.78760054486801323, 31.00000000000000355, -28.06521077754944926 ) ) ;
#21967=CARTESIAN_POINT ( 'NONE',  ( -61.81085491475939619, 40.00000000000000711, 35.57109242552864004 ) ) ;
#21979=CARTESIAN_POINT ( 'NONE',  ( 64.89583333437747115, 31.00000000000000000, -4.254240043327834009 ) ) ;
#21987=CARTESIAN_POINT ( 'NONE',  ( 39.23423008409712054, 31.00000000000000355, 79.83814995801117220 ) ) ;
#21988=CARTESIAN_POINT ( 'NONE',  ( -29.11455967534193334, 40.00000000000000000, 85.38284731560057139 ) ) ;
#22006=EDGE_CURVE ( 'NONE', #31505, #33113, #17931, .T. ) ;
#22010=CARTESIAN_POINT ( 'NONE',  ( 15.59370980024835696, 31.00000000000000355, -20.29731371384564653 ) ) ;
#22019=CARTESIAN_POINT ( 'NONE',  ( 36.58905133581346547, 40.00000000000000000, -27.97030060560320308 ) ) ;
#22024=B_SPLINE_CURVE_WITH_KNOTS ( 'NONE', 3,
 ( #3645, #23342, #40519, #14164, #33995, #4084, #13516, #40079, #23775, #3214, #10653, #23990, #17455, #16592, #16805, #13306, #30299, #26808, #36603, #27457, #10217, #37045, #40728, #10882, #39868, #13737, #23563, #36831, #6725, #20089, #17014, #6936, #33353, #27039, #30095, #17242, #20508, #20294, #33558, #40308, #33770, #3856, #30525, #41613, #28343, #31167, #4753, #31588, #8456, #24644, #11971, #28116, #37899, #30940, #1463, #1023, #14374, #1682, #27690, #11314, #8020, #17891, #40954, #15033, #38126, #21818, #34414, #11105, #8249, #1257, #11763, #28560, #24430, #37686, #41163, #21388, #34638, #7807, #18120, #17672, #31813, #31380, #21606, #14817, #4969, #41823, #25093, #41381, #18327, #21164, #37478, #24873, #4518, #11530, #34856, #14604, #35062, #27908, #18539, #38333, #5175, #1900, #15267, #7593, #20949, #34204, #4299, #32024, #26124, #39389, #9301, #12397, #12599, #2102, #35279, #42664, #25720, #32862, #42879, #9528, #18970, #8664, #5813, #32227, #28762, #16096, #28970, #32437, #8891, #22657, #22241, #2941, #42026, #22884, #2302, #36127, #6247, #15466, #25296, #29607, #12811, #19590, #12180, #16303, #25498, #38540, #15670, #35692, #2524, #35489, #38759, #22446, #5607, #2733, #22019, #5401, #18765, #42241, #38971, #29189, #9090, #19169, #15888, #42459, #25917, #39179, #35901, #6035, #19387, #32655, #29395, #3157, #30246, #33505, #3383, #40257, #20674, #13253, #548, #39612, #10157, #19802, #13040, #17403, #13900, #37201, #23933, #23088, #13467, #23726, #27197, #33941, #33071, #9739, #7098, #20454, #20244, #16964, #16533, #6887, #40466, #43100, #23510, #30684, #36989, #314, #26544, #4030, #30044, #9944, #29836, #23293, #13679, #33714, #36545, #36774, #26342, #39816, #36335, #6668, #6453, #26756, #20033, #3591, #33301, #16753, #3801, #94, #40028, #26979, #10388, #7310, #17182, #30470, #10600, #4916, #11055, #21557, #757, #24154, #7542, #37633, #8403, #35016, #7753, #10826, #38284, #37421, #34365, #4694, #11263, #14765, #41110, #11480, #5124, #34805, #31107, #24816, #30889, #18486, #31329, #21115, #31540, #24592, #18276, #40673, #1629, #14981, #27854, #1197, #8196, #7967, #18069, #20899, #37844, #28292, #40900, #21332, #34150, #41328, #11707, #14320, #21766, #17833, #24380, #4251, #4461, #1414, #38071, #14550, #34582, #14115, #17621, #969, #27631, #27406, #28067, #41557, #25044, #31976, #39132, #25872, #38490, #5560, #2253, #8606, #12762, #25667, #31757, #19332, #35847, #41977, #9252, #1851, #11918, #21967, #32602, #25446, #39332, #22824, #38708, #35225, #18919, #25244, #26068, #22605, #32175, #5977, #9471, #15214, #5347, #35644, #18717, #38924, #2053, #28917, #16044, #8831, #2683, #12343, #29345, #15417, #36077, #42613, #6195, #28511, #41774, #42183, #9042, #12126, #28711, #22398, #22188, #35444, #15613, #5761, #19118, #32383, #2469, #15830, #29139, #42408, #12551, #3747, #13201, #44, #6840, #43050, #19979, #12984, #257, #9691, #36720, #39975, #9894, #3541, #27150, #19751, #7047, #2888, #16703, #26285, #19540, #23885, #20403, #491, #30418, #29553, #33248, #30197, #33663, #40414, #39560, #16256, #13629, #26924, #13857, #17129, #10550, #26492, #23244, #36936, #3333, #37150, #32809, #42823, #39766, #13413, #20196, #36493, #29990, #23035, #40203, #36285, #33453, #10104, #6614, #16916, #6404, #33018, #3102, #16476, #29777, #26706, #23460, #10339, #23678, #31492, #18223, #17357, #7697, #18015, #21502, #14927, #14064, #3978, #1364, #14711, #14496, #11214, #27358, #4410, #21067, #37374, #17782, #24989, #31281, #24544, #20854, #28232, #24333, #4197, #10769, #17568, #7917, #28017, #30842, #31054, #20619, #24103, #30638, #7258, #41060, #34315, #702, #27808, #40621, #7486, #41277, #34104, #37587, #1146, #916, #1578, #37798, #33891, #38013, #11426, #14268, #24760, #27575, #8140, #41497, #40849, #11002, #21278, #34527, #4638, #34756, #4862, #11647, #32547, #2409, #38651, #42352, #2633, #8350, #1796, #42128, #25190, #32124, #12710, #25612, #38438, #25394, #8774, #2005, #22551, #8557, #19274, #15775, #5918, #29082, #15996 ),
 .UNSPECIFIED., .F., .F.,
 ( 4, 2, 2, 2, 2, 2, 2, 2, 2, 2, 2, 2, 2, 2, 2, 2, 2, 2, 2, 2, 2, 2, 2, 2, 2, 2, 2, 2, 2, 2, 2, 2, 2, 2, 2, 2, 2, 2, 2, 2, 2, 2, 2, 2, 2, 2, 2, 2, 2, 2, 2, 2, 2, 2, 2, 2, 2, 2, 2, 2, 2, 2, 2, 2, 2, 2, 2, 2, 2, 2, 2, 2, 2, 2, 2, 2, 2, 2, 2, 2, 2, 2, 2, 2, 2, 2, 2, 2, 2, 2, 2, 2, 2, 2, 2, 2, 2, 2, 2, 2, 2, 2, 2, 2, 2, 2, 2, 2, 2, 2, 2, 2, 2, 2, 2, 2, 2, 2, 2, 2, 2, 2, 2, 2, 2, 2, 2, 2, 2, 2, 2, 2, 2, 2, 2, 2, 2, 2, 2, 2, 2, 2, 2, 2, 2, 2, 2, 2, 2, 2, 2, 2, 2, 2, 2, 2, 2, 2, 2, 2, 2, 2, 2, 2, 2, 2, 2, 2, 2, 2, 2, 2, 2, 2, 2, 2, 2, 2, 2, 2, 2, 2, 2, 2, 2, 2, 2, 2, 2, 2, 2, 2, 2, 2, 2, 2, 2, 2, 2, 2, 2, 2, 2, 2, 2, 2, 2, 2, 2, 2, 2, 2, 2, 2, 2, 2, 2, 2, 2, 2, 2, 2, 2, 2, 2, 2, 2, 2, 2, 2, 2, 2, 2, 2, 2, 2, 2, 2, 2, 2, 2, 2, 2, 2, 2, 2, 2, 2, 2, 2, 2, 2, 2, 2, 2, 2, 4 ),
 ( 0.000000000000000000, 0.003906250000000000000, 0.007812500000000000000, 0.01171875000000000000, 0.01562500000000000000, 0.01953125000000000000, 0.02343750000000000000, 0.02734375000000000000, 0.03125000000000000000, 0.03515625000000000000, 0.03906250000000000000, 0.04296875000000000000, 0.04687500000000000000, 0.05078125000000000000, 0.05468750000000000000, 0.05859375000000000000, 0.06250000000000000000, 0.06640625000000000000, 0.07031250000000000000, 0.07421875000000000000, 0.07812500000000000000, 0.08203125000000000000, 0.08593750000000000000, 0.08984375000000000000, 0.09375000000000000000, 0.09765625000000000000, 0.1015625000000000000, 0.1054687500000000000, 0.1093750000000000000, 0.1132812500000000000, 0.1171875000000000000, 0.1210937500000000000, 0.1250000000000000000, 0.1289062500000000000, 0.1328125000000000000, 0.1367187500000000000, 0.1406250000000000000, 0.1445312500000000000, 0.1484375000000000000, 0.1523437500000000000, 0.1562500000000000000, 0.1601562500000000000, 0.1640625000000000000, 0.1679687500000000000, 0.1718750000000000000, 0.1757812500000000000, 0.1796875000000000000, 0.1835937500000000000, 0.1875000000000000000, 0.1914062500000000000, 0.1953125000000000000, 0.1992187500000000000, 0.2031250000000000000, 0.2070312500000000000, 0.2109375000000000000, 0.2148437500000000000, 0.2187500000000000000, 0.2226562500000000000, 0.2265625000000000000, 0.2304687500000000000, 0.2343750000000000000, 0.2382812500000000000, 0.2421875000000000000, 0.2460937500000000000, 0.2500000000000000000, 0.2539062500000000000, 0.2578125000000000000, 0.2617187500000000000, 0.2656250000000000000, 0.2695312500000000000, 0.2734375000000000000, 0.2773437500000000000, 0.2812500000000000000, 0.2851562500000000000, 0.2890625000000000000, 0.2929687500000000000, 0.2968750000000000000, 0.3007812500000000000, 0.3046875000000000000, 0.3085937500000000000, 0.3125000000000000000, 0.3164062500000000000, 0.3203125000000000000, 0.3242187500000000000, 0.3281250000000000000, 0.3320312500000000000, 0.3359375000000000000, 0.3398437500000000000, 0.3437500000000000000, 0.3476562500000000000, 0.3515625000000000000, 0.3554687500000000000, 0.3593750000000000000, 0.3632812500000000000, 0.3671875000000000000, 0.3710937500000000000, 0.3750000000000000000, 0.3789062500000000000, 0.3828125000000000000, 0.3867187500000000000, 0.3906250000000000000, 0.3945312500000000000, 0.3984375000000000000, 0.4023437500000000000, 0.4062500000000000000, 0.4101562500000000000, 0.4140625000000000000, 0.4179687500000000000, 0.4218750000000000000, 0.4257812500000000000, 0.4296875000000000000, 0.4335937500000000000, 0.4375000000000000000, 0.4414062500000000000, 0.4453125000000000000, 0.4492187500000000000, 0.4531250000000000000, 0.4570312500000000000, 0.4609375000000000000, 0.4648437500000000000, 0.4687500000000000000, 0.4726562500000000000, 0.4765625000000000000, 0.4804687500000000000, 0.4843750000000000000, 0.4882812500000000000, 0.4921875000000000000, 0.4960937500000000000, 0.5000000000000000000, 0.5039062500000000000, 0.5078125000000000000, 0.5117187500000000000, 0.5156250000000000000, 0.5195312500000000000, 0.5234375000000000000, 0.5273437500000000000, 0.5312500000000000000, 0.5351562500000000000, 0.5390625000000000000, 0.5429687500000000000, 0.5468750000000000000, 0.5507812500000000000, 0.5546875000000000000, 0.5585937500000000000, 0.5625000000000000000, 0.5664062500000000000, 0.5703125000000000000, 0.5742187500000000000, 0.5781250000000000000, 0.5820312500000000000, 0.5859375000000000000, 0.5898437500000000000, 0.5937500000000000000, 0.5976562500000000000, 0.6015625000000000000, 0.6054687500000000000, 0.6093750000000000000, 0.6132812500000000000, 0.6171875000000000000, 0.6210937500000000000, 0.6250000000000000000, 0.6289062500000000000, 0.6328125000000000000, 0.6367187500000000000, 0.6406250000000000000, 0.6445312500000000000, 0.6484375000000000000, 0.6523437500000000000, 0.6562500000000000000, 0.6601562500000000000, 0.6640625000000000000, 0.6679687500000000000, 0.6718750000000000000, 0.6757812500000000000, 0.6796875000000000000, 0.6835937500000000000, 0.6875000000000000000, 0.6914062500000000000, 0.6953125000000000000, 0.6992187500000000000, 0.7031250000000000000, 0.7070312500000000000, 0.7109375000000000000, 0.7148437500000000000, 0.7187500000000000000, 0.7226562500000000000, 0.7265625000000000000, 0.7304687500000000000, 0.7343750000000000000, 0.7382812500000000000, 0.7421875000000000000, 0.7460937500000000000, 0.7500000000000000000, 0.7539062500000000000, 0.7578125000000000000, 0.7617187500000000000, 0.7656250000000000000, 0.7695312500000000000, 0.7734375000000000000, 0.7773437500000000000, 0.7812500000000000000, 0.7851562500000000000, 0.7890625000000000000, 0.7929687500000000000, 0.7968750000000000000, 0.8007812500000000000, 0.8046875000000000000, 0.8085937500000000000, 0.8125000000000000000, 0.8164062500000000000, 0.8203125000000000000, 0.8242187500000000000, 0.8281250000000000000, 0.8320312500000000000, 0.8359375000000000000, 0.8398437500000000000, 0.8437500000000000000, 0.8476562500000000000, 0.8515625000000000000, 0.8554687500000000000, 0.8593750000000000000, 0.8632812500000000000, 0.8671875000000000000, 0.8710937500000000000, 0.8750000000000000000, 0.8789062500000000000, 0.8828125000000000000, 0.8867187500000000000, 0.8906250000000000000, 0.8945312500000000000, 0.8984375000000000000, 0.9023437500000000000, 0.9062500000000000000, 0.9101562500000000000, 0.9140625000000000000, 0.9179687500000000000, 0.9218750000000000000, 0.9257812500000000000, 0.9296875000000000000, 0.9335937500000000000, 0.9375000000000000000, 0.9414062500000000000, 0.9453125000000000000, 0.9492187500000000000, 0.9531250000000000000, 0.9570312500000000000, 0.9609375000000000000, 0.9648437500000000000, 0.9687500000000000000, 0.9726562500000000000, 0.9765625000000000000, 0.9804687500000000000, 0.9843750000000000000, 0.9882812500000000000, 0.9921875000000000000, 0.9960937500000000000, 1.000000000000000000 ),
 .UNSPECIFIED. ) ;
#22035=CARTESIAN_POINT ( 'NONE',  ( 25.50046184691807483, 31.00000000000000355, -22.37655979312362931 ) ) ;
#22040=ORIENTED_EDGE ( 'NONE', *, *, #2707, .T. ) ;
#22043=CARTESIAN_POINT ( 'NONE',  ( 71.66629920589342362, 31.00000000000000000, 24.32769631419027689 ) ) ;
#22045=CARTESIAN_POINT ( 'NONE',  ( -39.97893566998936166, 31.00000000000000355, -35.18630237794885574 ) ) ;
#22046=CARTESIAN_POINT ( 'NONE',  ( -5.726861599740728614, 40.00000000000000000, 87.60416666588449175 ) ) ;
#22059=CARTESIAN_POINT ( 'NONE',  ( 31.73387399974884104, 40.00000000000000000, -54.96645564127986461 ) ) ;
#22095=CARTESIAN_POINT ( 'NONE',  ( -49.89583333467011528, 31.00000000000000355, 3.272492339034415831 ) ) ;
#22101=CARTESIAN_POINT ( 'NONE',  ( 54.89583333452979730, 40.00000000000000000, -3.599741573803383332 ) ) ;
#22109=CARTESIAN_POINT ( 'NONE',  ( 24.02862666965263116, 40.00000000000000000, 27.38392887651082575 ) ) ;
#22125=CARTESIAN_POINT ( 'NONE',  ( -62.56443097448101298, 31.00000000000000355, -55.02758207457566897 ) ) ;
#22135=CARTESIAN_POINT ( 'NONE',  ( -22.06642698273766356, 31.00000000000000355, -2.901557744773885616 ) ) ;
#22148=CARTESIAN_POINT ( 'NONE',  ( 31.25450476884064699, 31.00000000000000355, 92.02345382966369414 ) ) ;
#22152=CARTESIAN_POINT ( 'NONE',  ( 17.42035916340572399, 40.00000000000000000, 19.85006075799527991 ) ) ;
#22153=CARTESIAN_POINT ( 'NONE',  ( 28.62564328229377608, 40.00000000000000000, -21.88780996305825965 ) ) ;
#22158=ORIENTED_EDGE ( 'NONE', *, *, #23937, .F. ) ;
#22170=AXIS2_PLACEMENT_3D ( 'NONE', #38442, #24546, #35170 ) ;
#22180=CARTESIAN_POINT ( 'NONE',  ( -44.44570800417318424, 31.00000000000000355, 25.56477902013656589 ) ) ;
#22188=CARTESIAN_POINT ( 'NONE',  ( 76.90008882636699639, 39.99999999999999289, -4.923574515426283327 ) ) ;
#22193=EDGE_CURVE ( 'NONE', #33557, #14757, #30936, .T. ) ;
#22202=CARTESIAN_POINT ( 'NONE',  ( -67.35649507452052376, 31.00000000000000711, 18.04843207638801772 ) ) ;
#22213=CARTESIAN_POINT ( 'NONE',  ( 6.309545988805660421, 31.00000000000000355, -94.59213238968112591 ) ) ;
#22214=CARTESIAN_POINT ( 'NONE',  ( 12.87762912549411354, 40.00000000000000000, 98.66289914827740404 ) ) ;
#22234=CARTESIAN_POINT ( 'NONE',  ( 8.075107282080610460, 31.00000000000000355, -23.73893940452553508 ) ) ;
#22241=CARTESIAN_POINT ( 'NONE',  ( -41.92568936861482598, 40.00000000000000000, -5.596851440153165491 ) ) ;
#22255=CARTESIAN_POINT ( 'NONE',  ( 11.92156526682413720, 31.00000000000000355, 35.08788755311113761 ) ) ;
#22261=CARTESIAN_POINT ( 'NONE',  ( 68.41617299536980568, 31.00000000000000000, 52.47886963225217016 ) ) ;
#22265=CARTESIAN_POINT ( 'NONE',  ( 55.55275676652586725, 31.00000000000000355, 14.97830846782891356 ) ) ;
#22266=CARTESIAN_POINT ( 'NONE',  ( 25.17870271038170316, 40.00000000000000000, 93.97695291299892517 ) ) ;
#22278=CARTESIAN_POINT ( 'NONE',  ( -34.66105084696506822, 40.00000000000000000, 70.31756248751102589 ) ) ;
#22306=CARTESIAN_POINT ( 'NONE',  ( 48.10206620145878276, 31.00000000000000355, -42.20136231105875879 ) ) ;
#22312=CARTESIAN_POINT ( 'NONE',  ( -25.79802671946675474, 40.00000000000000000, 52.34090327860478453 ) ) ;
#22318=CARTESIAN_POINT ( 'NONE',  ( 16.30133787010129254, 40.00000000000000000, 33.04822796959624753 ) ) ;
#22328=ADVANCED_FACE ( 'NONE', ( #1009 ), #15017, .T. ) ;
#22334=CARTESIAN_POINT ( 'NONE',  ( -70.49178429274641644, 31.00000000000000711, 40.57739572807859929 ) ) ;
#22339=PLANE ( 'NONE',  #36333 ) ;
#22341=CARTESIAN_POINT ( 'NONE',  ( -22.00000000000000000, 31.00000000000000355, 0.000000000000000000 ) ) ;
#22344=CARTESIAN_POINT ( 'NONE',  ( -1.472621547668719444, 31.00000000000000355, -22.39583333634585571 ) ) ;
#22359=CARTESIAN_POINT ( 'NONE',  ( 13.36968668718156295, 40.00000000000000000, 23.13838826010315941 ) ) ;
#22360=CARTESIAN_POINT ( 'NONE',  ( -41.52979953745317232, 40.00000000000000000, 5.398177843167591305 ) ) ;
#22381=CARTESIAN_POINT ( 'NONE',  ( 12.74197863150380883, 40.00000000000000000, 96.66318596537892915 ) ) ;
#22390=CARTESIAN_POINT ( 'NONE',  ( -51.46673616000524021, 31.00000000000000355, 6.691140578787329041 ) ) ;
#22398=CARTESIAN_POINT ( 'NONE',  ( 76.30724621505197547, 39.99999999999999289, -9.942258256684034734 ) ) ;
#22407=CARTESIAN_POINT ( 'NONE',  ( -41.80404827410195168, 31.00000000000000355, 54.50178954758867889 ) ) ;
#22416=CARTESIAN_POINT ( 'NONE',  ( 25.57473013255608052, 31.00000000000000355, 95.94174708837350352 ) ) ;
#22417=CARTESIAN_POINT ( 'NONE',  ( -80.50242771303932443, 40.00000000000000711, -46.62292012066232871 ) ) ;
#22437=CARTESIAN_POINT ( 'NONE',  ( -6.237032369604345483, 31.00000000000000355, -23.31551866006812190 ) ) ;
#22446=CARTESIAN_POINT ( 'NONE',  ( 27.84166646521873645, 40.00000000000000000, -36.16032403486059366 ) ) ;
#22459=CARTESIAN_POINT ( 'NONE',  ( -38.45388554590046937, 31.00000000000000355, -13.05014827191142679 ) ) ;
#22466=CARTESIAN_POINT ( 'NONE',  ( 46.76839422403993751, 31.00000000000000000, -81.00140361174831583 ) ) ;
#22469=CARTESIAN_POINT ( 'NONE',  ( 54.03410584561684260, 31.00000000000000355, 41.58544482236945328 ) ) ;
#22470=CARTESIAN_POINT ( 'NONE',  ( 52.50410707185378811, 39.99999999999999289, -40.15145572477544533 ) ) ;
#22485=CARTESIAN_POINT ( 'NONE',  ( -59.40286837855683899, 40.00000000000000711, 52.11376356989983805 ) ) ;
#22514=CARTESIAN_POINT ( 'NONE',  ( 31.73387399974884104, 31.00000000000000355, -54.96645564127986461 ) ) ;
#22521=CARTESIAN_POINT ( 'NONE',  ( 34.63398384099731686, 31.00000000000000355, -11.69655689657770203 ) ) ;
#22522=CARTESIAN_POINT ( 'NONE',  ( -8.856203846296160975, 40.00000000000000000, 67.27320953167645712 ) ) ;
#22530=CARTESIAN_POINT ( 'NONE',  ( 23.39270017067629936, 40.00000000000000000, 40.49502024156475244 ) ) ;
#22534=DIRECTION ( 'NONE',  ( 0.000000000000000000, -7.709882115452471264E-16, -1.000000000000000000 ) ) ;
#22544=CARTESIAN_POINT ( 'NONE',  ( 82.09539989324809994, 31.00000000000000000, -27.75477508811727390 ) ) ;
#22551=CARTESIAN_POINT ( 'NONE',  ( -87.85203729262056527, 40.00000000000000711, 50.59313708112332364 ) ) ;
#22558=CARTESIAN_POINT ( 'NONE',  ( -24.68525358734468611, 31.00000000000000355, -18.92943107747915832 ) ) ;
#22565=CARTESIAN_POINT ( 'NONE',  ( 39.78947517253659072, 40.00000000000000000, -19.62497191778171413 ) ) ;
#22566=CARTESIAN_POINT ( 'NONE',  ( 36.89914868738106435, 40.00000000000000000, -2.354335741662294978 ) ) ;
#22573=EDGE_CURVE ( 'NONE', #3181, #29181, #11516, .T. ) ;
#22589=CARTESIAN_POINT ( 'NONE',  ( 48.45023387855729879, 40.00000000000000000, 83.88660019351674180 ) ) ;
#22597=CARTESIAN_POINT ( 'NONE',  ( -22.33566874673848091, 31.00000000000000355, 45.10700316349001326 ) ) ;
#22605=CARTESIAN_POINT ( 'NONE',  ( -65.32047834219908111, 40.00000000000000711, -32.32491738442255524 ) ) ;
#22617=CARTESIAN_POINT ( 'NONE',  ( -51.96644965834242669, 31.00000000000000711, 59.25555446696338890 ) ) ;
#22629=CARTESIAN_POINT ( 'NONE',  ( -13.16936484334534008, 31.00000000000000355, 99.04657264463375554 ) ) ;
#22630=CARTESIAN_POINT ( 'NONE',  ( 43.66223835209735427, 40.00000000000000000, 88.82794485019093145 ) ) ;
#22638=CARTESIAN_POINT ( 'NONE',  ( -15.99999999999997691, 31.00000000000000355, 5.571627607371296764E-15 ) ) ;
#22647=CARTESIAN_POINT ( 'NONE',  ( 6.473670811831355287, 31.00000000000000355, -24.11571013580713441 ) ) ;
#22657=CARTESIAN_POINT ( 'NONE',  ( -42.09738266246711902, 40.00000000000000000, -2.828681863544772135 ) ) ;
#22667=CARTESIAN_POINT ( 'NONE',  ( 34.94781834021004840, 31.00000000000000355, -26.81980329959834108 ) ) ;
#22674=CARTESIAN_POINT ( 'NONE',  ( -54.00384411200708712, 31.00000000000000711, 70.40394205939183792 ) ) ;
#22678=CARTESIAN_POINT ( 'NONE',  ( 32.82854187708761629, 31.00000000000000355, -56.64543409046200395 ) ) ;
#22679=CARTESIAN_POINT ( 'NONE',  ( 8.570044366896553356, 40.00000000000000000, -64.27561742002654910 ) ) ;
#22693=CARTESIAN_POINT ( 'NONE',  ( 71.66629920589342362, 39.99999999999999289, 24.32769631419027689 ) ) ;
#22724=CARTESIAN_POINT ( 'NONE',  ( -59.89583333444493718, 31.00000000000000711, 3.926990808566372060 ) ) ;
#22727=CARTESIAN_POINT ( 'NONE',  ( 36.56095242095437925, 31.00000000000000355, -4.755136101395175174 ) ) ;
#22729=CARTESIAN_POINT ( 'NONE',  ( 62.17703816010947548, 39.99999999999999289, 21.10553973064489597 ) ) ;
#22740=CARTESIAN_POINT ( 'NONE',  ( 44.89583333484414140, 40.00000000000000000, -2.945243104263157274 ) ) ;
#22752=CARTESIAN_POINT ( 'NONE',  ( 83.51212062385671686, 31.00000000000000000, -48.08891344041042970 ) ) ;
#22774=AXIS2_PLACEMENT_3D ( 'NONE', #28331, #4509, #24636 ) ;
#22775=CARTESIAN_POINT ( 'NONE',  ( 26.99674208481366833, 31.00000000000000355, -20.71990538090019029 ) ) ;
#22782=CARTESIAN_POINT ( 'NONE',  ( -19.20510714644778361, 40.00000000000000000, 33.27066566623395261 ) ) ;
#22783=CARTESIAN_POINT ( 'NONE',  ( 5.076274692535532651, 40.00000000000000000, 39.04542013319162663 ) ) ;
#22816=CARTESIAN_POINT ( 'NONE',  ( 56.89991739620084132, 31.00000000000000355, -3.630084216720528278 ) ) ;
#22824=CARTESIAN_POINT ( 'NONE',  ( -71.33925323115938966, 40.00000000000000711, 9.290813765102964084 ) ) ;
#22839=CARTESIAN_POINT ( 'NONE',  ( 10.12401712103624263, 31.00000000000000355, 76.79210772277129138 ) ) ;
#22852=CARTESIAN_POINT ( 'NONE',  ( 77.87745995352098305, 31.00000000000000000, 59.89653754214596404 ) ) ;
#22853=CARTESIAN_POINT ( 'NONE',  ( 47.87658044100083288, 39.99999999999999289, -82.67148682534872250 ) ) ;
#22870=LINE ( 'NONE', #19580, #20846 ) ;
#22873=CARTESIAN_POINT ( 'NONE',  ( -18.31940394017777507, 31.00000000000000355, -14.05611420671224288 ) ) ;
#22884=CARTESIAN_POINT ( 'NONE',  ( -38.37160831358556123, 40.00000000000000000, -19.00137192356237392 ) ) ;
#22895=CARTESIAN_POINT ( 'NONE',  ( -16.75480014238754478, 31.00000000000000355, -49.32177912249007790 ) ) ;
#22903=CARTESIAN_POINT ( 'NONE',  ( 91.55691129138550366, 31.00000000000000000, -24.53049628908797430 ) ) ;
#22909=CARTESIAN_POINT ( 'NONE',  ( 66.37122006405570573, 31.00000000000000000, -8.639838683444628131 ) ) ;
#22910=CARTESIAN_POINT ( 'NONE',  ( 57.47007747233163144, 39.99999999999999289, -33.06854485814638878 ) ) ;
#22921=CARTESIAN_POINT ( 'NONE',  ( 38.42722039544141666, 40.00000000000000000, 66.52996821281629991 ) ) ;
#22952=CARTESIAN_POINT ( 'NONE',  ( -18.68892229297488683, 31.00000000000000355, 55.06009237583231197 ) ) ;
#22956=CARTESIAN_POINT ( 'NONE',  ( -2.197745971918068530, 31.00000000000000355, -34.39891587002171036 ) ) ;
#22957=CARTESIAN_POINT ( 'NONE',  ( 49.83821931962687302, 40.00000000000000000, 43.70611527624207326 ) ) ;
#22958=AXIS2_PLACEMENT_3D ( 'NONE', #26046, #35423, #2037 ) ;
#22964=CARTESIAN_POINT ( 'NONE',  ( 12.21457428495364006, 40.00000000000000000, 45.57612047952555656 ) ) ;
#22978=CARTESIAN_POINT ( 'NONE',  ( 77.87745995352098305, 31.00000000000000000, 59.89653754214596404 ) ) ;
#22995=CARTESIAN_POINT ( 'NONE',  ( 16.69935377588158332, 31.00000000000000355, -28.93150767131472989 ) ) ;
#23001=CARTESIAN_POINT ( 'NONE',  ( 24.02862666965263116, 40.00000000000000000, 27.38392887651082575 ) ) ;
#23002=CARTESIAN_POINT ( 'NONE',  ( -38.37160831358556123, 40.00000000000000000, -19.00137192356237392 ) ) ;
#23028=CARTESIAN_POINT ( 'NONE',  ( -8.314562429035724733, 31.00000000000000355, -63.88718494334916187 ) ) ;
#23035=CARTESIAN_POINT ( 'NONE',  ( 74.83201185296370284, 39.99999999999999289, -43.08100868844128684 ) ) ;
#23048=CARTESIAN_POINT ( 'NONE',  ( 60.46509673945340779, 31.00000000000000000, 46.37897171330492085 ) ) ;
#23059=CARTESIAN_POINT ( 'NONE',  ( -55.31949386280458469, 31.00000000000000711, 71.91600076666669850 ) ) ;
#23060=CARTESIAN_POINT ( 'NONE',  ( 87.78546986784174067, 39.99999999999999289, 43.41392487578124815 ) ) ;
#23080=CARTESIAN_POINT ( 'NONE',  ( 34.63398384099731686, 31.00000000000000355, -11.69655689657770203 ) ) ;
#23088=CARTESIAN_POINT ( 'NONE',  ( -44.44570800418432555, 40.00000000000000000, 25.56477902013099524 ) ) ;
#23094=LINE ( 'NONE', #19594, #8124 ) ;
#23095=CIRCLE ( 'NONE', #4222, 2.500000000000002665 ) ;
#23103=CARTESIAN_POINT ( 'NONE',  ( -32.14164714139042189, 31.00000000000000355, 36.65395011347077059 ) ) ;
#23108=CARTESIAN_POINT ( 'NONE',  ( -70.72766149062127283, 31.00000000000000711, 54.26934393422349956 ) ) ;
#23113=CARTESIAN_POINT ( 'NONE',  ( -61.40313508884858607, 31.00000000000000711, 7.989450542815522027 ) ) ;
#23114=CARTESIAN_POINT ( 'NONE',  ( 65.23019871244166268, 39.99999999999999289, 17.57949444736078703 ) ) ;
#23127=CARTESIAN_POINT ( 'NONE',  ( -9.469526743414824921, 40.00000000000000000, -71.82433816204535049 ) ) ;
#23154=CARTESIAN_POINT ( 'NONE',  ( -59.40491426035100631, 31.00000000000000711, 7.833300799371349932 ) ) ;
#23160=CARTESIAN_POINT ( 'NONE',  ( -5.264430561742837078, 31.00000000000000355, 39.44269128747090747 ) ) ;
#23164=CARTESIAN_POINT ( 'NONE',  ( 62.51641183113888900, 39.99999999999999289, -16.75201923384928548 ) ) ;
#23171=CARTESIAN_POINT ( 'NONE',  ( -39.95047694894377344, 40.00000000000000000, -5.256506769647570465 ) ) ;
#23180=VECTOR ( 'NONE', #37268, 1000.000000000000000 ) ;
#23185=CARTESIAN_POINT ( 'NONE',  ( 72.29027477042623673, 31.00000000000000000, -63.25088587033864229 ) ) ;
#23189=DIRECTION ( 'NONE',  ( 0.000000000000000000, 0.000000000000000000, 1.000000000000000000 ) ) ;
#23190=DIRECTION ( 'NONE',  ( 0.000000000000000000, 0.000000000000000000, 1.000000000000000000 ) ) ;
#23200=CARTESIAN_POINT ( 'NONE',  ( -26.30698076681265363, 31.00000000000000355, 12.97770382244945253 ) ) ;
#23208=CARTESIAN_POINT ( 'NONE',  ( -36.61132647064156487, 40.00000000000000000, -18.04288060775211378 ) ) ;
#23209=CARTESIAN_POINT ( 'NONE',  ( -51.46673615999394968, 40.00000000000000000, 6.691140578787329041 ) ) ;
#23237=CARTESIAN_POINT ( 'NONE',  ( 66.37122006405570573, 31.00000000000000000, -8.639838683444628131 ) ) ;
#23241=CARTESIAN_POINT ( 'NONE',  ( -101.9145453900123641, 17.11489954122026447, -1.407535261550449501 ) ) ;
#23244=CARTESIAN_POINT ( 'NONE',  ( -5.410573124821300262, 40.00000000000000000, -84.40011308931431699 ) ) ;
#23254=CARTESIAN_POINT ( 'NONE',  ( 19.99305134020393382, 31.00000000000000355, 74.61661993947731730 ) ) ;
#23284=CARTESIAN_POINT ( 'NONE',  ( 19.31996883370903362, 31.00000000000000355, 33.58758284028576924 ) ) ;
#23293=CARTESIAN_POINT ( 'NONE',  ( 14.32751628686350287, 40.00000000000000000, -53.13354968558886071 ) ) ;
#23303=CARTESIAN_POINT ( 'NONE',  ( 36.61186797162192619, 31.00000000000000355, 28.07927795628900469 ) ) ;
#23309=EDGE_LOOP ( 'NONE', ( #42535, #30048, #25835, #24610 ) ) ;
#23310=CARTESIAN_POINT ( 'NONE',  ( -89.22528799552154055, 31.00000000000000711, 43.99828826784794700 ) ) ;
#23314=CARTESIAN_POINT ( 'NONE',  ( 63.11376326756305843, 31.00000000000000000, -21.32174659671377626 ) ) ;
#23315=CARTESIAN_POINT ( 'NONE',  ( -16.51797447735934199, 40.00000000000000000, -62.05742538352703974 ) ) ;
#23332=CARTESIAN_POINT ( 'NONE',  ( 82.68608547523962216, 39.99999999999999289, 22.14036602612658200 ) ) ;
#23342=CARTESIAN_POINT ( 'NONE',  ( -22.10416666678001718, 40.00000000000000000, -1.441157586896875564 ) ) ;
#23350=ORIENTED_EDGE ( 'NONE', *, *, #20424, .F. ) ;
#23351=CARTESIAN_POINT ( 'NONE',  ( -105.9879088449591933, 17.11489954122026447, 4.119280070842334496 ) ) ;
#23361=CARTESIAN_POINT ( 'NONE',  ( 55.63593431947571588, 31.00000000000000000, -48.80962981700470493 ) ) ;
#23363=CARTESIAN_POINT ( 'NONE',  ( 15.66220904948440662, 31.00000000000000355, -31.63873590539992264 ) ) ;
#23364=CARTESIAN_POINT ( 'NONE',  ( -62.26029918285335896, 40.00000000000000711, 30.70375207684418228 ) ) ;
#23374=CARTESIAN_POINT ( 'NONE',  ( 55.10416666547021691, 40.00000000000000000, 3.599741573803287853 ) ) ;
#23389=CARTESIAN_POINT ( 'NONE',  ( 96.17895579821514218, 31.00000000000000000, -12.55124642863780515 ) ) ;
#23409=CARTESIAN_POINT ( 'NONE',  ( 24.60508655230852781, 31.00000000000000355, 6.583411914924224284 ) ) ;
#23417=CARTESIAN_POINT ( 'NONE',  ( -40.10416666498607441, 40.00000000000000000, -2.617993869485698344 ) ) ;
#23418=CARTESIAN_POINT ( 'NONE',  ( 15.70068437845367093, 40.00000000000000000, 46.50252577712053892 ) ) ;
#23447=CARTESIAN_POINT ( 'NONE',  ( 28.99662776679064891, 31.00000000000000355, -58.58186007941694129 ) ) ;
#23459=ORIENTED_EDGE ( 'NONE', *, *, #4195, .T. ) ;
#23460=CARTESIAN_POINT ( 'NONE',  ( 66.32976035609178211, 39.99999999999999289, 58.33333674018342663 ) ) ;
#23469=CARTESIAN_POINT ( 'NONE',  ( -59.40286837853895463, 31.00000000000000711, 52.11376356991771530 ) ) ;
#23476=CIRCLE ( 'NONE', #33187, 1.999999999999998668 ) ;
#23496=CARTESIAN_POINT ( 'NONE',  ( -15.99999999999997691, 31.00000000000000355, 5.571627607371296764E-15 ) ) ;
#23501=CARTESIAN_POINT ( 'NONE',  ( 36.56095242095437925, 31.00000000000000355, -4.755136101395175174 ) ) ;
#23510=CARTESIAN_POINT ( 'NONE',  ( -32.53655534684257589, 40.00000000000000000, -42.55839752837238166 ) ) ;
#23525=CARTESIAN_POINT ( 'NONE',  ( 12.21457428495364006, 31.00000000000000355, 45.57612047952555656 ) ) ;
#23530=CARTESIAN_POINT ( 'NONE',  ( 72.43982367323130234, 31.00000000000000000, 63.53091779346544143 ) ) ;
#23534=CARTESIAN_POINT ( 'NONE',  ( -44.72205690102930475, 31.00000000000000355, -58.47036224961646411 ) ) ;
#23535=CARTESIAN_POINT ( 'NONE',  ( -58.00742674161275403, 40.00000000000000711, -44.63796826977546317 ) ) ;
#23551=CARTESIAN_POINT ( 'NONE',  ( 81.87674480462379734, 39.99999999999999289, -21.93767060400471891 ) ) ;
#23555=DIRECTION ( 'NONE',  ( 0.000000000000000000, -1.000000000000000000, 5.297542245118643184E-16 ) ) ;
#23558=ADVANCED_FACE ( 'NONE', ( #1563 ), #18417, .T. ) ;
#23563=CARTESIAN_POINT ( 'NONE',  ( 20.65150112226537260, 40.00000000000000000, -15.81946110361252877 ) ) ;
#23567=DIRECTION ( 'NONE',  ( -1.000000000000000000, 0.000000000000000000, 0.000000000000000000 ) ) ;
#23586=CARTESIAN_POINT ( 'NONE',  ( -54.82550897924149069, 31.00000000000000711, 42.06954809655981364 ) ) ;
#23589=CARTESIAN_POINT ( 'NONE',  ( -21.81649963859176822, 31.00000000000000355, -37.93159502954523532 ) ) ;
#23590=CARTESIAN_POINT ( 'NONE',  ( 50.46169669344906339, 40.00000000000000000, 57.51940134901310131 ) ) ;
#23604=CARTESIAN_POINT ( 'NONE',  ( 48.77780477658175329, 40.00000000000000000, -24.05648398140741406 ) ) ;
#23619=CARTESIAN_POINT ( 'NONE',  ( 6.309545988805660421, 31.00000000000000355, -94.59213238968112591 ) ) ;
#23638=CARTESIAN_POINT ( 'NONE',  ( 19.15075862373047144, 31.00000000000000355, -38.85840887180553693 ) ) ;
#23644=CARTESIAN_POINT ( 'NONE',  ( 39.77940265867437120, 40.00000000000000000, 22.96373720238702276 ) ) ;
#23645=CARTESIAN_POINT ( 'NONE',  ( -11.35616125661516307, 40.00000000000000000, -42.69191301636733726 ) ) ;
#23649=EDGE_CURVE ( 'NONE', #42330, #38968, #10432, .T. ) ;
#23653=CARTESIAN_POINT ( 'NONE',  ( 24.89583333603155069, 40.00000000000000000, -1.636246165087041016 ) ) ;
#23659=VECTOR ( 'NONE', #8008, 1000.000000000000114 ) ;
#23671=CARTESIAN_POINT ( 'NONE',  ( -48.52617905695110068, 31.00000000000000355, 37.10499320822106029 ) ) ;
#23678=CARTESIAN_POINT ( 'NONE',  ( 53.86549405311984628, 40.00000000000000000, 70.40131829845091715 ) ) ;
#23688=CARTESIAN_POINT ( 'NONE',  ( 41.75688748258168914, 31.00000000000000355, -72.32308762158416471 ) ) ;
#23691=ORIENTED_EDGE ( 'NONE', *, *, #3610, .T. ) ;
#23718=CARTESIAN_POINT ( 'NONE',  ( 36.89914868738900822, 31.00000000000000355, -2.354335741662294534 ) ) ;
#23726=CARTESIAN_POINT ( 'NONE',  ( -48.87578956996785706, 40.00000000000000000, 16.50293044077288940 ) ) ;
#23728=CARTESIAN_POINT ( 'NONE',  ( -105.9879088449591933, 31.00000000000000355, 2.119280070842335384 ) ) ;
#23734=CARTESIAN_POINT ( 'NONE',  ( -8.160545988181935328, 31.00000000000000355, -61.88879904071598048 ) ) ;
#23739=CARTESIAN_POINT ( 'NONE',  ( 94.59594211465898184, 31.00000000000000000, 12.45590092308117569 ) ) ;
#23745=CARTESIAN_POINT ( 'NONE',  ( -19.10382689932575673, 31.00000000000000355, -71.73905014346600240 ) ) ;
#23746=CARTESIAN_POINT ( 'NONE',  ( -36.82253293460209420, 40.00000000000000000, -63.98115709648401150 ) ) ;
#23762=CARTESIAN_POINT ( 'NONE',  ( 11.43299787627070607, 40.00000000000000000, 86.72764684403134083 ) ) ;
#23775=CARTESIAN_POINT ( 'NONE',  ( -17.43724119492421565, 40.00000000000000000, -15.29674861594511803 ) ) ;
#23789=CARTESIAN_POINT ( 'NONE',  ( -14.11622541012940601, 31.00000000000000355, -16.08312669853564358 ) ) ;
#23795=CARTESIAN_POINT ( 'NONE',  ( -60.02123122004734768, 31.00000000000000711, 34.66859033927303813 ) ) ;
#23797=CARTESIAN_POINT ( 'NONE',  ( -41.03896728213481992, 31.00000000000000355, -11.06873348903806864 ) ) ;
#23799=CARTESIAN_POINT ( 'NONE',  ( 55.27058341129635721, 39.99999999999999289, -63.02248852588876105 ) ) ;
#23812=CARTESIAN_POINT ( 'NONE',  ( -25.89845354150052259, 40.00000000000000000, -44.83417823681238445 ) ) ;
#23817=EDGE_CURVE ( 'NONE', #27469, #31476, #35053, .T. ) ;
#23842=ORIENTED_EDGE ( 'NONE', *, *, #16267, .T. ) ;
#23845=CARTESIAN_POINT ( 'NONE',  ( 39.78947517253659072, 31.00000000000000355, -19.62497191778171413 ) ) ;
#23851=CARTESIAN_POINT ( 'NONE',  ( -6.851565232941113415, 40.00000000000000000, -51.95325991929587417 ) ) ;
#23852=CARTESIAN_POINT ( 'NONE',  ( 41.62382930722196051, 40.00000000000000000, -20.43270582883756248 ) ) ;
#23860=CARTESIAN_POINT ( 'NONE',  ( 7.411374251232441424, 40.00000000000000000, -21.84767871671174788 ) ) ;
#23879=CARTESIAN_POINT ( 'NONE',  ( -45.90931453311223720, 31.00000000000000355, 40.13788153756826915 ) ) ;
#23885=CARTESIAN_POINT ( 'NONE',  ( -81.27520743796613090, 40.00000000000000711, 10.59408403753070083 ) ) ;
#23898=CARTESIAN_POINT ( 'NONE',  ( -85.90019077458921970, 31.00000000000000711, -29.16093118951848240 ) ) ;
#23925=CARTESIAN_POINT ( 'NONE',  ( -16.82630558382797403, 31.00000000000000355, -29.24196894321154971 ) ) ;
#23933=CARTESIAN_POINT ( 'NONE',  ( -40.56882557769177566, 40.00000000000000000, 31.01417895415859505 ) ) ;
#23937=EDGE_CURVE ( 'NONE', #5066, #36133, #1838, .T. ) ;
#23947=CARTESIAN_POINT ( 'NONE',  ( -7.547223091130065953, 31.00000000000000355, 57.33767041057931380 ) ) ;
#23953=CARTESIAN_POINT ( 'NONE',  ( -6.381360069252544953, 31.00000000000000355, 97.60416666604666602 ) ) ;
#23958=CARTESIAN_POINT ( 'NONE',  ( -32.59403919554602425, 31.00000000000000355, -66.35267222981636337 ) ) ;
#23959=CARTESIAN_POINT ( 'NONE',  ( 20.39742982868580157, 40.00000000000000000, 76.57971376067894198 ) ) ;
#23977=CARTESIAN_POINT ( 'NONE',  ( -66.93673649651354651, 40.00000000000000711, 58.72203107584222437 ) ) ;
#23990=CARTESIAN_POINT ( 'NONE',  ( -11.85532105537472880, 40.00000000000000000, -20.54123584193517260 ) ) ;
#23994=EDGE_CURVE ( 'NONE', #31505, #29860, #42349, .T. ) ;
#24004=CARTESIAN_POINT ( 'NONE',  ( -23.46968090759046888, 31.00000000000000355, -20.57717900685300449 ) ) ;
#24010=CARTESIAN_POINT ( 'NONE',  ( 44.85399723358655422, 31.00000000000000355, -58.47732767552992073 ) ) ;
#24014=CARTESIAN_POINT ( 'NONE',  ( -22.33566874673848091, 31.00000000000000355, 45.10700316349001326 ) ) ;
#24016=CARTESIAN_POINT ( 'NONE',  ( -59.40286837855683899, 40.00000000000000711, 52.11376356989983805 ) ) ;
#24026=CARTESIAN_POINT ( 'NONE',  ( -38.74991464700507748, 40.00000000000000000, 44.18781823130588293 ) ) ;
#24028=COLOUR_RGB ( '', 0.08235294, 0.09019608, 0.10196078) ;
#24037=CIRCLE ( 'NONE', #37918, 4.500000000000000888 ) ;
#24058=CARTESIAN_POINT ( 'NONE',  ( 9.621748599878955588, 31.00000000000000355, 35.89595399306684698 ) ) ;
#24066=CARTESIAN_POINT ( 'NONE',  ( 3.436116956419347002, 40.00000000000000000, -52.60416666537189911 ) ) ;
#24068=CARTESIAN_POINT ( 'NONE',  ( -62.09442273004785307, 40.00000000000000711, -4.163950221635984938 ) ) ;
#24078=CARTESIAN_POINT ( 'NONE',  ( -9.022452542771789652, 40.00000000000000000, 26.59230923919664491 ) ) ;
#24087=DIRECTION ( 'NONE',  ( 0.000000000000000000, 1.000000000000000000, 0.000000000000000000 ) ) ;
#24088=ORIENTED_EDGE ( 'NONE', *, *, #19160, .T. ) ;
#24093=CARTESIAN_POINT ( 'NONE',  ( 68.60033760563639760, 31.00000000000000000, -33.70054013428169526 ) ) ;
#24103=CARTESIAN_POINT ( 'NONE',  ( -46.83686391397709770, 40.00000000000000000, -81.34213072392142863 ) ) ;
#24115=CARTESIAN_POINT ( 'NONE',  ( 82.68608547523962216, 31.00000000000000000, 22.14036602612658200 ) ) ;
#24124=AXIS2_PLACEMENT_3D ( 'NONE', #38656, #25399, #18020 ) ;
#24147=CARTESIAN_POINT ( 'NONE',  ( 38.14553738579559905, 31.00000000000000355, 29.36968266378863746 ) ) ;
#24148=CARTESIAN_POINT ( 'NONE',  ( -105.3367680159044966, 17.11489954122026447, 2.032994142711228136 ) ) ;
#24154=CARTESIAN_POINT ( 'NONE',  ( 7.664524495375378166, 40.00000000000000000, 58.91906827748253050 ) ) ;
#24170=CARTESIAN_POINT ( 'NONE',  ( 53.64558601427197004, 31.00000000000000355, 14.36188897069615500 ) ) ;
#24178=CARTESIAN_POINT ( 'NONE',  ( -18.63466726053507472, 40.00000000000000000, -9.179856479542758407 ) ) ;
#24182=CARTESIAN_POINT ( 'NONE',  ( -5.321195512787073589, 31.00000000000000355, 79.59297073838583003 ) ) ;
#24183=CARTESIAN_POINT ( 'NONE',  ( -64.43604943162229404, 40.00000000000000711, 49.29347324003091302 ) ) ;
#24203=CARTESIAN_POINT ( 'NONE',  ( -36.24314215638268877, 40.00000000000000000, -73.49571118816069770 ) ) ;
#24228=CARTESIAN_POINT ( 'NONE',  ( -12.50349052776452297, 31.00000000000000355, 25.37591446456323041 ) ) ;
#24236=CARTESIAN_POINT ( 'NONE',  ( -69.34045338167970840, 31.00000000000000711, 9.142281554609933636 ) ) ;
#24241=CARTESIAN_POINT ( 'NONE',  ( 34.59698569360211451, 31.00000000000000355, -30.23997570423561498 ) ) ;
#24242=CARTESIAN_POINT ( 'NONE',  ( 66.75212336275305347, 39.99999999999999289, -51.21939497476837744 ) ) ;
#24256=CARTESIAN_POINT ( 'NONE',  ( -40.58740609958903889, 40.00000000000000000, -31.12922691583434798 ) ) ;
#24276=FACE_OUTER_BOUND ( 'NONE', #38749, .T. ) ;
#24288=CARTESIAN_POINT ( 'NONE',  ( 16.30133787010129254, 31.00000000000000355, 33.04822796959624753 ) ) ;
#24296=CARTESIAN_POINT ( 'NONE',  ( 44.91824650936478491, 40.00000000000000000, 5.910997147197376123 ) ) ;
#24298=CARTESIAN_POINT ( 'NONE',  ( 56.89991739620084843, 40.00000000000000000, -3.630084216720919521 ) ) ;
#24310=CARTESIAN_POINT ( 'NONE',  ( 19.04566582976364941, 40.00000000000000000, -14.62000746238684989 ) ) ;
#24318=LINE ( 'NONE', #21263, #36798 ) ;
#24324=CARTESIAN_POINT ( 'NONE',  ( -61.81085491475939619, 31.00000000000000711, 35.57109242551294415 ) ) ;
#24333=CARTESIAN_POINT ( 'NONE',  ( -91.59543978412355614, 40.00000000000000711, -12.18496625897608254 ) ) ;
#24344=CARTESIAN_POINT ( 'NONE',  ( -89.89583333403318477, 31.00000000000000711, 5.890486217120591839 ) ) ;
#24347=CARTESIAN_POINT ( 'NONE',  ( 15.59370980024836051, 40.00000000000000000, -20.29731371384565364 ) ) ;
#24374=CARTESIAN_POINT ( 'NONE',  ( 31.88898475263450649, 31.00000000000000355, 36.48290236124523744 ) ) ;
#24380=CARTESIAN_POINT ( 'NONE',  ( 59.60939625460783731, 39.99999999999999289, -29.27517545779414831 ) ) ;
#24394=CARTESIAN_POINT ( 'NONE',  ( 34.44467569804516671, 31.00000000000000355, 44.88666365967159777 ) ) ;
#24400=CARTESIAN_POINT ( 'NONE',  ( -23.02120395722396395, 40.00000000000000000, 17.66995642160909696 ) ) ;
#24404=CARTESIAN_POINT ( 'NONE',  ( 76.30724621508588257, 31.00000000000000000, -9.942258256679791018 ) ) ;
#24405=CARTESIAN_POINT ( 'NONE',  ( 74.90833963778730720, 39.99999999999999289, 20.17845691863183077 ) ) ;
#24407=ADVANCED_FACE ( 'NONE', ( #9997 ), #38283, .T. ) ;
#24420=CARTESIAN_POINT ( 'NONE',  ( 12.12865573427490062, 40.00000000000000000, -92.11205733446308841 ) ) ;
#24430=CARTESIAN_POINT ( 'NONE',  ( -24.93870012979089168, 40.00000000000000000, -21.94074674037796058 ) ) ;
#24443=CARTESIAN_POINT ( 'NONE',  ( -25.30796725786148826, 31.00000000000000355, 14.62256337265529815 ) ) ;
#24451=CARTESIAN_POINT ( 'NONE',  ( -39.25113411183426848, 31.00000000000000355, 67.98392962655870519 ) ) ;
#24454=CARTESIAN_POINT ( 'NONE',  ( -40.27082278477694643, 31.00000000000000355, 10.71261860272906397 ) ) ;
#24455=CARTESIAN_POINT ( 'NONE',  ( -71.24862878704732339, 40.00000000000000711, 35.13526414049667324 ) ) ;
#24462=ORIENTED_EDGE ( 'NONE', *, *, #32426, .T. ) ;
#24468=CARTESIAN_POINT ( 'NONE',  ( 17.40022565512299479, 40.00000000000000000, 64.93645345284011228 ) ) ;
#24503=CARTESIAN_POINT ( 'NONE',  ( -20.88694679984194380, 31.00000000000000355, -36.15586224631631751 ) ) ;
#24513=CARTESIAN_POINT ( 'NONE',  ( -46.94946386092573221, 40.00000000000000000, 15.94926099647653928 ) ) ;
#24514=CARTESIAN_POINT ( 'NONE',  ( -39.97893566998936876, 40.00000000000000000, -35.18630237794886995 ) ) ;
#24521=CARTESIAN_POINT ( 'NONE',  ( -29.59829689555773058, 40.00000000000000000, 3.906358533625565954 ) ) ;
#24536=CARTESIAN_POINT ( 'NONE',  ( 77.09314031436156256, 31.00000000000000000, 5.156213784760050878 ) ) ;
#24544=CARTESIAN_POINT ( 'NONE',  ( -91.21105805184879500, 40.00000000000000711, 11.89862498596346718 ) ) ;
#24546=DIRECTION ( 'NONE',  ( 1.000000000000000000, 0.000000000000000000, 0.000000000000000000 ) ) ;
#24557=CARTESIAN_POINT ( 'NONE',  ( 73.03870520561201829, 31.00000000000000000, -42.18585045165268355 ) ) ;
#24560=CARTESIAN_POINT ( 'NONE',  ( -20.28213647683248766, 40.00000000000000000, 23.06128528321566051 ) ) ;
#24585=CARTESIAN_POINT ( 'NONE',  ( 40.10317558968866081, 31.00000000000000355, -23.06553963618950931 ) ) ;
#24592=CARTESIAN_POINT ( 'NONE',  ( -50.06114249711410480, 40.00000000000000000, -38.53249520213266521 ) ) ;
#24604=CARTESIAN_POINT ( 'NONE',  ( 18.36587843422771016, 31.00000000000000355, 54.06640964556338957 ) ) ;
#24610=ORIENTED_EDGE ( 'NONE', *, *, #19160, .F. ) ;
#24611=CARTESIAN_POINT ( 'NONE',  ( -2.127120017302697619, 40.00000000000000000, -32.39583333539214038 ) ) ;
#24616=CARTESIAN_POINT ( 'NONE',  ( -60.98551593175036345, 31.00000000000000711, 53.34359504441579247 ) ) ;
#24617=CARTESIAN_POINT ( 'NONE',  ( -5.410573124821300262, 40.00000000000000000, -84.40011308931431699 ) ) ;
#24628=CARTESIAN_POINT ( 'NONE',  ( -20.39032260654148132, 17.11489954122026447, 1.150830359615497844 ) ) ;
#24631=CARTESIAN_POINT ( 'NONE',  ( -25.38139813252123034, 40.00000000000000000, 94.78629358389331117 ) ) ;
#24634=VECTOR ( 'NONE', #18132, 1000.000000000000000 ) ;
#24636=DIRECTION ( 'NONE',  ( 0.000000000000000000, -7.709882115452474222E-16, -1.000000000000000000 ) ) ;
#24644=CARTESIAN_POINT ( 'NONE',  ( -1.974796425974089331, 40.00000000000000000, 29.60085432090885149 ) ) ;
#24656=CARTESIAN_POINT ( 'NONE',  ( 24.63052733448982323, 31.00000000000000355, -3.251868155982907904 ) ) ;
#24663=CARTESIAN_POINT ( 'NONE',  ( 75.74279358916429317, 31.00000000000000000, -37.35102017232331661 ) ) ;
#24666=CARTESIAN_POINT ( 'NONE',  ( -19.43072497042362556, 31.00000000000000355, 56.92208038676059800 ) ) ;
#24668=CARTESIAN_POINT ( 'NONE',  ( 61.87885091699251916, 39.99999999999999289, -70.55635664373320992 ) ) ;
#24681=CARTESIAN_POINT ( 'NONE',  ( 65.10416666562252885, 39.99999999999999289, 4.254240043327690124 ) ) ;
#24695=CARTESIAN_POINT ( 'NONE',  ( 31.77777543000702565, 31.00000000000000355, 93.95825142778512884 ) ) ;
#24712=CARTESIAN_POINT ( 'NONE',  ( 48.77780477658175329, 31.00000000000000355, -24.05648398140741406 ) ) ;
#24721=CARTESIAN_POINT ( 'NONE',  ( 57.76613438074698337, 39.99999999999999289, -28.48799604501563110 ) ) ;
#24723=CARTESIAN_POINT ( 'NONE',  ( -53.12901929299007975, 40.00000000000000000, 30.56653509229933263 ) ) ;
#24732=CARTESIAN_POINT ( 'NONE',  ( -29.44516979616424024, 40.00000000000000000, -7.879824757621473275 ) ) ;
#24751=CARTESIAN_POINT ( 'NONE',  ( 47.76959191294547225, 31.00000000000000355, 62.44753968350421047 ) ) ;
#24760=CARTESIAN_POINT ( 'NONE',  ( 96.17895579825814423, 39.99999999999999289, -12.55124642863780338 ) ) ;
#24761=CARTESIAN_POINT ( 'NONE',  ( -101.9001375415117963, 40.00000000000000711, 6.549163350515033066 ) ) ;
#24772=CARTESIAN_POINT ( 'NONE',  ( -89.22528799552154055, 31.00000000000000711, 43.99828826784794700 ) ) ;
#24777=CARTESIAN_POINT ( 'NONE',  ( -7.793954689940647995, 40.00000000000000000, 28.94896179907301459 ) ) ;
#24807=CARTESIAN_POINT ( 'NONE',  ( -2.829072032612243159, 31.00000000000000355, -44.39959014221899025 ) ) ;
#24816=CARTESIAN_POINT ( 'NONE',  ( -62.09442273004785307, 40.00000000000000711, -4.163950221635984938 ) ) ;
#24825=CARTESIAN_POINT ( 'NONE',  ( 42.05404839982585941, 31.00000000000000355, -47.95475229022623864 ) ) ;
#24837=VECTOR ( 'NONE', #36999, 1000.000000000000000 ) ;
#24839=CARTESIAN_POINT ( 'NONE',  ( 27.50146173783093317, 31.00000000000000355, -80.63904244945182143 ) ) ;
#24841=CARTESIAN_POINT ( 'NONE',  ( 5.650912336215121456, 40.00000000000000000, -84.59266001511657862 ) ) ;
#24853=DIRECTION ( 'NONE',  ( 0.3211947320043963550, 0.000000000000000000, -0.9470131699890049770 ) ) ;
#24857=CARTESIAN_POINT ( 'NONE',  ( -65.18298466990795248, 40.00000000000000711, 74.32329070269128124 ) ) ;
#24873=CARTESIAN_POINT ( 'NONE',  ( 31.41502175087570947, 40.00000000000000000, -18.07270130326806523 ) ) ;
#24888=CARTESIAN_POINT ( 'NONE',  ( 3.579113344806025054, 31.00000000000000355, 27.11441211503905535 ) ) ;
#24893=CARTESIAN_POINT ( 'NONE',  ( 63.16980243745005907, 31.00000000000000000, -55.41789732285823078 ) ) ;
#24896=CARTESIAN_POINT ( 'NONE',  ( 7.664524495375376389, 31.00000000000000355, 58.91906827746952757 ) ) ;
#24897=CARTESIAN_POINT ( 'NONE',  ( 52.74436945453300041, 40.00000000000000000, 68.73989242669851762 ) ) ;
#24913=CARTESIAN_POINT ( 'NONE',  ( -46.07128526072433772, 40.00000000000000000, -40.40198152342698990 ) ) ;
#24943=CARTESIAN_POINT ( 'NONE',  ( -46.94946386092573221, 31.00000000000000355, 15.94926099647653928 ) ) ;
#24952=CARTESIAN_POINT ( 'NONE',  ( 44.56294422764113250, 40.00000000000000000, 34.17917587534974189 ) ) ;
#24953=CARTESIAN_POINT ( 'NONE',  ( -23.74678488968044832, 40.00000000000000000, -48.36925102894097961 ) ) ;
#24958=CARTESIAN_POINT ( 'NONE',  ( 15.62097837807030842, 31.00000000000000355, -17.81927981957692353 ) ) ;
#24963=CARTESIAN_POINT ( 'NONE',  ( -2.454369252093152376, 40.00000000000000000, 37.60416666486730009 ) ) ;
#24980=CARTESIAN_POINT ( 'NONE',  ( -69.31868535681203980, 31.00000000000000711, 18.45717643660088214 ) ) ;
#24989=CARTESIAN_POINT ( 'NONE',  ( -86.84058463553202500, 40.00000000000000711, 29.36381822872188607 ) ) ;
#24990=CARTESIAN_POINT ( 'NONE',  ( -66.59699903142620769, 40.00000000000000711, 75.74378954611491110 ) ) ;
#25002=CARTESIAN_POINT ( 'NONE',  ( -74.47060461443528823, 31.00000000000000711, 65.33029858165178894 ) ) ;
#25008=CARTESIAN_POINT ( 'NONE',  ( -1.974796425974089331, 40.00000000000000000, 29.60085432090885149 ) ) ;
#25036=CARTESIAN_POINT ( 'NONE',  ( 36.58905133582347702, 31.00000000000000355, -27.97030060560319953 ) ) ;
#25040=CARTESIAN_POINT ( 'NONE',  ( -17.44537629401976275, 17.11489954122026447, 4.261559264950522063 ) ) ;
#25044=CARTESIAN_POINT ( 'NONE',  ( 41.67488199336423804, 40.00000000000000000, 54.49293397273886086 ) ) ;
#25054=CARTESIAN_POINT ( 'NONE',  ( -17.60292107714122878, 31.00000000000000355, 65.74579412301164894 ) ) ;
#25067=CARTESIAN_POINT ( 'NONE',  ( -79.74759331938361129, 31.00000000000000711, -21.47736420602193519 ) ) ;
#25068=CARTESIAN_POINT ( 'NONE',  ( -37.02054590706428172, 40.00000000000000000, -75.34311506435015815 ) ) ;
#25093=CARTESIAN_POINT ( 'NONE',  ( 17.75583184595346964, 40.00000000000000000, -30.63479189996225216 ) ) ;
#25102=CARTESIAN_POINT ( 'NONE',  ( 5.583751958424166162, 31.00000000000000355, -42.43436172917101601 ) ) ;
#25109=CARTESIAN_POINT ( 'NONE',  ( 74.72486387243833406, 31.00000000000000000, 9.837939412698395003 ) ) ;
#25113=CARTESIAN_POINT ( 'NONE',  ( 33.95200755730775199, 31.00000000000000355, -44.10258293179329314 ) ) ;
#25114=CARTESIAN_POINT ( 'NONE',  ( 84.66040299356156140, 39.99999999999999289, 11.14692016787551765 ) ) ;
#25126=CARTESIAN_POINT ( 'NONE',  ( 40.54457361686378647, 40.00000000000000000, 52.83773991529862712 ) ) ;
#25131=CARTESIAN_POINT ( 'NONE',  ( -101.9145453900124068, 17.11489954122026447, -1.407535261550463268 ) ) ;
#25150=CARTESIAN_POINT ( 'NONE',  ( -29.60425243605831724, 31.00000000000000355, 38.59963703562669934 ) ) ;
#25157=CARTESIAN_POINT ( 'NONE',  ( 28.40420691229738281, 40.00000000000000000, 49.17333623205379922 ) ) ;
#25167=CARTESIAN_POINT ( 'NONE',  ( -2.924622967158192921, 31.00000000000000355, -22.14664255385889291 ) ) ;
#25169=CARTESIAN_POINT ( 'NONE',  ( -14.08558183832706234, 40.00000000000000000, -28.55406316770863739 ) ) ;
#25183=CARTESIAN_POINT ( 'NONE',  ( -81.27520743792995006, 31.00000000000000711, 10.59408403752164851 ) ) ;
#25190=CARTESIAN_POINT ( 'NONE',  ( -26.02152878260477564, 40.00000000000000000, 96.68563202207252516 ) ) ;
#25193=CARTESIAN_POINT ( 'NONE',  ( -18.31940394017777507, 31.00000000000000355, -14.05611420671224288 ) ) ;
#25207=CARTESIAN_POINT ( 'NONE',  ( -65.18298466990795248, 31.00000000000000711, 74.32329070269128124 ) ) ;
#25210=CARTESIAN_POINT ( 'NONE',  ( -6.237032369604346371, 40.00000000000000000, -23.31551866006812901 ) ) ;
#25237=CARTESIAN_POINT ( 'NONE',  ( -6.590854309045712789, 31.00000000000000355, 49.37518673228670707 ) ) ;
#25244=CARTESIAN_POINT ( 'NONE',  ( -70.06919973880852126, 40.00000000000000711, -18.87919424805731339 ) ) ;
#25253=CARTESIAN_POINT ( 'NONE',  ( -60.02123122004734768, 31.00000000000000711, 34.66859033927303813 ) ) ;
#25259=VERTEX_POINT ( 'NONE', #5872 ) ;
#25263=CARTESIAN_POINT ( 'NONE',  ( 74.83201185292551827, 31.00000000000000000, -43.08100868842220166 ) ) ;
#25264=CARTESIAN_POINT ( 'NONE',  ( 28.55926749299792178, 40.00000000000000000, 84.46800049165049984 ) ) ;
#25286=FACE_OUTER_BOUND ( 'NONE', #1908, .T. ) ;
#25296=CARTESIAN_POINT ( 'NONE',  ( -26.44890248586417414, 40.00000000000000000, -34.59877114778964113 ) ) ;
#25305=CARTESIAN_POINT ( 'NONE',  ( 22.24487986055951083, 31.00000000000000355, 28.98451114863597766 ) ) ;
#25307=( NAMED_UNIT ( * ) SI_UNIT ( $, .STERADIAN. ) SOLID_ANGLE_UNIT ( ) );
#25312=CARTESIAN_POINT ( 'NONE',  ( -68.69954721042445556, 31.00000000000000711, 39.68009708086182741 ) ) ;
#25314=CARTESIAN_POINT ( 'NONE',  ( 54.79583221319987985, 31.00000000000000355, -14.58025558542526490 ) ) ;
#25316=CARTESIAN_POINT ( 'NONE',  ( -68.67288961433401084, 40.00000000000000711, -60.22678404055071155 ) ) ;
#25327=CARTESIAN_POINT ( 'NONE',  ( -60.02123122004734768, 40.00000000000000711, 34.66859033927303813 ) ) ;
#25356=LINE ( 'NONE', #21668, #4404 ) ;
#25357=CARTESIAN_POINT ( 'NONE',  ( 15.14372185054182651, 31.00000000000000355, 44.57714859939663654 ) ) ;
#25363=CARTESIAN_POINT ( 'NONE',  ( -58.48566925782336057, 40.00000000000000711, -15.65830181329500803 ) ) ;
#25368=CARTESIAN_POINT ( 'NONE',  ( -19.76500330823589735, 31.00000000000000355, -5.286999072153966139 ) ) ;
#25371=CARTESIAN_POINT ( 'NONE',  ( 25.50046184691807483, 40.00000000000000000, -22.37655979312362931 ) ) ;
#25385=CARTESIAN_POINT ( 'NONE',  ( -81.90010630563853056, 31.00000000000000711, 5.248159452637419342 ) ) ;
#25394=CARTESIAN_POINT ( 'NONE',  ( -66.59699903142620769, 40.00000000000000711, 75.74378954611491110 ) ) ;
#25395=CARTESIAN_POINT ( 'NONE',  ( 8.075107282080610460, 31.00000000000000355, -23.73893940452553508 ) ) ;
#25399=DIRECTION ( 'NONE',  ( 0.000000000000000000, -1.000000000000000000, 5.297542245118643184E-16 ) ) ;
#25407=CARTESIAN_POINT ( 'NONE',  ( 25.17870271038170316, 31.00000000000000355, 93.97695291299892517 ) ) ;
#25410=CARTESIAN_POINT ( 'NONE',  ( -25.30796725786148826, 40.00000000000000000, 14.62256337265529815 ) ) ;
#25412=CARTESIAN_POINT ( 'NONE',  ( 17.12248163736668261, 40.00000000000000000, 34.87662400048956357 ) ) ;
#25433=EDGE_CURVE ( 'NONE', #10114, #6869, #20306, .T. ) ;
#25434=LINE ( 'NONE', #41966, #32568 ) ;
#25437=CARTESIAN_POINT ( 'NONE',  ( -105.0363123600777442, 17.11489954122026447, -2.692529638013756887 ) ) ;
#25439=CARTESIAN_POINT ( 'NONE',  ( 38.48770111205617894, 31.00000000000000355, 44.02435964457617956 ) ) ;
#25444=LINE ( 'NONE', #25040, #2837 ) ;
#25446=CARTESIAN_POINT ( 'NONE',  ( -67.85934734800838442, 40.00000000000000711, 22.92939687791763248 ) ) ;
#25459=CARTESIAN_POINT ( 'NONE',  ( -8.856203846296160975, 31.00000000000000355, 67.27320953167645712 ) ) ;
#25469=CARTESIAN_POINT ( 'NONE',  ( 52.26791824981292223, 31.00000000000000355, -67.94187691988643962 ) ) ;
#25470=CARTESIAN_POINT ( 'NONE',  ( 27.50146173784981229, 40.00000000000000000, -80.63904244945182143 ) ) ;
#25490=CARTESIAN_POINT ( 'NONE',  ( 24.91045342551303321, 31.00000000000000355, 12.31387362277163433 ) ) ;
#25498=CARTESIAN_POINT ( 'NONE',  ( -2.829072032612394594, 40.00000000000000000, -44.39959014221900446 ) ) ;
#25516=CARTESIAN_POINT ( 'NONE',  ( 34.28525303991722240, 31.00000000000000355, 9.176237600273646322 ) ) ;
#25523=CARTESIAN_POINT ( 'NONE',  ( -87.52616871875942195, 31.00000000000000711, -23.43677886868077209 ) ) ;
#25526=CARTESIAN_POINT ( 'NONE',  ( -46.12092335262209986, 31.00000000000000355, 22.64177125690870795 ) ) ;
#25528=CARTESIAN_POINT ( 'NONE',  ( -86.71682804797315214, 40.00000000000000711, 23.23408344657299196 ) ) ;
#25532=DIRECTION ( 'NONE',  ( 0.000000000000000000, -1.000000000000000000, 5.297542245118643184E-16 ) ) ;
#25542=CARTESIAN_POINT ( 'NONE',  ( -77.03666156126601550, 40.00000000000000711, 20.64125776147949409 ) ) ;
#25572=CARTESIAN_POINT ( 'NONE',  ( -49.46937513889707105, 31.00000000000000355, 6.524320044134898744 ) ) ;
#25573=ORIENTED_EDGE ( 'NONE', *, *, #36398, .T. ) ;
#25582=CARTESIAN_POINT ( 'NONE',  ( 38.75409931461306456, 40.00000000000000000, -50.52625141960567134 ) ) ;
#25591=CARTESIAN_POINT ( 'NONE',  ( 30.80114556864472775, 40.00000000000000000, -15.19345985420777190 ) ) ;
#25605=CARTESIAN_POINT ( 'NONE',  ( -20.82795069773117547, 31.00000000000000355, 77.32795358076221248 ) ) ;
#25612=CARTESIAN_POINT ( 'NONE',  ( -50.38378093996033869, 40.00000000000000711, 87.00968337440519917 ) ) ;
#25613=CARTESIAN_POINT ( 'NONE',  ( -20.42974159057666483, 31.00000000000000355, -10.07157319949386753 ) ) ;
#25627=CARTESIAN_POINT ( 'NONE',  ( 2.127120017302678523, 40.00000000000000000, -32.60416666460785962 ) ) ;
#25629=CARTESIAN_POINT ( 'NONE',  ( -2.197745971917953511, 40.00000000000000000, -34.39891587002171747 ) ) ;
#25645=ORIENTED_EDGE ( 'NONE', *, *, #2272, .F. ) ;
#25653=CARTESIAN_POINT ( 'NONE',  ( -85.90019077458921970, 40.00000000000000711, -29.16093118951848240 ) ) ;
#25654=ORIENTED_EDGE ( 'NONE', *, *, #10934, .F. ) ;
#25659=CARTESIAN_POINT ( 'NONE',  ( -52.09564885853935579, 31.00000000000000355, -3.498939618562641574 ) ) ;
#25667=CARTESIAN_POINT ( 'NONE',  ( -18.22940504111446458, 40.00000000000000000, 67.64968002090884625 ) ) ;
#25679=CARTESIAN_POINT ( 'NONE',  ( 48.10206620145878276, 31.00000000000000355, -42.20136231105875879 ) ) ;
#25687=CARTESIAN_POINT ( 'NONE',  ( -101.9145453900123641, 40.00000000000000000, -1.407535261550449501 ) ) ;
#25689=CARTESIAN_POINT ( 'NONE',  ( 97.09201668843397215, 31.00000000000000000, 6.474068422258194566 ) ) ;
#25690=CARTESIAN_POINT ( 'NONE',  ( 12.51314706078825090, 40.00000000000000000, -94.07914177280382262 ) ) ;
#25711=CARTESIAN_POINT ( 'NONE',  ( 14.33709021557830887, 31.00000000000000355, 24.89380824183666263 ) ) ;
#25720=CARTESIAN_POINT ( 'NONE',  ( -12.95950413119146205, 40.00000000000000000, 37.95406330258916938 ) ) ;
#25731=CARTESIAN_POINT ( 'NONE',  ( 16.30133787010129254, 31.00000000000000355, 33.04822796959624753 ) ) ;
#25737=CARTESIAN_POINT ( 'NONE',  ( -5.726861599740728614, 31.00000000000000355, 87.60416666588449175 ) ) ;
#25740=CARTESIAN_POINT ( 'NONE',  ( 58.81396797841471624, 31.00000000000000355, 34.08301911901634895 ) ) ;
#25741=CARTESIAN_POINT ( 'NONE',  ( 34.31975892712151222, 40.00000000000000000, 59.64049725130580271 ) ) ;
#25742=CARTESIAN_POINT ( 'NONE',  ( 94.89583333399441756, 39.99999999999999289, -6.217735451874103703 ) ) ;
#25755=CARTESIAN_POINT ( 'NONE',  ( 10.12401712103624263, 40.00000000000000000, 76.79210772277129138 ) ) ;
#25781=CARTESIAN_POINT ( 'NONE',  ( -48.53848235557606472, 31.00000000000000355, -37.22912483484027035 ) ) ;
#25785=CARTESIAN_POINT ( 'NONE',  ( -43.59452257625678584, 40.00000000000000000, -56.81327804312699925 ) ) ;
#25788=DIRECTION ( 'NONE',  ( 0.000000000000000000, 0.000000000000000000, 1.000000000000000000 ) ) ;
#25793=CARTESIAN_POINT ( 'NONE',  ( 21.71086051706764763, 40.00000000000000000, -37.60982366119799991 ) ) ;
#25796=PLANE ( 'NONE',  #33323 ) ;
#25807=FACE_OUTER_BOUND ( 'NONE', #14791, .T. ) ;
#25809=CARTESIAN_POINT ( 'NONE',  ( 84.58694138809386232, 31.00000000000000000, 22.77597867319729374 ) ) ;
#25824=CARTESIAN_POINT ( 'NONE',  ( 1.799870782497353439, 31.00000000000000355, 27.39583333577991908 ) ) ;
#25832=CARTESIAN_POINT ( 'NONE',  ( 25.04716826810500763, 40.00000000000000000, 3.293035637142270655 ) ) ;
#25833=CARTESIAN_POINT ( 'NONE',  ( -31.99444157863030114, 40.00000000000000000, -4.262017635501984536 ) ) ;
#25835=ORIENTED_EDGE ( 'NONE', *, *, #26632, .T. ) ;
#25853=CARTESIAN_POINT ( 'NONE',  ( 46.76839422406115432, 39.99999999999999289, -81.00140361174831583 ) ) ;
#25862=CARTESIAN_POINT ( 'NONE',  ( 44.54779904930365575, 31.00000000000000355, -34.05916983163054113 ) ) ;
#25872=CARTESIAN_POINT ( 'NONE',  ( 22.12550800842195287, 40.00000000000000000, 65.48657384633656875 ) ) ;
#25883=CARTESIAN_POINT ( 'NONE',  ( 5.399612364985509672, 31.00000000000000355, -82.60416666586320389 ) ) ;
#25885=CARTESIAN_POINT ( 'NONE',  ( -19.99999999999999645, 17.11489954122026447, 1.283214542831033755 ) ) ;
#25893=CARTESIAN_POINT ( 'NONE',  ( 6.386360208629405122, 31.00000000000000355, 99.40013590833048340 ) ) ;
#25894=CARTESIAN_POINT ( 'NONE',  ( -41.44813913998980581, 40.00000000000000000, -84.33308812960441969 ) ) ;
#25909=CARTESIAN_POINT ( 'NONE',  ( -22.10416666678001008, 31.00000000000000355, -1.441157586896874898 ) ) ;
#25917=CARTESIAN_POINT ( 'NONE',  ( 45.06603723658675875, 40.00000000000000000, 15.38899812202754624 ) ) ;
#25930=CARTESIAN_POINT ( 'NONE',  ( 32.71557229150619861, 31.00000000000000355, -11.11602612089219910 ) ) ;
#25934=CARTESIAN_POINT ( 'NONE',  ( 11.43299787627070607, 31.00000000000000355, 86.72764684403134083 ) ) ;
#25937=CARTESIAN_POINT ( 'NONE',  ( 51.26988013555838819, 31.00000000000000355, 45.10883117380814866 ) ) ;
#25938=CARTESIAN_POINT ( 'NONE',  ( -56.48168293059611500, 40.00000000000000711, 43.19841958066528065 ) ) ;
#25939=CARTESIAN_POINT ( 'NONE',  ( 94.59594211465898184, 39.99999999999999289, 12.45590092308117569 ) ) ;
#25945=LINE ( 'NONE', #26373, #28950 ) ;
#25952=CARTESIAN_POINT ( 'NONE',  ( 58.80104710710317306, 39.99999999999999289, -45.11949705600698479 ) ) ;
#25968=VERTEX_POINT ( 'NONE', #3168 ) ;
#25980=CARTESIAN_POINT ( 'NONE',  ( 50.09382087749727930, 31.00000000000000355, 24.69014870349942825 ) ) ;
#25984=CARTESIAN_POINT ( 'NONE',  ( -22.00208165626505519, 31.00000000000000355, -25.16137218361809502 ) ) ;
#25985=CARTESIAN_POINT ( 'NONE',  ( 33.41571365387085280, 40.00000000000000000, 57.85165222247763239 ) ) ;
#25994=CARTESIAN_POINT ( 'NONE',  ( -13.53264355869793967, 40.00000000000000000, -39.83251807627727459 ) ) ;
#26005=CARTESIAN_POINT ( 'NONE',  ( -79.74759331938361129, 31.00000000000000711, -21.47736420602193519 ) ) ;
#26022=CARTESIAN_POINT ( 'NONE',  ( 14.71924655979513297, 31.00000000000000355, -29.87007926703815741 ) ) ;
#26028=CARTESIAN_POINT ( 'NONE',  ( -25.29482881991252086, 40.00000000000000000, -32.96004927633274662 ) ) ;
#26029=STYLED_ITEM ( 'NONE', ( #31121 ), #31788 ) ;
#26030=CARTESIAN_POINT ( 'NONE',  ( 35.42814233786123879, 40.00000000000000000, -9.427541829740359702 ) ) ;
#26043=ORIENTED_EDGE ( 'NONE', *, *, #30853, .F. ) ;
#26046=CARTESIAN_POINT ( 'NONE',  ( -105.9879088449591933, 40.00000000000000000, -0.3807199291576673361 ) ) ;
#26060=CARTESIAN_POINT ( 'NONE',  ( 14.32751628686350287, 31.00000000000000355, -53.13354968560084757 ) ) ;
#26068=CARTESIAN_POINT ( 'NONE',  ( -68.78002826189113250, 40.00000000000000711, -23.46745878763887916 ) ) ;
#26081=CARTESIAN_POINT ( 'NONE',  ( 74.30822294231431613, 31.00000000000000000, -9.796771932235298408 ) ) ;
#26093=CARTESIAN_POINT ( 'NONE',  ( 96.17895579821514218, 31.00000000000000000, -12.55124642863780515 ) ) ;
#26094=CARTESIAN_POINT ( 'NONE',  ( -61.59955500558135100, 40.00000000000000711, -70.40623950603891501 ) ) ;
#26115=CARTESIAN_POINT ( 'NONE',  ( -19.81637295874435978, 31.00000000000000355, -11.44243563873997793 ) ) ;
#26119=ORIENTED_EDGE ( 'NONE', *, *, #9450, .T. ) ;
#26124=CARTESIAN_POINT ( 'NONE',  ( 17.12248163736668261, 40.00000000000000000, 34.87662400048956357 ) ) ;
#26125=LINE ( 'NONE', #39390, #14650 ) ;
#26134=CARTESIAN_POINT ( 'NONE',  ( 44.50160557815096496, 31.00000000000000355, -5.869829666507492050 ) ) ;
#26138=CARTESIAN_POINT ( 'NONE',  ( -28.35539204363714205, 31.00000000000000355, 83.52787551312086123 ) ) ;
#26142=CARTESIAN_POINT ( 'NONE',  ( -61.89998375878432313, 31.00000000000000711, 3.952486745199417673 ) ) ;
#26143=CARTESIAN_POINT ( 'NONE',  ( -54.47698434027259395, 40.00000000000000000, -31.57393205620729404 ) ) ;
#26146=CARTESIAN_POINT ( 'NONE',  ( -94.39576909109665337, 40.00000000000000711, 32.06004391471374504 ) ) ;
#26158=CARTESIAN_POINT ( 'NONE',  ( 60.46509673945340779, 39.99999999999999289, 46.37897171328766888 ) ) ;
#26187=CARTESIAN_POINT ( 'NONE',  ( -15.01009539198478748, 31.00000000000000355, 56.06562763604418365 ) ) ;
#26191=CARTESIAN_POINT ( 'NONE',  ( -14.91913624998189469, 31.00000000000000355, -30.37684071746364012 ) ) ;
#26193=CARTESIAN_POINT ( 'NONE',  ( 70.67261647610648367, 39.99999999999999289, -24.00465245562410743 ) ) ;
#26206=CARTESIAN_POINT ( 'NONE',  ( 44.50160557815096496, 40.00000000000000000, -5.869829666507492050 ) ) ;
#26218=CARTESIAN_POINT ( 'NONE',  ( 97.09201668843397215, 31.00000000000000000, 6.474068422258194566 ) ) ;
#26239=CARTESIAN_POINT ( 'NONE',  ( -12.50349052776452297, 31.00000000000000355, 25.37591446456323041 ) ) ;
#26246=CARTESIAN_POINT ( 'NONE',  ( 22.24487986055951083, 40.00000000000000000, 28.98451114863597766 ) ) ;
#26248=CARTESIAN_POINT ( 'NONE',  ( -25.29816761084670063, 40.00000000000000000, 43.63644233508315295 ) ) ;
#26266=EDGE_CURVE ( 'NONE', #20422, #19261, #9481, .T. ) ;
#26278=CARTESIAN_POINT ( 'NONE',  ( -7.911223860809958097, 31.00000000000000355, 59.30865348673673765 ) ) ;
#26285=CARTESIAN_POINT ( 'NONE',  ( -77.35014290652780744, 40.00000000000000711, 26.14598721591455899 ) ) ;
#26301=CARTESIAN_POINT ( 'NONE',  ( -20.19574676229028043, 31.00000000000000355, 75.42596061005518493 ) ) ;
#26313=CARTESIAN_POINT ( 'NONE',  ( 93.52153384689862037, 31.00000000000000000, -24.92737483788710406 ) ) ;
#26314=CARTESIAN_POINT ( 'NONE',  ( 42.30527206516848793, 40.00000000000000000, -85.53883208674149330 ) ) ;
#26342=CARTESIAN_POINT ( 'NONE',  ( 36.84045577241590763, 40.00000000000000000, -41.86038302679909151 ) ) ;
#26356=CARTESIAN_POINT ( 'NONE',  ( 41.10549127292548377, 31.00000000000000355, 20.25863663968860706 ) ) ;
#26362=CARTESIAN_POINT ( 'NONE',  ( -89.89583333403318477, 31.00000000000000711, 5.890486217120591839 ) ) ;
#26367=CARTESIAN_POINT ( 'NONE',  ( -31.21560191380782001, 31.00000000000000355, 63.07420938637471863 ) ) ;
#26368=CARTESIAN_POINT ( 'NONE',  ( 4.437437895627098783, 40.00000000000000000, 69.40004907513484511 ) ) ;
#26373=CARTESIAN_POINT ( 'NONE',  ( -16.41266422346948772, 40.00000000000000000, -1.216702565357022037 ) ) ;
#26380=CARTESIAN_POINT ( 'NONE',  ( 36.74538074116732389, 40.00000000000000000, -63.64477163140654170 ) ) ;
#26383=DIRECTION ( 'NONE',  ( 0.000000000000000000, 1.000000000000000000, 0.000000000000000000 ) ) ;
#26404=CARTESIAN_POINT ( 'NONE',  ( -19.99999999999999645, 31.00000000000000355, 2.168407390121265812E-15 ) ) ;
#26410=CARTESIAN_POINT ( 'NONE',  ( 64.37268382102905662, 31.00000000000000000, -8.487791176987355968 ) ) ;
#26414=CARTESIAN_POINT ( 'NONE',  ( 28.69597684714336339, 31.00000000000000355, 25.25520295781697655 ) ) ;
#26415=CARTESIAN_POINT ( 'NONE',  ( -54.82550897924149069, 40.00000000000000711, 42.06954809655981364 ) ) ;
#26421=CARTESIAN_POINT ( 'NONE',  ( 13.85568741775851542, 40.00000000000000000, -40.82620080729295609 ) ) ;
#26432=CARTESIAN_POINT ( 'NONE',  ( 91.58570893733639195, 31.00000000000000000, -30.97307622143650363 ) ) ;
#26450=CARTESIAN_POINT ( 'NONE',  ( 29.64712525329720449, 31.00000000000000355, -17.12831674356021239 ) ) ;
#26457=CARTESIAN_POINT ( 'NONE',  ( -16.93500259178182432, 40.00000000000000000, 34.36424406943201149 ) ) ;
#26458=CARTESIAN_POINT ( 'NONE',  ( -40.56882557769177566, 40.00000000000000000, 31.01417895415859505 ) ) ;
#26468=ORIENTED_EDGE ( 'NONE', *, *, #6812, .F. ) ;
#26485=CARTESIAN_POINT ( 'NONE',  ( 58.81396797841471624, 31.00000000000000355, 34.08301911901634895 ) ) ;
#26492=CARTESIAN_POINT ( 'NONE',  ( -10.92011822083620309, 40.00000000000000000, -83.75917815547794021 ) ) ;
#26505=CARTESIAN_POINT ( 'NONE',  ( 58.80104710710317306, 31.00000000000000000, -45.11949705600698479 ) ) ;
#26514=CARTESIAN_POINT ( 'NONE',  ( -72.38966680861454961, 31.00000000000000711, 55.38960906678870089 ) ) ;
#26522=EDGE_CURVE ( 'NONE', #27469, #36133, #25356, .T. ) ;
#26536=CARTESIAN_POINT ( 'NONE',  ( -28.46928290085317315, 31.00000000000000355, -16.49637127829624106 ) ) ;
#26537=DIRECTION ( 'NONE',  ( 0.000000000000000000, 1.000000000000000000, 0.000000000000000000 ) ) ;
#26539=CARTESIAN_POINT ( 'NONE',  ( -15.99999999999997691, 17.11489954122026447, 5.571627607371296764E-15 ) ) ;
#26544=CARTESIAN_POINT ( 'NONE',  ( -13.93478910046542829, 40.00000000000000000, -52.37520058408175316 ) ) ;
#26559=CARTESIAN_POINT ( 'NONE',  ( 19.15075862373047144, 31.00000000000000355, -38.85840887180553693 ) ) ;
#26565=CARTESIAN_POINT ( 'NONE',  ( 14.35450763783260797, 40.00000000000000000, -18.72194639494853874 ) ) ;
#26570=CARTESIAN_POINT ( 'NONE',  ( -55.11358496760189496, 31.00000000000000711, 27.06326608205353779 ) ) ;
#26571=CARTESIAN_POINT ( 'NONE',  ( 51.26988013557343749, 40.00000000000000000, 45.10883117380814866 ) ) ;
#26572=CARTESIAN_POINT ( 'NONE',  ( 12.74197863150380883, 40.00000000000000000, 96.66318596537892915 ) ) ;
#26587=CARTESIAN_POINT ( 'NONE',  ( -89.89583333403318477, 40.00000000000000711, 5.890486217120591839 ) ) ;
#26607=ORIENTED_EDGE ( 'NONE', *, *, #8735, .T. ) ;
#26617=CARTESIAN_POINT ( 'NONE',  ( -66.92166868300088822, 31.00000000000000711, -22.71661802240650019 ) ) ;
#26619=CARTESIAN_POINT ( 'NONE',  ( 19.31996883370903362, 31.00000000000000355, 33.58758284028576924 ) ) ;
#26621=CARTESIAN_POINT ( 'NONE',  ( 4.417864660711233959, 40.00000000000000000, 67.39583333436242185 ) ) ;
#26632=EDGE_CURVE ( 'NONE', #33075, #7939, #18389, .T. ) ;
#26634=CARTESIAN_POINT ( 'NONE',  ( 33.03432996520027132, 40.00000000000000000, -28.98482729919588863 ) ) ;
#26648=CARTESIAN_POINT ( 'NONE',  ( -45.36921519482122278, 31.00000000000000711, 78.33339762288051134 ) ) ;
#26664=CARTESIAN_POINT ( 'NONE',  ( 11.86982580658625075, 31.00000000000000355, 24.05989836594520526 ) ) ;
#26668=ORIENTED_EDGE ( 'NONE', *, *, #38506, .F. ) ;
#26670=CARTESIAN_POINT ( 'NONE',  ( -39.89583333501392559, 40.00000000000000000, 2.617993869485681468 ) ) ;
#26671=CARTESIAN_POINT ( 'NONE',  ( 34.59698569361206211, 40.00000000000000000, -30.23997570423562209 ) ) ;
#26700=CARTESIAN_POINT ( 'NONE',  ( -38.62815422673675414, 31.00000000000000355, -50.51519254952904703 ) ) ;
#26706=CARTESIAN_POINT ( 'NONE',  ( 69.92891852059224789, 39.99999999999999289, 53.79372986807582180 ) ) ;
#26709=DIRECTION ( 'NONE',  ( 0.06345332152672161774, -5.286866677681789116E-16, -0.9979848074931934043 ) ) ;
#26716=CARTESIAN_POINT ( 'NONE',  ( -79.27599250299880396, 31.00000000000000711, 10.45126230984107707 ) ) ;
#26749=CARTESIAN_POINT ( 'NONE',  ( 31.41502175087182991, 31.00000000000000355, -18.07270130326418922 ) ) ;
#26756=CARTESIAN_POINT ( 'NONE',  ( 53.62204311759386854, 40.00000000000000000, -18.10832464707264577 ) ) ;
#26766=CARTESIAN_POINT ( 'NONE',  ( -3.108867721649295035, 31.00000000000000355, 47.60416666525765095 ) ) ;
#26773=CARTESIAN_POINT ( 'NONE',  ( -2.924622967158192921, 40.00000000000000000, -22.14664255385889291 ) ) ;
#26777=CARTESIAN_POINT ( 'NONE',  ( -55.03444096782886419, 31.00000000000000355, -48.41538206856125015 ) ) ;
#26778=CARTESIAN_POINT ( 'NONE',  ( -70.49178429274644486, 40.00000000000000711, 40.57739572807859929 ) ) ;
#26796=CARTESIAN_POINT ( 'NONE',  ( 64.90595555531619709, 39.99999999999999289, 56.92265028770086843 ) ) ;
#26808=CARTESIAN_POINT ( 'NONE',  ( 1.622176940739286310, 40.00000000000000000, -24.60292901074089045 ) ) ;
#26829=AXIS2_PLACEMENT_3D ( 'NONE', #22638, #31796, #19152 ) ;
#26830=CARTESIAN_POINT ( 'NONE',  ( 29.59587406094124873, 31.00000000000000355, 60.01321678176139329 ) ) ;
#26832=CARTESIAN_POINT ( 'NONE',  ( -41.89947471387618805, 31.00000000000000355, 2.670153906482984674 ) ) ;
#26833=CARTESIAN_POINT ( 'NONE',  ( -72.56464488860213180, 40.00000000000000711, -35.76892886290303863 ) ) ;
#26845=CARTESIAN_POINT ( 'NONE',  ( -48.80550277073417931, 40.00000000000000000, -13.06547612810710035 ) ) ;
#26860=CARTESIAN_POINT ( 'NONE',  ( -92.09225407318749035, 31.00000000000000711, -6.144973693751363264 ) ) ;
#26881=CARTESIAN_POINT ( 'NONE',  ( -39.12533628356670334, 31.00000000000000355, -10.47265044290268499 ) ) ;
#26891=CARTESIAN_POINT ( 'NONE',  ( 19.15075862373047144, 40.00000000000000000, -38.85840887180553693 ) ) ;
#26892=CARTESIAN_POINT ( 'NONE',  ( 14.57966847436756019, 40.00000000000000000, -42.69519604897453036 ) ) ;
#26898=CARTESIAN_POINT ( 'NONE',  ( -20.10416666680962550, 40.00000000000000000, -1.308996940106889273 ) ) ;
#26916=CARTESIAN_POINT ( 'NONE',  ( -55.11358496760189496, 31.00000000000000711, 27.06326608205353779 ) ) ;
#26923=VERTEX_POINT ( 'NONE', #30545 ) ;
#26924=CARTESIAN_POINT ( 'NONE',  ( -41.82916961767931951, 40.00000000000000000, -72.66191475361131324 ) ) ;
#26936=CARTESIAN_POINT ( 'NONE',  ( -29.64342647699677613, 31.00000000000000355, -87.27882330658468391 ) ) ;
#26949=CARTESIAN_POINT ( 'NONE',  ( -50.38378093998269946, 31.00000000000000711, 87.00968337440518496 ) ) ;
#26969=CARTESIAN_POINT ( 'NONE',  ( 3.798394181603659270, 31.00000000000000355, 29.10671710469610574 ) ) ;
#26975=UNCERTAINTY_MEASURE_WITH_UNIT (LENGTH_MEASURE( 1.000000000000000082E-05 ), #12825, 'distance_accuracy_value', 'NONE');
#26979=CARTESIAN_POINT ( 'NONE',  ( 51.84393115708665079, 40.00000000000000000, 25.66707601012906537 ) ) ;
#26987=ORIENTED_EDGE ( 'NONE', *, *, #15485, .T. ) ;
#26994=CARTESIAN_POINT ( 'NONE',  ( -44.28363997456384737, 31.00000000000000355, 21.84072794957603492 ) ) ;
#27002=CARTESIAN_POINT ( 'NONE',  ( 1.472621547668719444, 40.00000000000000000, -22.60416666365413718 ) ) ;
#27008=CARTESIAN_POINT ( 'NONE',  ( -70.06919973877657526, 31.00000000000000711, -18.87919424805730984 ) ) ;
#27009=CARTESIAN_POINT ( 'NONE',  ( 66.15140951845482675, 39.99999999999999289, -38.07406969931857077 ) ) ;
#27026=CARTESIAN_POINT ( 'NONE',  ( 84.66040299356156140, 39.99999999999999289, 11.14692016787551765 ) ) ;
#27039=CARTESIAN_POINT ( 'NONE',  ( 27.10182830755125138, 40.00000000000000000, 1.799748011963437255 ) ) ;
#27060=CARTESIAN_POINT ( 'NONE',  ( 21.58803501788969115, 31.00000000000000355, 63.55567069162312777 ) ) ;
#27062=CARTESIAN_POINT ( 'NONE',  ( 24.31498657912377226, 31.00000000000000355, 42.27453502171529465 ) ) ;
#27063=CARTESIAN_POINT ( 'NONE',  ( -20.19574676229028043, 40.00000000000000000, 75.42596061005518493 ) ) ;
#27072=CARTESIAN_POINT ( 'NONE',  ( -56.43872490705654599, 40.00000000000000711, 19.17141758012168751 ) ) ;
#27088=CARTESIAN_POINT ( 'NONE',  ( 12.51314706078824912, 31.00000000000000355, -94.07914177284597201 ) ) ;
#27093=DIRECTION ( 'NONE',  ( 0.000000000000000000, 1.000000000000000000, -1.060184893785364939E-15 ) ) ;
#27102=FACE_OUTER_BOUND ( 'NONE', #1950, .T. ) ;
#27108=CARTESIAN_POINT ( 'NONE',  ( 11.12085686420672381, 31.00000000000000355, -41.54537790535560760 ) ) ;
#27112=CARTESIAN_POINT ( 'NONE',  ( -105.3367680159044966, 31.00000000000000355, 2.032994142711224583 ) ) ;
#27113=ORIENTED_EDGE ( 'NONE', *, *, #39490, .T. ) ;
#27116=CARTESIAN_POINT ( 'NONE',  ( 34.77048308403384169, 40.00000000000000000, 30.48958026498159768 ) ) ;
#27117=CARTESIAN_POINT ( 'NONE',  ( 2.996940313443920978, 40.00000000000000000, -44.59688583547568896 ) ) ;
#27123=CARTESIAN_POINT ( 'NONE',  ( 23.22631124480444598, 40.00000000000000000, -7.893869537065737241 ) ) ;
#27144=CARTESIAN_POINT ( 'NONE',  ( -4.113979049837550583, 31.00000000000000355, -64.40000927351897531 ) ) ;
#27150=CARTESIAN_POINT ( 'NONE',  ( -53.37462671635322664, 40.00000000000000711, 60.68184199298008252 ) ) ;
#27161=CARTESIAN_POINT ( 'NONE',  ( -15.99999999999997691, 31.00000000000000355, 2.500000000000006217 ) ) ;
#27162=CARTESIAN_POINT ( 'NONE',  ( -81.55297449308174862, 31.00000000000000711, -40.20044092665353475 ) ) ;
#27190=CARTESIAN_POINT ( 'NONE',  ( -4.434938641671373638, 31.00000000000000355, -34.07637162043106116 ) ) ;
#27197=CARTESIAN_POINT ( 'NONE',  ( -49.95450512539639476, 40.00000000000000000, 13.28959769214884545 ) ) ;
#27207=CARTESIAN_POINT ( 'NONE',  ( 42.30435120181500963, 31.00000000000000355, 37.09784777058769123 ) ) ;
#27213=CARTESIAN_POINT ( 'NONE',  ( 15.62097837807030842, 40.00000000000000000, -17.81927981957692353 ) ) ;
#27219=CARTESIAN_POINT ( 'NONE',  ( 76.69346925293527306, 31.00000000000000000, 10.21457306974767398 ) ) ;
#27220=CARTESIAN_POINT ( 'NONE',  ( -5.321195512787074478, 40.00000000000000000, 79.59297073838583003 ) ) ;
#27232=CARTESIAN_POINT ( 'NONE',  ( 68.41617299536980568, 39.99999999999999289, 52.47886963225217016 ) ) ;
#27253=LINE ( 'NONE', #23351, #745 ) ;
#27258=CARTESIAN_POINT ( 'NONE',  ( 2.127120017302678523, 31.00000000000000355, -32.60416666460785962 ) ) ;
#27265=CARTESIAN_POINT ( 'NONE',  ( 33.41571365387085280, 31.00000000000000355, 57.85165222247763239 ) ) ;
#27268=CARTESIAN_POINT ( 'NONE',  ( 42.86166521170756027, 31.00000000000000355, 21.22462828018744219 ) ) ;
#27269=CARTESIAN_POINT ( 'NONE',  ( -5.072363130230006512, 40.00000000000000000, 77.60416666578095146 ) ) ;
#27282=CARTESIAN_POINT ( 'NONE',  ( 3.763366191185776088, 40.00000000000000000, 57.39583333449059666 ) ) ;
#27313=CARTESIAN_POINT ( 'NONE',  ( 2.781618486875130358, 31.00000000000000355, -42.60416666509636485 ) ) ;
#27322=CARTESIAN_POINT ( 'NONE',  ( -47.94314659152439617, 40.00000000000000000, -16.27230485535717719 ) ) ;
#27323=CARTESIAN_POINT ( 'NONE',  ( -61.40313508883502891, 40.00000000000000711, 7.989450542818913092 ) ) ;
#27331=CARTESIAN_POINT ( 'NONE',  ( -18.08361268445098347, 40.00000000000000000, -10.43497034982449456 ) ) ;
#27350=CARTESIAN_POINT ( 'NONE',  ( 24.27443280711675300, 31.00000000000000355, -71.15176282235542260 ) ) ;
#27358=CARTESIAN_POINT ( 'NONE',  ( -59.98614492175870794, 40.00000000000000711, 68.21249229748744369 ) ) ;
#27369=CARTESIAN_POINT ( 'NONE',  ( -44.26264085333531995, 31.00000000000000711, 76.66224561662070869 ) ) ;
#27399=CARTESIAN_POINT ( 'NONE',  ( 46.89194940766294906, 31.00000000000000355, 6.259973086888626526 ) ) ;
#27406=CARTESIAN_POINT ( 'NONE',  ( 54.03410584561684971, 40.00000000000000000, 41.58544482236945328 ) ) ;
#27415=CARTESIAN_POINT ( 'NONE',  ( -46.87443272357899815, 31.00000000000000355, 35.96965017775951878 ) ) ;
#27425=CARTESIAN_POINT ( 'NONE',  ( -13.09503298281258132, 40.00000000000000000, -17.05789676611946959 ) ) ;
#27429=CARTESIAN_POINT ( 'NONE',  ( 51.69257347811147696, 31.00000000000000355, 59.10123636506271083 ) ) ;
#27430=CARTESIAN_POINT ( 'NONE',  ( -70.06919973880852126, 40.00000000000000711, -18.87919424805731339 ) ) ;
#27439=ORIENTED_EDGE ( 'NONE', *, *, #39160, .F. ) ;
#27444=CARTESIAN_POINT ( 'NONE',  ( 80.16187752211510542, 39.99999999999999289, -27.22680903928618434 ) ) ;
#27457=CARTESIAN_POINT ( 'NONE',  ( 6.473670811831357064, 40.00000000000000000, -24.11571013580714151 ) ) ;
#27459=DIRECTION ( 'NONE',  ( -0.06345332152672161774, 0.000000000000000000, 0.9979848074931934043 ) ) ;
#27468=CARTESIAN_POINT ( 'NONE',  ( 25.10416666396844576, 31.00000000000000355, 1.636246165087044124 ) ) ;
#27469=VERTEX_POINT ( 'NONE', #333 ) ;
#27478=CARTESIAN_POINT ( 'NONE',  ( -69.89583333424914713, 31.00000000000000711, 4.581489278091138040 ) ) ;
#27481=CARTESIAN_POINT ( 'NONE',  ( 36.58905133582347702, 31.00000000000000355, -27.97030060560319953 ) ) ;
#27483=CARTESIAN_POINT ( 'NONE',  ( -39.25113411183426848, 40.00000000000000000, 67.98392962655870519 ) ) ;
#27495=CARTESIAN_POINT ( 'NONE',  ( -59.89583333444493718, 40.00000000000000711, 3.926990808566372060 ) ) ;
#27529=CARTESIAN_POINT ( 'NONE',  ( -37.46020281470095625, 31.00000000000000355, 12.72710441276525017 ) ) ;
#27532=CARTESIAN_POINT ( 'NONE',  ( -101.9959696149863646, 35.50000000000000711, -0.1269066430510136789 ) ) ;
#27538=CARTESIAN_POINT ( 'NONE',  ( -47.99616210117395099, 40.00000000000000000, 12.86278070621785119 ) ) ;
#27540=CARTESIAN_POINT ( 'NONE',  ( 54.55067978551168295, 40.00000000000000000, 18.62288743479739495 ) ) ;
#27549=CARTESIAN_POINT ( 'NONE',  ( -26.30698076681265363, 40.00000000000000000, 12.97770382244945253 ) ) ;
#27554=CARTESIAN_POINT ( 'NONE',  ( -19.99999999999999645, 17.11489954122026447, 1.283214542831032867 ) ) ;
#27556=ORIENTED_EDGE ( 'NONE', *, *, #8574, .F. ) ;
#27565=CARTESIAN_POINT ( 'NONE',  ( -35.33737842959504150, 31.00000000000000355, 60.98257694382487415 ) ) ;
#27575=CARTESIAN_POINT ( 'NONE',  ( 96.90013369365227902, 39.99999999999999289, -6.223598210838602540 ) ) ;
#27589=CARTESIAN_POINT ( 'NONE',  ( 63.16980243745005907, 31.00000000000000000, -55.41789732285823078 ) ) ;
#27592=CARTESIAN_POINT ( 'NONE',  ( 18.71272080434063056, 40.00000000000000000, 21.38210947162712117 ) ) ;
#27624=CARTESIAN_POINT ( 'NONE',  ( 5.928665350384932253, 31.00000000000000355, -44.40877992884582426 ) ) ;
#27631=CARTESIAN_POINT ( 'NONE',  ( 58.81396797841472335, 40.00000000000000000, 34.08301911901634895 ) ) ;
#27641=FILL_AREA_STYLE_COLOUR ( '', #24028 ) ;
#27646=CARTESIAN_POINT ( 'NONE',  ( 48.77780477658175329, 31.00000000000000355, -24.05648398140741406 ) ) ;
#27653=CARTESIAN_POINT ( 'NONE',  ( -12.50349052776452297, 40.00000000000000000, 25.37591446456323041 ) ) ;
#27658=CARTESIAN_POINT ( 'NONE',  ( 37.84579180137232157, 31.00000000000000355, -65.31998993212283722 ) ) ;
#27659=CARTESIAN_POINT ( 'NONE',  ( 19.52887458859586900, 40.00000000000000000, -72.48875405283516216 ) ) ;
#27675=CARTESIAN_POINT ( 'NONE',  ( 24.08498528996878107, 40.00000000000000000, -89.94621034038658536 ) ) ;
#27690=CARTESIAN_POINT ( 'NONE',  ( -24.64063138600937464, 40.00000000000000000, 18.85097431370326859 ) ) ;
#27700=CARTESIAN_POINT ( 'NONE',  ( -7.231618336280544845, 31.00000000000000355, 27.02512817425793656 ) ) ;
#27709=CARTESIAN_POINT ( 'NONE',  ( 73.03870520561201829, 31.00000000000000000, -42.18585045165268355 ) ) ;
#27714=CARTESIAN_POINT ( 'NONE',  ( 46.49836147156941024, 31.00000000000000355, -6.043767708844123732 ) ) ;
#27716=CARTESIAN_POINT ( 'NONE',  ( -79.69263343296167079, 40.00000000000000711, -10.49242979028127820 ) ) ;
#27726=CARTESIAN_POINT ( 'NONE',  ( 54.85378563033546584, 40.00000000000000000, 7.219977902337870290 ) ) ;
#27749=CARTESIAN_POINT ( 'NONE',  ( -105.9879088449591933, 17.11489954122026447, -0.3807199291576673361 ) ) ;
#27761=CARTESIAN_POINT ( 'NONE',  ( 35.10416666475790493, 31.00000000000000355, 2.290744634698880233 ) ) ;
#27764=LINE ( 'NONE', #34711, #19300 ) ;
#27770=CARTESIAN_POINT ( 'NONE',  ( 41.10549127292548377, 40.00000000000000000, 20.25863663968860706 ) ) ;
#27771=CIRCLE ( 'NONE', #2640, 2.500000000000000444 ) ;
#27772=CARTESIAN_POINT ( 'NONE',  ( 27.80911911934546055, 40.00000000000000000, -47.97225535894359894 ) ) ;
#27774=CIRCLE ( 'NONE', #42364, 2.500000000000000444 ) ;
#27782=CARTESIAN_POINT ( 'NONE',  ( -3.620280825866593055, 40.00000000000000000, 27.53105304817175636 ) ) ;
#27796=CARTESIAN_POINT ( 'NONE',  ( -4.761419979751499554, 31.00000000000000355, -74.40007767863900767 ) ) ;
#27808=CARTESIAN_POINT ( 'NONE',  ( 6.309545988805658645, 40.00000000000000000, -94.59213238963913284 ) ) ;
#27817=CARTESIAN_POINT ( 'NONE',  ( 84.89583333414414312, 31.00000000000000000, -5.563236982362012029 ) ) ;
#27820=CARTESIAN_POINT ( 'NONE',  ( 27.10182830755125138, 40.00000000000000000, 1.799748011963437255 ) ) ;
#27846=CARTESIAN_POINT ( 'NONE',  ( -12.95950413119362743, 31.00000000000000355, 37.95406330259781669 ) ) ;
#27854=CARTESIAN_POINT ( 'NONE',  ( -28.16914340537297434, 40.00000000000000000, -57.36152490105313007 ) ) ;
#27864=SURFACE_SIDE_STYLE ('',( #17840 ) ) ;
#27867=CARTESIAN_POINT ( 'NONE',  ( -29.22812062908682051, 31.00000000000000355, 50.62729764625685647 ) ) ;
#27871=CARTESIAN_POINT ( 'NONE',  ( -29.44516979616424024, 40.00000000000000000, -7.879824757621473275 ) ) ;
#27872=ADVANCED_FACE ( 'NONE', ( #19997 ), #39833, .F. ) ;
#27877=CARTESIAN_POINT ( 'NONE',  ( 86.24314314301659579, 31.00000000000000000, -11.24622374123920920 ) ) ;
#27878=CARTESIAN_POINT ( 'NONE',  ( 77.59064570039033981, 39.99999999999999289, -38.12735739512951483 ) ) ;
#27889=CARTESIAN_POINT ( 'NONE',  ( -17.44537629401976631, 17.11489954122025736, -4.261559264950514958 ) ) ;
#27895=CARTESIAN_POINT ( 'NONE',  ( -55.79431841392906222, 40.00000000000000000, -72.71543055464235294 ) ) ;
#27908=CARTESIAN_POINT ( 'NONE',  ( 37.09854380388319584, 40.00000000000000000, 2.490183985263671129 ) ) ;
#27916=DIRECTION ( 'NONE',  ( 1.000000000000000000, 0.000000000000000000, 0.000000000000000000 ) ) ;
#27923=CARTESIAN_POINT ( 'NONE',  ( -18.92511213055653130, 31.00000000000000355, 21.58621387822740090 ) ) ;
#27928=CARTESIAN_POINT ( 'NONE',  ( -26.42126989340051324, 31.00000000000000355, -77.78956226056263290 ) ) ;
#27932=CARTESIAN_POINT ( 'NONE',  ( 3.791180027291366716, 31.00000000000000355, 59.39995347152935778 ) ) ;
#27936=CARTESIAN_POINT ( 'NONE',  ( -55.79431841392906222, 40.00000000000000000, -72.71543055464235294 ) ) ;
#27947=CARTESIAN_POINT ( 'NONE',  ( 61.18335543008118549, 39.99999999999999289, -20.78249587198964576 ) ) ;
#27961=CARTESIAN_POINT ( 'NONE',  ( -6.638544827991894159, 31.00000000000000355, 99.59190654106262741 ) ) ;
#27975=CARTESIAN_POINT ( 'NONE',  ( 42.89889459577944564, 31.00000000000000355, -32.91970121835214513 ) ) ;
#27987=CARTESIAN_POINT ( 'NONE',  ( 31.73387399974884104, 40.00000000000000000, -54.96645564127986461 ) ) ;
#27988=CARTESIAN_POINT ( 'NONE',  ( -3.469229457552012619, 40.00000000000000000, -54.39987425098301799 ) ) ;
#27996=CARTESIAN_POINT ( 'NONE',  ( -27.62299686580952240, 40.00000000000000000, -13.61136854378590577 ) ) ;
#28009=CARTESIAN_POINT ( 'NONE',  ( 51.69257347811147696, 31.00000000000000355, 59.10123636506271083 ) ) ;
#28017=CARTESIAN_POINT ( 'NONE',  ( -73.90312034494817794, 40.00000000000000711, -56.84521418463217657 ) ) ;
#28019=CARTESIAN_POINT ( 'NONE',  ( 22.27703560431448793, 31.00000000000000355, 17.12883495622356023 ) ) ;
#28033=CARTESIAN_POINT ( 'NONE',  ( 17.33436897218374639, 40.00000000000000000, 22.64673195036553111 ) ) ;
#28060=CARTESIAN_POINT ( 'NONE',  ( 10.06970066534735331, 31.00000000000000355, 37.84957806120349488 ) ) ;
#28067=CARTESIAN_POINT ( 'NONE',  ( 51.26988013557343749, 40.00000000000000000, 45.10883117380814866 ) ) ;
#28078=CARTESIAN_POINT ( 'NONE',  ( -48.53848235557606472, 31.00000000000000355, -37.22912483484027035 ) ) ;
#28087=CARTESIAN_POINT ( 'NONE',  ( -65.95487968126425926, 31.00000000000000711, -50.74205456613862708 ) ) ;
#28088=CARTESIAN_POINT ( 'NONE',  ( -78.26717753304431824, 40.00000000000000711, -26.69481836930730978 ) ) ;
#28095=EDGE_CURVE ( 'NONE', #40305, #9994, #38257, .T. ) ;
#28103=CARTESIAN_POINT ( 'NONE',  ( -68.67288961433401084, 40.00000000000000711, -60.22678404055071155 ) ) ;
#28116=CARTESIAN_POINT ( 'NONE',  ( -7.793954689940647995, 40.00000000000000000, 28.94896179907301459 ) ) ;
#28128=CARTESIAN_POINT ( 'NONE',  ( 21.81281596512078025, 31.00000000000000355, -10.76194779073239083 ) ) ;
#28133=CARTESIAN_POINT ( 'NONE',  ( -79.89583333417640176, 31.00000000000000711, 5.235987747608064957 ) ) ;
#28135=CARTESIAN_POINT ( 'NONE',  ( 18.91139405008774688, 31.00000000000000355, 55.99505798891475195 ) ) ;
#28136=CARTESIAN_POINT ( 'NONE',  ( 89.65113856817994531, 39.99999999999999289, -30.44896562292877462 ) ) ;
#28144=CARTESIAN_POINT ( 'NONE',  ( -101.9145453900123641, 31.00000000000000355, -1.407535261550449501 ) ) ;
#28152=CARTESIAN_POINT ( 'NONE',  ( 64.89583333437747115, 39.99999999999999289, -4.254240043327834009 ) ) ;
#28184=CARTESIAN_POINT ( 'NONE',  ( -32.14164714139042189, 31.00000000000000355, 36.65395011347077059 ) ) ;
#28190=CARTESIAN_POINT ( 'NONE',  ( 53.64558601427197004, 40.00000000000000000, 14.36188897069615500 ) ) ;
#28192=CARTESIAN_POINT ( 'NONE',  ( 33.95200755731382714, 40.00000000000000000, -44.10258293181757949 ) ) ;
#28195=CYLINDRICAL_SURFACE ( 'NONE', #17264, 2.500000000000000444 ) ;
#28204=CARTESIAN_POINT ( 'NONE',  ( 34.89583333524210218, 40.00000000000000000, -2.290744634698907767 ) ) ;
#28221=CARTESIAN_POINT ( 'NONE',  ( 17.81064159971323946, 31.00000000000000355, 66.89829513328324140 ) ) ;
#28232=CARTESIAN_POINT ( 'NONE',  ( -92.09225407318750456, 40.00000000000000711, -6.144973693751363264 ) ) ;
#28233=CARTESIAN_POINT ( 'NONE',  ( 7.507699080471219588, 31.00000000000000355, 28.16210111025598195 ) ) ;
#28245=CARTESIAN_POINT ( 'NONE',  ( 86.04713929520032423, 31.00000000000000000, 42.41619695850760507 ) ) ;
#28250=CARTESIAN_POINT ( 'NONE',  ( -18.31940394017777862, 40.00000000000000000, -14.05611420671344014 ) ) ;
#28252=EDGE_LOOP ( 'NONE', ( #26468, #13529, #19627, #34959 ) ) ;
#28273=DIRECTION ( 'NONE',  ( 0.000000000000000000, 1.000000000000000000, 0.000000000000000000 ) ) ;
#28279=CARTESIAN_POINT ( 'NONE',  ( 11.72132095739929625, 31.00000000000000355, -43.45763713126748229 ) ) ;
#28292=CARTESIAN_POINT ( 'NONE',  ( 16.92944795087012722, 40.00000000000000000, -62.81076020707057950 ) ) ;
#28296=CARTESIAN_POINT ( 'NONE',  ( -17.44537629401976275, 40.00000000000000000, 4.261559264950522063 ) ) ;
#28301=CARTESIAN_POINT ( 'NONE',  ( -61.47519263390311295, 31.00000000000000711, -35.49250405583519807 ) ) ;
#28313=CARTESIAN_POINT ( 'NONE',  ( -62.56443097448101298, 31.00000000000000355, -55.02758207457566897 ) ) ;
#28315=CARTESIAN_POINT ( 'NONE',  ( -74.30604906370724905, 40.00000000000000711, -36.76128443489604791 ) ) ;
#28328=CARTESIAN_POINT ( 'NONE',  ( -6.381360069252544953, 40.00000000000000000, 97.60416666604666602 ) ) ;
#28331=CARTESIAN_POINT ( 'NONE',  ( -15.99999999999997691, 31.00000000000000355, 5.571627607371296764E-15 ) ) ;
#28343=CARTESIAN_POINT ( 'NONE',  ( 12.72035051019986618, 40.00000000000000000, 25.87482915247129966 ) ) ;
#28358=CARTESIAN_POINT ( 'NONE',  ( -9.824444021593908616, 31.00000000000000355, 36.70529466175499778 ) ) ;
#28361=VECTOR ( 'NONE', #39349, 1000.000000000000000 ) ;
#28363=CARTESIAN_POINT ( 'NONE',  ( -51.96644965834242669, 31.00000000000000711, 59.25555446696338890 ) ) ;
#28366=CARTESIAN_POINT ( 'NONE',  ( -17.30549157494827384, 31.00000000000000355, -51.24895740946764988 ) ) ;
#28367=CARTESIAN_POINT ( 'NONE',  ( -6.054110834496889026, 40.00000000000000000, -92.39583333400220511 ) ) ;
#28382=CARTESIAN_POINT ( 'NONE',  ( 4.090615425948669781, 40.00000000000000000, -62.60416666561555132 ) ) ;
#28395=CIRCLE ( 'NONE', #6089, 4.500000000000000888 ) ;
#28413=CARTESIAN_POINT ( 'NONE',  ( -47.99616210117395099, 31.00000000000000355, 12.86278070621785119 ) ) ;
#28418=CARTESIAN_POINT ( 'NONE',  ( -54.58798567973315841, 40.00000000000000000, -26.90590473539369754 ) ) ;
#28419=CARTESIAN_POINT ( 'NONE',  ( -56.33579487689732446, 40.00000000000000000, -27.88694065509425357 ) ) ;
#28426=CARTESIAN_POINT ( 'NONE',  ( 2.965790448435745574, 31.00000000000000355, -22.56328348808469997 ) ) ;
#28429=CARTESIAN_POINT ( 'NONE',  ( 35.10416666475790493, 40.00000000000000000, 2.290744634698880233 ) ) ;
#28446=CARTESIAN_POINT ( 'NONE',  ( 25.34170449640226508, 31.00000000000000355, 74.97748276543396173 ) ) ;
#28454=CARTESIAN_POINT ( 'NONE',  ( -101.9959696149863788, 40.00000000000000711, -0.1269066430510139010 ) ) ;
#28470=CARTESIAN_POINT ( 'NONE',  ( 84.73112319332513209, 31.00000000000000000, -41.78253223598262167 ) ) ;
#28474=CARTESIAN_POINT ( 'NONE',  ( 25.13348990051749965, 40.00000000000000000, -8.510361017570636122 ) ) ;
#28505=CARTESIAN_POINT ( 'NONE',  ( 27.80911911935152503, 31.00000000000000355, -47.97225535896787108 ) ) ;
#28511=CARTESIAN_POINT ( 'NONE',  ( 57.21690105882998267, 39.99999999999999289, -50.04162206025958426 ) ) ;
#28521=CARTESIAN_POINT ( 'NONE',  ( 4.417864660711233959, 31.00000000000000355, 67.39583333436242185 ) ) ;
#28530=CARTESIAN_POINT ( 'NONE',  ( -82.09281090897877675, 31.00000000000000711, -5.486092462564049477 ) ) ;
#28531=CARTESIAN_POINT ( 'NONE',  ( 56.68048384767583769, 39.99999999999999289, -64.44707192207098956 ) ) ;
#28560=CARTESIAN_POINT ( 'NONE',  ( -26.24023198663969580, 40.00000000000000000, -20.19409642360271917 ) ) ;
#28569=CARTESIAN_POINT ( 'NONE',  ( 4.888094100070568437, 31.00000000000000355, 37.04995123692341252 ) ) ;
#28573=CARTESIAN_POINT ( 'NONE',  ( 73.00591898829820536, 31.00000000000000000, 19.54754034098114701 ) ) ;
#28577=CARTESIAN_POINT ( 'NONE',  ( -42.11670055801651102, 31.00000000000000355, -32.42481051985740237 ) ) ;
#28579=CARTESIAN_POINT ( 'NONE',  ( -54.00384411202717416, 40.00000000000000711, 70.40394205935166383 ) ) ;
#28590=CARTESIAN_POINT ( 'NONE',  ( -65.92798595308768483, 40.00000000000000711, 22.39357416381200849 ) ) ;
#28606=DIRECTION ( 'NONE',  ( 0.000000000000000000, 1.000000000000000000, -1.060184893785364939E-15 ) ) ;
#28616=CARTESIAN_POINT ( 'NONE',  ( -25.89845354150052259, 31.00000000000000355, -44.83417823681238445 ) ) ;
#28622=CARTESIAN_POINT ( 'NONE',  ( 25.16436199730139123, 40.00000000000000000, 51.02488717759543135 ) ) ;
#28633=CARTESIAN_POINT ( 'NONE',  ( -12.24460912605626106, 40.00000000000000000, 36.08157028455360660 ) ) ;
#28646=CARTESIAN_POINT ( 'NONE',  ( -60.98551593175036345, 31.00000000000000711, 53.34359504441579247 ) ) ;
#28658=CARTESIAN_POINT ( 'NONE',  ( 24.91045342551303321, 31.00000000000000355, 12.31387362277163433 ) ) ;
#28671=CARTESIAN_POINT ( 'NONE',  ( 74.70319961851696178, 31.00000000000000000, -57.31929289364909152 ) ) ;
#28675=CARTESIAN_POINT ( 'NONE',  ( -14.19360040536685830, 40.00000000000000000, 24.59234967646941783 ) ) ;
#28677=CARTESIAN_POINT ( 'NONE',  ( -32.60815990948594134, 40.00000000000000000, 24.92795611697640368 ) ) ;
#28706=CARTESIAN_POINT ( 'NONE',  ( 43.74200748489511881, 31.00000000000000355, 38.49442098324159645 ) ) ;
#28711=CARTESIAN_POINT ( 'NONE',  ( 74.15939217265263039, 39.99999999999999289, -19.75058139460558237 ) ) ;
#28719=DIRECTION ( 'NONE',  ( 0.000000000000000000, 0.000000000000000000, 1.000000000000000000 ) ) ;
#28727=CARTESIAN_POINT ( 'NONE',  ( 31.73387399974884104, 31.00000000000000355, -54.96645564127986461 ) ) ;
#28734=CARTESIAN_POINT ( 'NONE',  ( 5.735608225908778834, 31.00000000000000355, 89.40012361740336644 ) ) ;
#28735=CARTESIAN_POINT ( 'NONE',  ( -68.52217190868857699, 40.00000000000000711, 59.94826526062049510 ) ) ;
#28754=CARTESIAN_POINT ( 'NONE',  ( 26.10672890669568602, 31.00000000000000355, 8.893381768403882504 ) ) ;
#28759=DIRECTION ( 'NONE',  ( 0.000000000000000000, 1.541976423090494253E-15, 1.000000000000000000 ) ) ;
#28762=CARTESIAN_POINT ( 'NONE',  ( -37.12595630543398073, 40.00000000000000000, 18.22532657727797911 ) ) ;
#28776=CARTESIAN_POINT ( 'NONE',  ( -16.93500259178182432, 31.00000000000000355, 34.36424406943201149 ) ) ;
#28783=CARTESIAN_POINT ( 'NONE',  ( -84.90650804512098659, 31.00000000000000711, 28.83788733109305014 ) ) ;
#28785=CARTESIAN_POINT ( 'NONE',  ( -30.89738163651153258, 31.00000000000000355, 40.13100860029957317 ) ) ;
#28787=CARTESIAN_POINT ( 'NONE',  ( -72.39171112334068425, 40.00000000000000711, -55.52881859171880308 ) ) ;
#28798=CARTESIAN_POINT ( 'NONE',  ( -52.79687664379660816, 40.00000000000000000, -30.48099731442381710 ) ) ;
#28826=CARTESIAN_POINT ( 'NONE',  ( 39.77940265867437120, 31.00000000000000355, 22.96373720238702276 ) ) ;
#28832=CARTESIAN_POINT ( 'NONE',  ( 7.506055610550203205, 40.00000000000000000, 56.92102948000351148 ) ) ;
#28840=CARTESIAN_POINT ( 'NONE',  ( 22.22924588317381023, 40.00000000000000000, -25.35314793696836588 ) ) ;
#28853=CARTESIAN_POINT ( 'NONE',  ( -5.321195512787073589, 31.00000000000000355, 79.59297073838583003 ) ) ;
#28863=CARTESIAN_POINT ( 'NONE',  ( -17.43724119492662794, 31.00000000000000355, -15.29674861594511448 ) ) ;
#28867=CARTESIAN_POINT ( 'NONE',  ( -2.924622967158192921, 31.00000000000000355, -22.14664255385889291 ) ) ;
#28879=CARTESIAN_POINT ( 'NONE',  ( 3.579113344806025054, 40.00000000000000000, 27.11441211503905535 ) ) ;
#28881=CARTESIAN_POINT ( 'NONE',  ( 21.72498709343026846, 40.00000000000000000, -28.22316639787646864 ) ) ;
#28892=LINE ( 'NONE', #32576, #42475 ) ;
#28910=CARTESIAN_POINT ( 'NONE',  ( 24.55685208794459129, 31.00000000000000355, -49.59815698162134368 ) ) ;
#28917=CARTESIAN_POINT ( 'NONE',  ( -9.616483412535155040, 40.00000000000000000, -73.82325415887568454 ) ) ;
#28930=CARTESIAN_POINT ( 'NONE',  ( 38.75409931461306456, 31.00000000000000355, -50.52625141960567134 ) ) ;
#28940=CARTESIAN_POINT ( 'NONE',  ( 42.30527206516848082, 31.00000000000000355, -85.53883208674149330 ) ) ;
#28941=CARTESIAN_POINT ( 'NONE',  ( 76.36627019849126441, 39.99999999999999289, -58.43797548694632127 ) ) ;
#28950=VECTOR ( 'NONE', #16125, 999.9999999999998863 ) ;
#28970=CARTESIAN_POINT ( 'NONE',  ( -40.27082278478597033, 40.00000000000000000, 10.71261860272680977 ) ) ;
#28981=EDGE_CURVE ( 'NONE', #25259, #39678, #29584, .T. ) ;
#28987=CARTESIAN_POINT ( 'NONE',  ( -40.10416666498607441, 31.00000000000000355, -2.617993869485698344 ) ) ;
#28993=AXIS2_PLACEMENT_3D ( 'NONE', #16343, #26383, #42700 ) ;
#28994=CARTESIAN_POINT ( 'NONE',  ( 70.70367055548476287, 31.00000000000000000, -62.02616482874480397 ) ) ;
#28997=CARTESIAN_POINT ( 'NONE',  ( -61.79211991636739754, 31.00000000000000711, -8.240724169199884486 ) ) ;
#28998=CARTESIAN_POINT ( 'NONE',  ( 31.25450476884064699, 40.00000000000000000, 92.02345382966369414 ) ) ;
#29015=CARTESIAN_POINT ( 'NONE',  ( 19.99305134020393382, 40.00000000000000000, 74.61661993947731730 ) ) ;
#29045=CARTESIAN_POINT ( 'NONE',  ( -57.43240763726046794, 31.00000000000000355, -19.49446143887317717 ) ) ;
#29049=CARTESIAN_POINT ( 'NONE',  ( -47.15756294055117337, 40.00000000000000000, -53.75246728999482571 ) ) ;
#29061=CARTESIAN_POINT ( 'NONE',  ( 34.77048308403384169, 40.00000000000000000, 30.48958026498159768 ) ) ;
#29063=DIRECTION ( 'NONE',  ( -0.2604563316218753699, 0.000000000000000000, -0.9654856287475622745 ) ) ;
#29072=DIRECTION ( 'NONE',  ( 0.3211947320043963550, 0.000000000000000000, -0.9470131699890049770 ) ) ;
#29075=CARTESIAN_POINT ( 'NONE',  ( -65.95487968126425926, 31.00000000000000711, -50.74205456613862708 ) ) ;
#29076=ORIENTED_EDGE ( 'NONE', *, *, #30741, .F. ) ;
#29082=CARTESIAN_POINT ( 'NONE',  ( -101.9001375415117963, 40.00000000000000711, 6.549163350515033066 ) ) ;
#29088=ADVANCED_FACE ( 'NONE', ( #16074 ), #20432, .T. ) ;
#29091=CARTESIAN_POINT ( 'NONE',  ( -27.97094176822542977, 31.00000000000000355, 9.504947828999611659 ) ) ;
#29097=CARTESIAN_POINT ( 'NONE',  ( -23.46968090759046888, 40.00000000000000000, -20.57717900685300449 ) ) ;
#29099=CARTESIAN_POINT ( 'NONE',  ( -4.434938641671375414, 40.00000000000000000, -34.07637162044569834 ) ) ;
#29122=CARTESIAN_POINT ( 'NONE',  ( -81.55297449308174862, 40.00000000000000711, -40.20044092665353475 ) ) ;
#29130=CARTESIAN_POINT ( 'NONE',  ( 7.251580242022521716, 31.00000000000000355, -54.34182998361462325 ) ) ;
#29139=CARTESIAN_POINT ( 'NONE',  ( 58.79931003850258975, 40.00000000000000000, 51.72161244498203558 ) ) ;
#29151=CARTESIAN_POINT ( 'NONE',  ( -77.03666156126601550, 31.00000000000000711, 20.64125776147949409 ) ) ;
#29160=CARTESIAN_POINT ( 'NONE',  ( -30.16842255227261660, 31.00000000000000355, -89.21315370691763746 ) ) ;
#29162=CARTESIAN_POINT ( 'NONE',  ( -70.09526419943651376, 40.00000000000000711, -61.63891210109846241 ) ) ;
#29181=VERTEX_POINT ( 'NONE', #4228 ) ;
#29189=CARTESIAN_POINT ( 'NONE',  ( 46.49836147156941735, 40.00000000000000000, -6.043767708841586206 ) ) ;
#29201=CARTESIAN_POINT ( 'NONE',  ( -36.61132647064156487, 31.00000000000000355, -18.04288060775211378 ) ) ;
#29206=CARTESIAN_POINT ( 'NONE',  ( 24.08498528996878107, 31.00000000000000355, -89.94621034038658536 ) ) ;
#29209=CARTESIAN_POINT ( 'NONE',  ( -47.50570208456527155, 31.00000000000000355, -41.80188021843024160 ) ) ;
#29210=CARTESIAN_POINT ( 'NONE',  ( -28.16914340537297434, 40.00000000000000000, -57.36152490105313007 ) ) ;
#29211=CARTESIAN_POINT ( 'NONE',  ( 94.17930118497612568, 39.99999999999999289, -12.41473344271720691 ) ) ;
#29223=ORIENTED_EDGE ( 'NONE', *, *, #39160, .T. ) ;
#29224=CARTESIAN_POINT ( 'NONE',  ( 18.89933391970155085, 40.00000000000000000, -70.58587736658564893 ) ) ;
#29257=CARTESIAN_POINT ( 'NONE',  ( 55.68207322489292466, 31.00000000000000000, -32.16283696845439266 ) ) ;
#29260=CARTESIAN_POINT ( 'NONE',  ( 35.42814233785335176, 31.00000000000000355, -9.427541829740359702 ) ) ;
#29261=CARTESIAN_POINT ( 'NONE',  ( 18.89933391970155085, 40.00000000000000000, -70.58587736658564893 ) ) ;
#29268=CARTESIAN_POINT ( 'NONE',  ( -6.238242335983215092, 40.00000000000000000, 47.40213128959678102 ) ) ;
#29282=CARTESIAN_POINT ( 'NONE',  ( -50.81742119984753714, 31.00000000000000355, -66.42451308377114572 ) ) ;
#29297=ORIENTED_EDGE ( 'NONE', *, *, #2975, .F. ) ;
#29300=CARTESIAN_POINT ( 'NONE',  ( -28.96462450050677973, 31.00000000000000355, -9.827991688575851370 ) ) ;
#29308=CARTESIAN_POINT ( 'NONE',  ( 18.38119342899891961, 40.00000000000000000, 31.81670425098764099 ) ) ;
#29309=CARTESIAN_POINT ( 'NONE',  ( 35.58384423644164229, 40.00000000000000000, 12.14845634898874494 ) ) ;
#29337=CARTESIAN_POINT ( 'NONE',  ( -7.015336270751801884, 31.00000000000000355, -53.95087245963820521 ) ) ;
#29345=CARTESIAN_POINT ( 'NONE',  ( 24.27443280711675655, 40.00000000000000000, -71.15176282235543681 ) ) ;
#29352=CYLINDRICAL_SURFACE ( 'NONE', #3525, 4.500000000000002665 ) ;
#29358=CARTESIAN_POINT ( 'NONE',  ( 57.37208743749949491, 31.00000000000000355, 50.31438278193533620 ) ) ;
#29370=CARTESIAN_POINT ( 'NONE',  ( 47.87658044097961607, 31.00000000000000000, -82.67148682534870829 ) ) ;
#29371=CARTESIAN_POINT ( 'NONE',  ( -44.52253807734693680, 40.00000000000000000, 90.03212995793734308 ) ) ;
#29387=CARTESIAN_POINT ( 'NONE',  ( 16.96065435355024320, 31.00000000000000355, -19.31014141889295388 ) ) ;
#29395=CARTESIAN_POINT ( 'NONE',  ( 29.49207856986237530, 40.00000000000000000, 38.57905506995709288 ) ) ;
#29408=CARTESIAN_POINT ( 'NONE',  ( -31.39472673864601049, 31.00000000000000355, -40.91112553188754930 ) ) ;
#29414=CARTESIAN_POINT ( 'NONE',  ( 81.15556025174309696, 31.00000000000000000, 27.54985289775053658 ) ) ;
#29418=CARTESIAN_POINT ( 'NONE',  ( 8.965261019430212031, 31.00000000000000355, 68.85524230650666766 ) ) ;
#29419=CARTESIAN_POINT ( 'NONE',  ( -71.33925323115938966, 40.00000000000000711, 9.290813765102964084 ) ) ;
#29420=CARTESIAN_POINT ( 'NONE',  ( 92.36625196220676060, 39.99999999999999289, 24.73319171124347093 ) ) ;
#29433=CARTESIAN_POINT ( 'NONE',  ( 55.63593431945896839, 39.99999999999999289, -48.80962981700470493 ) ) ;
#29460=SHAPE_DEFINITION_REPRESENTATION ( #30124, #41895 ) ;
#29463=CARTESIAN_POINT ( 'NONE',  ( -59.82155519080263417, 31.00000000000000711, -7.874468279917395286 ) ) ;
#29468=CARTESIAN_POINT ( 'NONE',  ( -30.84436395684956977, 31.00000000000000355, -10.52363363425319243 ) ) ;
#29469=CARTESIAN_POINT ( 'NONE',  ( 58.80104710710317306, 39.99999999999999289, -45.11949705600698479 ) ) ;
#29476=CARTESIAN_POINT ( 'NONE',  ( -35.44024466369167925, 40.00000000000000000, -20.45798383175513635 ) ) ;
#29478=CARTESIAN_POINT ( 'NONE',  ( -100.0589655806010967, 17.11489954122028578, 21.59728106529621883 ) ) ;
#29490=CARTESIAN_POINT ( 'NONE',  ( 42.30527206516848082, 31.00000000000000355, -85.53883208674149330 ) ) ;
#29506=CARTESIAN_POINT ( 'NONE',  ( -17.40445659762299968, 31.00000000000000355, 22.69748452323785060 ) ) ;
#29513=CARTESIAN_POINT ( 'NONE',  ( -33.98628324864968420, 40.00000000000000000, 19.63407011443918293 ) ) ;
#29514=CARTESIAN_POINT ( 'NONE',  ( 17.75583184595346964, 40.00000000000000000, -30.63479189996225216 ) ) ;
#29521=AXIS2_PLACEMENT_3D ( 'NONE', #19965, #15818, #9030 ) ;
#29545=CARTESIAN_POINT ( 'NONE',  ( 63.11376326756305843, 31.00000000000000000, -21.32174659671377626 ) ) ;
#29552=AXIS2_PLACEMENT_3D ( 'NONE', #31344, #34161, #1426 ) ;
#29553=CARTESIAN_POINT ( 'NONE',  ( -79.74759331938361129, 40.00000000000000711, -21.47736420602193874 ) ) ;
#29565=CARTESIAN_POINT ( 'NONE',  ( 72.19657831791809599, 31.00000000000000000, -19.34484491892447622 ) ) ;
#29576=CARTESIAN_POINT ( 'NONE',  ( -86.84058463553202500, 31.00000000000000711, 29.36381822872188607 ) ) ;
#29577=CARTESIAN_POINT ( 'NONE',  ( -46.83686391397709770, 40.00000000000000000, -81.34213072392142863 ) ) ;
#29584=LINE ( 'NONE', #42858, #19312 ) ;
#29591=CIRCLE ( 'NONE', #37228, 4.500000000000002665 ) ;
#29607=CARTESIAN_POINT ( 'NONE',  ( -21.81649963859176822, 40.00000000000000000, -37.93159502954524243 ) ) ;
#29619=CARTESIAN_POINT ( 'NONE',  ( 43.15607885788778475, 31.00000000000000355, -11.56636786368396486 ) ) ;
#29626=CARTESIAN_POINT ( 'NONE',  ( 28.03234818517180216, 31.00000000000000355, 82.53419278363811884 ) ) ;
#29627=CIRCLE ( 'NONE', #17130, 1.999999999999998668 ) ;
#29630=CARTESIAN_POINT ( 'NONE',  ( 64.47787635702036368, 31.00000000000000000, -17.16423577041365789 ) ) ;
#29631=CARTESIAN_POINT ( 'NONE',  ( -8.314562429032193336, 40.00000000000000000, -63.88718494337742015 ) ) ;
#29633=CARTESIAN_POINT ( 'NONE',  ( -86.05617919112455638, 40.00000000000000711, 49.70311056393224192 ) ) ;
#29645=CARTESIAN_POINT ( 'NONE',  ( -47.90394619311608437, 40.00000000000000000, 62.45286580340285099 ) ) ;
#29660=EDGE_LOOP ( 'NONE', ( #22158, #31327, #21057, #30189 ) ) ;
#29678=CARTESIAN_POINT ( 'NONE',  ( -29.22812062908682051, 31.00000000000000355, 50.62729764625685647 ) ) ;
#29682=CARTESIAN_POINT ( 'NONE',  ( -2.659806967433831382, 31.00000000000000355, 39.59793253467758944 ) ) ;
#29683=CARTESIAN_POINT ( 'NONE',  ( -4.745113895469965648, 40.00000000000000000, -72.39583333427917466 ) ) ;
#29695=CARTESIAN_POINT ( 'NONE',  ( -18.51709390187839688, 40.00000000000000000, -37.54239277154294996 ) ) ;
#29707=CARTESIAN_POINT ( 'NONE',  ( -68.52217190868857699, 31.00000000000000711, 59.94826526066079708 ) ) ;
#29728=CARTESIAN_POINT ( 'NONE',  ( -1.799870782497340782, 31.00000000000000355, 27.60416666422008802 ) ) ;
#29737=CARTESIAN_POINT ( 'NONE',  ( -10.91816144241376563, 40.00000000000000000, -40.73603723627661566 ) ) ;
#29738=CARTESIAN_POINT ( 'NONE',  ( 45.06603723658675875, 40.00000000000000000, 15.38899812202754624 ) ) ;
#29752=DIRECTION ( 'NONE',  ( 0.000000000000000000, -1.000000000000000000, 5.297542245118643184E-16 ) ) ;
#29768=CARTESIAN_POINT ( 'NONE',  ( 66.90003082756123831, 31.00000000000000000, -4.275635516647131595 ) ) ;
#29773=ORIENTED_EDGE ( 'NONE', *, *, #6483, .F. ) ;
#29777=CARTESIAN_POINT ( 'NONE',  ( 76.16439905403352384, 39.99999999999999289, 44.11546174421767574 ) ) ;
#29782=DIRECTION ( 'NONE',  ( 0.000000000000000000, 0.000000000000000000, 1.000000000000000000 ) ) ;
#29792=CARTESIAN_POINT ( 'NONE',  ( -61.13902149641835138, 31.00000000000000355, -53.61851653479526902 ) ) ;
#29806=CARTESIAN_POINT ( 'NONE',  ( -61.59955500562279695, 31.00000000000000711, -70.40623950599746195 ) ) ;
#29826=CARTESIAN_POINT ( 'NONE',  ( -14.91913624998189469, 31.00000000000000355, -30.37684071746364012 ) ) ;
#29836=CARTESIAN_POINT ( 'NONE',  ( 7.251580242022520828, 40.00000000000000000, -54.34182998362662431 ) ) ;
#29846=CARTESIAN_POINT ( 'NONE',  ( 6.892732713553924917, 31.00000000000000355, -52.36990085009771434 ) ) ;
#29855=ADVANCED_FACE ( 'NONE', ( #16181 ), #25796, .T. ) ;
#29858=CARTESIAN_POINT ( 'NONE',  ( 86.04713929520032423, 31.00000000000000000, 42.41619695850760507 ) ) ;
#29860=VERTEX_POINT ( 'NONE', #39255 ) ;
#29864=CARTESIAN_POINT ( 'NONE',  ( -48.52617905695110068, 31.00000000000000355, 37.10499320822106029 ) ) ;
#29865=CARTESIAN_POINT ( 'NONE',  ( 4.329677741076332964, 40.00000000000000000, -64.59417075179260337 ) ) ;
#29866=CARTESIAN_POINT ( 'NONE',  ( -60.10374203099167545, 40.00000000000000711, 78.35501831527777483 ) ) ;
#29871=CARTESIAN_POINT ( 'NONE',  ( -15.99999999999997691, 31.00000000000000355, 5.571627607371296764E-15 ) ) ;
#29878=CARTESIAN_POINT ( 'NONE',  ( -5.726861599740728614, 40.00000000000000000, 87.60416666588449175 ) ) ;
#29884=ORIENTED_EDGE ( 'NONE', *, *, #30498, .T. ) ;
#29907=CARTESIAN_POINT ( 'NONE',  ( -53.27196957865878346, 31.00000000000000711, 26.27224001321920355 ) ) ;
#29910=CARTESIAN_POINT ( 'NONE',  ( 28.62564328229763788, 31.00000000000000355, -21.88780996306212501 ) ) ;
#29911=CARTESIAN_POINT ( 'NONE',  ( -60.02123122004734768, 40.00000000000000711, 34.66859033927303813 ) ) ;
#29921=CARTESIAN_POINT ( 'NONE',  ( -36.80126402429788612, 40.00000000000000000, 32.28896105221774349 ) ) ;
#29932=CARTESIAN_POINT ( 'NONE',  ( -55.31949386280458469, 31.00000000000000711, 71.91600076666669850 ) ) ;
#29936=VECTOR ( 'NONE', #9855, 1000.000000000000000 ) ;
#29948=CARTESIAN_POINT ( 'NONE',  ( -19.19493090124598922, 31.00000000000000355, -25.00897302100653263 ) ) ;
#29954=CARTESIAN_POINT ( 'NONE',  ( -38.45388554590046937, 40.00000000000000000, -13.05014827191142679 ) ) ;
#29955=CARTESIAN_POINT ( 'NONE',  ( -21.81649963859176822, 40.00000000000000000, -37.93159502954524243 ) ) ;
#29970=DIRECTION ( 'NONE',  ( 0.000000000000000000, 0.000000000000000000, -1.000000000000000000 ) ) ;
#29983=CARTESIAN_POINT ( 'NONE',  ( -61.40313508884858607, 31.00000000000000711, 7.989450542815522027 ) ) ;
#29990=CARTESIAN_POINT ( 'NONE',  ( 68.41293481152064260, 39.99999999999999289, -52.34142988144959219 ) ) ;
#30004=CARTESIAN_POINT ( 'NONE',  ( 70.67261647610648367, 31.00000000000000000, -24.00465245562410743 ) ) ;
#30011=ORIENTED_EDGE ( 'NONE', *, *, #36812, .T. ) ;
#30015=CARTESIAN_POINT ( 'NONE',  ( -101.1468392227577340, 31.00000000000000711, 13.20405500233197671 ) ) ;
#30035=CARTESIAN_POINT ( 'NONE',  ( -22.00208165626505519, 31.00000000000000355, -25.16137218361809502 ) ) ;
#30044=CARTESIAN_POINT ( 'NONE',  ( -3.469229457552012619, 40.00000000000000000, -54.39987425098301799 ) ) ;
#30048=ORIENTED_EDGE ( 'NONE', *, *, #30498, .F. ) ;
#30054=CARTESIAN_POINT ( 'NONE',  ( 28.83751338862256119, 31.00000000000000355, -32.88701605462710376 ) ) ;
#30061=CARTESIAN_POINT ( 'NONE',  ( -20.07939870814534089, 40.00000000000000000, -2.638545259751242877 ) ) ;
#30066=CARTESIAN_POINT ( 'NONE',  ( 47.76959191294547225, 31.00000000000000355, 62.44753968350421047 ) ) ;
#30067=CARTESIAN_POINT ( 'NONE',  ( -49.21613380539481142, 40.00000000000000000, 63.96793098899348706 ) ) ;
#30070=ORIENTED_EDGE ( 'NONE', *, *, #42019, .F. ) ;
#30079=CARTESIAN_POINT ( 'NONE',  ( -64.44063486737354651, 40.00000000000000711, -49.42892067282641477 ) ) ;
#30095=CARTESIAN_POINT ( 'NONE',  ( 27.02985023942251885, 40.00000000000000000, 3.586895573513070090 ) ) ;
#30110=CARTESIAN_POINT ( 'NONE',  ( -62.26029918285335896, 31.00000000000000711, 30.70375207684418228 ) ) ;
#30115=CARTESIAN_POINT ( 'NONE',  ( 32.62694724487210607, 31.00000000000000355, -16.02036196159510339 ) ) ;
#30117=CARTESIAN_POINT ( 'NONE',  ( -79.27599250299880396, 40.00000000000000711, 10.45126230984107707 ) ) ;
#30124=PRODUCT_DEFINITION_SHAPE ( 'NONE', 'NONE',  #32055 ) ;
#30126=CARTESIAN_POINT ( 'NONE',  ( 54.89583333452979730, 40.00000000000000000, -3.599741573803383332 ) ) ;
#30142=CARTESIAN_POINT ( 'NONE',  ( -56.91377077966711084, 31.00000000000000355, -74.37798324515208037 ) ) ;
#30158=CARTESIAN_POINT ( 'NONE',  ( 22.24487986055951083, 31.00000000000000355, 28.98451114863597766 ) ) ;
#30165=CARTESIAN_POINT ( 'NONE',  ( 21.71086051706764763, 40.00000000000000000, -37.60982366119799991 ) ) ;
#30166=CARTESIAN_POINT ( 'NONE',  ( 38.14553738578516828, 40.00000000000000000, 29.36968266378342207 ) ) ;
#30172=CARTESIAN_POINT ( 'NONE',  ( 11.86982580658625075, 40.00000000000000000, 24.05989836594520526 ) ) ;
#30188=CARTESIAN_POINT ( 'NONE',  ( -28.16914340538000161, 31.00000000000000355, -57.36152490105312296 ) ) ;
#30189=ORIENTED_EDGE ( 'NONE', *, *, #39490, .F. ) ;
#30197=CARTESIAN_POINT ( 'NONE',  ( -74.30604906370724905, 40.00000000000000711, -36.76128443489604791 ) ) ;
#30206=COLOUR_RGB ( '', 0.08235294, 0.09019608, 0.10196078) ;
#30209=CARTESIAN_POINT ( 'NONE',  ( -54.00384411200708712, 31.00000000000000711, 70.40394205939183792 ) ) ;
#30237=CARTESIAN_POINT ( 'NONE',  ( 32.80084743084299248, 31.00000000000000355, 19.01436317119123842 ) ) ;
#30243=ORIENTED_EDGE ( 'NONE', *, *, #10320, .F. ) ;
#30246=CARTESIAN_POINT ( 'NONE',  ( 21.53706125533296500, 40.00000000000000000, 43.87245753945351368 ) ) ;
#30258=CARTESIAN_POINT ( 'NONE',  ( -15.46676570949300000, 31.00000000000000355, 45.57083133015776610 ) ) ;
#30265=CARTESIAN_POINT ( 'NONE',  ( 17.96659372829068246, 40.00000000000000000, -15.76829228678407624 ) ) ;
#30270=CARTESIAN_POINT ( 'NONE',  ( -20.82795069773117547, 31.00000000000000355, 77.32795358076221248 ) ) ;
#30271=CARTESIAN_POINT ( 'NONE',  ( -77.35014290652780744, 40.00000000000000711, 26.14598721591455899 ) ) ;
#30288=CARTESIAN_POINT ( 'NONE',  ( -76.41092972884307244, 40.00000000000000711, -25.93877460596726436 ) ) ;
#30299=CARTESIAN_POINT ( 'NONE',  ( -1.587008504153756938, 40.00000000000000000, -24.39691638390478090 ) ) ;
#30320=CARTESIAN_POINT ( 'NONE',  ( -31.81163009274181519, 31.00000000000000355, -64.50738158386226928 ) ) ;
#30321=EDGE_CURVE ( 'NONE', #19359, #9181, #17265, .T. ) ;
#30324=CARTESIAN_POINT ( 'NONE',  ( -2.829072032612243159, 31.00000000000000355, -44.39959014221899025 ) ) ;
#30327=CARTESIAN_POINT ( 'NONE',  ( 41.75688748258168914, 40.00000000000000000, -72.32308762158416471 ) ) ;
#30336=CARTESIAN_POINT ( 'NONE',  ( -38.53741714288415210, 40.00000000000000000, -33.79371401777069650 ) ) ;
#30350=CARTESIAN_POINT ( 'NONE',  ( -83.29221842953128885, 31.00000000000000711, -41.19657635674187190 ) ) ;
#30368=CARTESIAN_POINT ( 'NONE',  ( -39.53383601736616271, 31.00000000000000355, 5.215339288884301538 ) ) ;
#30379=CARTESIAN_POINT ( 'NONE',  ( 43.15607885788778475, 40.00000000000000000, -11.56636786368396486 ) ) ;
#30380=CARTESIAN_POINT ( 'NONE',  ( -16.19793102918200134, 40.00000000000000000, 47.43702525406639836 ) ) ;
#30389=CARTESIAN_POINT ( 'NONE',  ( 21.81281596512078025, 40.00000000000000000, -10.76194779073239083 ) ) ;
#30409=CARTESIAN_POINT ( 'NONE',  ( 7.664524495375376389, 31.00000000000000355, 58.91906827746952757 ) ) ;
#30418=CARTESIAN_POINT ( 'NONE',  ( -81.66074000183850501, 40.00000000000000711, -10.87165890510346777 ) ) ;
#30427=CARTESIAN_POINT ( 'NONE',  ( 52.74436945453300041, 31.00000000000000355, 68.73989242669851762 ) ) ;
#30439=CARTESIAN_POINT ( 'NONE',  ( -66.59699903142619348, 31.00000000000000711, 75.74378954611491110 ) ) ;
#30459=CARTESIAN_POINT ( 'NONE',  ( 30.20675218207096790, 31.00000000000000355, 23.25504409023748309 ) ) ;
#30461=VECTOR ( 'NONE', #31569, 1000.000000000000000 ) ;
#30463=VECTOR ( 'NONE', #20836, 1000.000000000000000 ) ;
#30470=CARTESIAN_POINT ( 'NONE',  ( 38.48770111205618605, 40.00000000000000000, 44.02435964457617956 ) ) ;
#30472=CIRCLE ( 'NONE', #1164, 4.500000000000002665 ) ;
#30482=CARTESIAN_POINT ( 'NONE',  ( 32.65420139560029611, 31.00000000000000355, -42.57517516360295673 ) ) ;
#30486=PRODUCT ( 'Return Coil Spring', 'Return Coil Spring', '', ( #16612 ) ) ;
#30489=CARTESIAN_POINT ( 'NONE',  ( -19.76500330823589735, 40.00000000000000000, -5.286999072153966139 ) ) ;
#30494=CARTESIAN_POINT ( 'NONE',  ( 19.52887458859586545, 31.00000000000000355, -72.48875405280207929 ) ) ;
#30495=CARTESIAN_POINT ( 'NONE',  ( -4.761419979751499554, 40.00000000000000000, -74.40007767863900767 ) ) ;
#30498=EDGE_CURVE ( 'NONE', #33075, #16446, #30472, .T. ) ;
#30514=CARTESIAN_POINT ( 'NONE',  ( 41.75688748258168914, 40.00000000000000000, -72.32308762158416471 ) ) ;
#30525=CARTESIAN_POINT ( 'NONE',  ( 17.33436897218374639, 40.00000000000000000, 22.64673195036553111 ) ) ;
#30530=CARTESIAN_POINT ( 'NONE',  ( -19.99999999999999645, 40.00000000000000000, 0.000000000000000000 ) ) ;
#30540=CARTESIAN_POINT ( 'NONE',  ( 13.36968668718156295, 31.00000000000000355, 23.13838826010315941 ) ) ;
#30545=CARTESIAN_POINT ( 'NONE',  ( -100.0000000000000568, 31.00000000000000355, 2.687086664288074189E-12 ) ) ;
#30546=CARTESIAN_POINT ( 'NONE',  ( 64.89583333437747115, 31.00000000000000000, -4.254240043327834009 ) ) ;
#30549=CARTESIAN_POINT ( 'NONE',  ( -3.331996295684063192, 31.00000000000000355, 49.59602437330212865 ) ) ;
#30550=CARTESIAN_POINT ( 'NONE',  ( 36.87680687886029318, 40.00000000000000000, -74.81172728975037955 ) ) ;
#30564=CARTESIAN_POINT ( 'NONE',  ( 44.56294422764113250, 40.00000000000000000, 34.17917587534974189 ) ) ;
#30595=CARTESIAN_POINT ( 'NONE',  ( -4.929261580875707871, 31.00000000000000355, 37.46659216873931797 ) ) ;
#30601=CARTESIAN_POINT ( 'NONE',  ( 45.10416666515585860, 40.00000000000000000, 2.945243104263102651 ) ) ;
#30602=CARTESIAN_POINT ( 'NONE',  ( -19.32876798325328949, 40.00000000000000000, -39.37500834187648735 ) ) ;
#30610=CARTESIAN_POINT ( 'NONE',  ( 5.935205493550105516, 40.00000000000000000, -22.18504493031268865 ) ) ;
#30623=LINE ( 'NONE', #3732, #8614 ) ;
#30628=CARTESIAN_POINT ( 'NONE',  ( -9.616483412539254871, 31.00000000000000355, -73.82325415884287168 ) ) ;
#30635=DIRECTION ( 'NONE',  ( 0.000000000000000000, 0.000000000000000000, 1.000000000000000000 ) ) ;
#30638=CARTESIAN_POINT ( 'NONE',  ( -41.44813913998980581, 40.00000000000000000, -84.33308812960441969 ) ) ;
#30648=CARTESIAN_POINT ( 'NONE',  ( -11.47416535668642723, 31.00000000000000355, 87.14428777381637303 ) ) ;
#30674=CARTESIAN_POINT ( 'NONE',  ( -20.36888183406315278, 31.00000000000000355, -26.63352584488936614 ) ) ;
#30684=CARTESIAN_POINT ( 'NONE',  ( -26.81486728383016072, 40.00000000000000000, -46.61672233255473685 ) ) ;
#30695=CARTESIAN_POINT ( 'NONE',  ( -59.40491426035100631, 31.00000000000000711, 7.833300799371349932 ) ) ;
#30700=CARTESIAN_POINT ( 'NONE',  ( -99.14707074559267141, 31.00000000000000711, 13.06922382031732610 ) ) ;
#30706=CARTESIAN_POINT ( 'NONE',  ( 66.15140951848846385, 31.00000000000000000, -38.07406969931856366 ) ) ;
#30707=CARTESIAN_POINT ( 'NONE',  ( -10.54315780146311532, 40.00000000000000000, 79.17709703063971460 ) ) ;
#30717=CARTESIAN_POINT ( 'NONE',  ( -105.9879088449591933, 31.00000000000000355, -0.3807199291576673361 ) ) ;
#30720=CARTESIAN_POINT ( 'NONE',  ( 10.81967497908702214, 40.00000000000000000, -82.17651821321413763 ) ) ;
#30737=CARTESIAN_POINT ( 'NONE',  ( -22.00000000000000000, 31.00000000000000355, 1.283214542831021765 ) ) ;
#30741=EDGE_CURVE ( 'NONE', #14757, #37436, #25434, .T. ) ;
#30746=CARTESIAN_POINT ( 'NONE',  ( 4.274771203358150196, 31.00000000000000355, -32.49882260841580006 ) ) ;
#30752=CARTESIAN_POINT ( 'NONE',  ( -65.92798595308768483, 31.00000000000000711, 22.39357416381200849 ) ) ;
#30754=CARTESIAN_POINT ( 'NONE',  ( -5.720710522141557952, 31.00000000000000355, -44.01410879003383059 ) ) ;
#30755=CARTESIAN_POINT ( 'NONE',  ( 65.81435062899562638, 39.99999999999999289, 37.99825742656441463 ) ) ;
#30769=CARTESIAN_POINT ( 'NONE',  ( 14.80739997004469366, 40.00000000000000000, 55.25628696611591550 ) ) ;
#30782=CARTESIAN_POINT ( 'NONE',  ( -91.07534658258107640, 31.00000000000000711, 44.76935032132903558 ) ) ;
#30798=CARTESIAN_POINT ( 'NONE',  ( 38.32544124395173668, 31.00000000000000355, -22.13982348525413002 ) ) ;
#30806=CARTESIAN_POINT ( 'NONE',  ( -45.59965607524345899, 40.00000000000000000, -22.47439267160796916 ) ) ;
#30807=CARTESIAN_POINT ( 'NONE',  ( 54.79583221321230724, 40.00000000000000000, -14.58025558542526490 ) ) ;
#30816=CARTESIAN_POINT ( 'NONE',  ( -25.30796725786148826, 40.00000000000000000, 14.62256337265529815 ) ) ;
#30835=CARTESIAN_POINT ( 'NONE',  ( 61.98103557012429121, 31.00000000000000000, 47.69015029125303329 ) ) ;
#30842=CARTESIAN_POINT ( 'NONE',  ( -70.09526419943651376, 40.00000000000000711, -61.63891210109846241 ) ) ;
#30852=CARTESIAN_POINT ( 'NONE',  ( -22.78857244739539212, 31.00000000000000355, 85.10612709700112077 ) ) ;
#30853=EDGE_CURVE ( 'NONE', #40305, #31476, #37883, .T. ) ;
#30856=CARTESIAN_POINT ( 'NONE',  ( -24.64063138600937464, 40.00000000000000000, 18.85097431370326859 ) ) ;
#30883=CARTESIAN_POINT ( 'NONE',  ( -28.59133019391535768, 31.00000000000000355, -32.71076623427349261 ) ) ;
#30889=CARTESIAN_POINT ( 'NONE',  ( -61.79211991639481028, 40.00000000000000711, -8.240724169186190551 ) ) ;
#30893=CARTESIAN_POINT ( 'NONE',  ( -15.99999999999997691, 40.00000000000000000, 2.500000000000006217 ) ) ;
#30897=CARTESIAN_POINT ( 'NONE',  ( 51.69409438402072965, 31.00000000000000355, -17.56033928829605273 ) ) ;
#30904=CARTESIAN_POINT ( 'NONE',  ( -10.31048697494744815, 40.00000000000000000, -30.34325702988586215 ) ) ;
#30908=CARTESIAN_POINT ( 'NONE',  ( 46.16409756963976463, 31.00000000000000355, -59.99419878592187416 ) ) ;
#30909=CARTESIAN_POINT ( 'NONE',  ( 5.085823974618865151, 40.00000000000000000, 79.40009828669005287 ) ) ;
#30926=CARTESIAN_POINT ( 'NONE',  ( 25.17870271038170316, 40.00000000000000000, 93.97695291299892517 ) ) ;
#30936=CIRCLE ( 'NONE', #42058, 2.500000000000002665 ) ;
#30940=CARTESIAN_POINT ( 'NONE',  ( -13.43146050690766735, 40.00000000000000000, 27.15249184974963015 ) ) ;
#30942=PLANE ( 'NONE',  #7297 ) ;
#30952=CARTESIAN_POINT ( 'NONE',  ( 10.28773449565296083, 31.00000000000000355, -20.88174966193524895 ) ) ;
#30958=CARTESIAN_POINT ( 'NONE',  ( 48.66231590553977071, 31.00000000000000000, -55.48862040801125062 ) ) ;
#30961=CARTESIAN_POINT ( 'NONE',  ( 45.87644943786595064, 31.00000000000000355, 12.37342411884007376 ) ) ;
#30963=CARTESIAN_POINT ( 'NONE',  ( 10.12401712103624263, 40.00000000000000000, 76.79210772277129138 ) ) ;
#30969=EDGE_CURVE ( 'NONE', #33557, #10195, #30623, .T. ) ;
#30972=DIRECTION ( 'NONE',  ( -0.000000000000000000, 5.297542245118643184E-16, 1.000000000000000000 ) ) ;
#30976=CARTESIAN_POINT ( 'NONE',  ( -22.94860596549062848, 40.00000000000000000, -46.53072237555588231 ) ) ;
#31008=CARTESIAN_POINT ( 'NONE',  ( -38.45388554590046937, 31.00000000000000355, -13.05014827191142679 ) ) ;
#31014=AXIS2_PLACEMENT_3D ( 'NONE', #16409, #9402, #23189 ) ;
#31016=CARTESIAN_POINT ( 'NONE',  ( 23.58227068755204314, 40.00000000000000000, -47.84673847638903510 ) ) ;
#31019=CARTESIAN_POINT ( 'NONE',  ( -45.90931453312558119, 40.00000000000000000, 40.13788153756827626 ) ) ;
#31030=CARTESIAN_POINT ( 'NONE',  ( 14.35450763783260797, 40.00000000000000000, -18.72194639494853874 ) ) ;
#31039=LINE ( 'NONE', #40399, #30463 ) ;
#31044=CARTESIAN_POINT ( 'NONE',  ( -71.33925323112771366, 31.00000000000000711, 9.290813765106920030 ) ) ;
#31054=CARTESIAN_POINT ( 'NONE',  ( -61.59955500558135100, 40.00000000000000711, -70.40623950603891501 ) ) ;
#31068=CARTESIAN_POINT ( 'NONE',  ( 66.75212336275305347, 31.00000000000000000, -51.21939497476837744 ) ) ;
#31072=CARTESIAN_POINT ( 'NONE',  ( 21.18498618631003438, 40.00000000000000000, 18.62224443192851098 ) ) ;
#31086=EDGE_LOOP ( 'NONE', ( #35996, #34686, #13132, #17000 ) ) ;
#31098=CARTESIAN_POINT ( 'NONE',  ( -105.9879088449591933, 31.00000000000000355, -0.3807199291576673361 ) ) ;
#31102=CARTESIAN_POINT ( 'NONE',  ( -26.44890248586417414, 31.00000000000000355, -34.59877114778963403 ) ) ;
#31107=CARTESIAN_POINT ( 'NONE',  ( -61.89998375879795844, 40.00000000000000711, 3.952486745199417673 ) ) ;
#31121=PRESENTATION_STYLE_ASSIGNMENT (( #6947 ) ) ;
#31125=CARTESIAN_POINT ( 'NONE',  ( 54.43714469963884284, 31.00000000000000355, -7.178810421751046000 ) ) ;
#31132=CARTESIAN_POINT ( 'NONE',  ( 26.99674208481366833, 40.00000000000000000, -20.71990538090019029 ) ) ;
#31136=CARTESIAN_POINT ( 'NONE',  ( 44.33290732825512492, 31.00000000000000355, 77.00207852755224280 ) ) ;
#31137=CARTESIAN_POINT ( 'NONE',  ( -62.56443097449947288, 40.00000000000000000, -55.02758207457567607 ) ) ;
#31154=CARTESIAN_POINT ( 'NONE',  ( -45.94448050778635917, 40.00000000000000000, -79.54744219826071117 ) ) ;
#31167=CARTESIAN_POINT ( 'NONE',  ( 9.304442065600174061, 40.00000000000000000, 27.50946418541003169 ) ) ;
#31182=CARTESIAN_POINT ( 'NONE',  ( -27.97094176822542977, 31.00000000000000355, 9.504947828999611659 ) ) ;
#31185=LINE ( 'NONE', #14176, #24634 ) ;
#31190=CARTESIAN_POINT ( 'NONE',  ( -53.76583044639610165, 31.00000000000000355, -61.28633540801820345 ) ) ;
#31193=CARTESIAN_POINT ( 'NONE',  ( -42.09738266246711191, 31.00000000000000355, -2.828681863544771691 ) ) ;
#31195=CARTESIAN_POINT ( 'NONE',  ( 68.41617299536980568, 39.99999999999999289, 52.47886963225217016 ) ) ;
#31206=CARTESIAN_POINT ( 'NONE',  ( -27.38011802910879311, 40.00000000000000000, -55.51905197969063011 ) ) ;
#31238=CARTESIAN_POINT ( 'NONE',  ( 6.892732713553924917, 31.00000000000000355, -52.36990085009771434 ) ) ;
#31246=CARTESIAN_POINT ( 'NONE',  ( -12.41726970680908515, 40.00000000000000000, 46.38546114896210071 ) ) ;
#31248=CARTESIAN_POINT ( 'NONE',  ( -42.11670055800494339, 40.00000000000000000, -32.42481051986320040 ) ) ;
#31255=CARTESIAN_POINT ( 'NONE',  ( -14.11622541012940601, 31.00000000000000355, -16.08312669853564358 ) ) ;
#31257=CARTESIAN_POINT ( 'NONE',  ( -37.46020281470095625, 40.00000000000000000, 12.72710441276525017 ) ) ;
#31269=CARTESIAN_POINT ( 'NONE',  ( 73.52353481979008620, 31.00000000000000000, 25.08131146961490998 ) ) ;
#31281=CARTESIAN_POINT ( 'NONE',  ( -88.68107738130200346, 40.00000000000000711, 23.63280646693861087 ) ) ;
#31282=CARTESIAN_POINT ( 'NONE',  ( 22.71825314374493487, 31.00000000000000355, -13.09499307598873585 ) ) ;
#31293=CARTESIAN_POINT ( 'NONE',  ( -96.39699453480135105, 31.00000000000000711, 25.82690913164849889 ) ) ;
#31296=CARTESIAN_POINT ( 'NONE',  ( 11.19416946702162718, 40.00000000000000000, -22.66942529387992522 ) ) ;
#31308=EDGE_LOOP ( 'NONE', ( #34947, #40825, #26043, #15884 ) ) ;
#31322=CARTESIAN_POINT ( 'NONE',  ( -30.82418422902937039, 31.00000000000000355, 26.94311707098126618 ) ) ;
#31327=ORIENTED_EDGE ( 'NONE', *, *, #10934, .T. ) ;
#31328=DIRECTION ( 'NONE',  ( 0.000000000000000000, 0.000000000000000000, 1.000000000000000000 ) ) ;
#31329=CARTESIAN_POINT ( 'NONE',  ( -59.29355402628473826, 40.00000000000000000, -20.23837177251483155 ) ) ;
#31343=CARTESIAN_POINT ( 'NONE',  ( -52.79687664379660816, 31.00000000000000355, -30.48099731442381710 ) ) ;
#31344=CARTESIAN_POINT ( 'NONE',  ( -30.61154013076160751, 17.11489954122029289, 25.77968906985393716 ) ) ;
#31350=CARTESIAN_POINT ( 'NONE',  ( 86.62806645044915399, 31.00000000000000000, 11.52843970785434990 ) ) ;
#31351=CARTESIAN_POINT ( 'NONE',  ( -11.85673204381699364, 40.00000000000000000, 89.11174773313419450 ) ) ;
#31367=CARTESIAN_POINT ( 'NONE',  ( 89.65113856817994531, 39.99999999999999289, -30.44896562292877462 ) ) ;
#31371=DIRECTION ( 'NONE',  ( -0.9247238835424298475, -2.016449031586420221E-16, -0.3806385939525924744 ) ) ;
#31380=CARTESIAN_POINT ( 'NONE',  ( 2.319640971205140900, 40.00000000000000000, -34.59922639972668890 ) ) ;
#31394=CARTESIAN_POINT ( 'NONE',  ( 19.04566582976364941, 31.00000000000000355, -14.62000746238684989 ) ) ;
#31400=CARTESIAN_POINT ( 'NONE',  ( -80.10416666582359824, 31.00000000000000711, -5.235987747607834031 ) ) ;
#31403=CARTESIAN_POINT ( 'NONE',  ( 46.08863070263671347, 31.00000000000000355, 35.47900410130831972 ) ) ;
#31404=CARTESIAN_POINT ( 'NONE',  ( -12.08748825390017068, 40.00000000000000000, -91.69541640458645304 ) ) ;
#31412=EDGE_CURVE ( 'NONE', #38968, #6578, #15311, .T. ) ;
#31420=CARTESIAN_POINT ( 'NONE',  ( 4.417864660711233959, 40.00000000000000000, 67.39583333436242185 ) ) ;
#31447=CARTESIAN_POINT ( 'NONE',  ( 54.43714469963884284, 31.00000000000000355, -7.178810421751046000 ) ) ;
#31457=CARTESIAN_POINT ( 'NONE',  ( 14.80739997004469366, 40.00000000000000000, 55.25628696611591550 ) ) ;
#31458=CARTESIAN_POINT ( 'NONE',  ( 46.08863070263672057, 40.00000000000000000, 35.47900410130833393 ) ) ;
#31465=CARTESIAN_POINT ( 'NONE',  ( 5.935205493550105516, 31.00000000000000355, -22.18504493031268865 ) ) ;
#31469=CARTESIAN_POINT ( 'NONE',  ( 4.274771203358150196, 40.00000000000000000, -32.49882260841580006 ) ) ;
#31476=VERTEX_POINT ( 'NONE', #39221 ) ;
#31484=CARTESIAN_POINT ( 'NONE',  ( -19.10382689932575673, 31.00000000000000355, -71.73905014346600240 ) ) ;
#31492=CARTESIAN_POINT ( 'NONE',  ( 44.33290732825513203, 40.00000000000000000, 77.00207852759155003 ) ) ;
#31493=CARTESIAN_POINT ( 'NONE',  ( 12.70938237924789327, 31.00000000000000355, -21.97768283340561979 ) ) ;
#31503=CARTESIAN_POINT ( 'NONE',  ( 24.08498528996878107, 31.00000000000000355, -89.94621034038658536 ) ) ;
#31505=VERTEX_POINT ( 'NONE', #9348 ) ;
#31506=CARTESIAN_POINT ( 'NONE',  ( -30.58448433907587827, 40.00000000000000000, 8.146263651249089577 ) ) ;
#31534=CARTESIAN_POINT ( 'NONE',  ( 42.86166521170756027, 31.00000000000000355, 21.22462828018744219 ) ) ;
#31540=CARTESIAN_POINT ( 'NONE',  ( -54.47698434027259395, 40.00000000000000000, -31.57393205620729404 ) ) ;
#31551=CARTESIAN_POINT ( 'NONE',  ( 59.08215048199704711, 31.00000000000000000, 29.12166076728773589 ) ) ;
#31558=CARTESIAN_POINT ( 'NONE',  ( -81.27520743792995006, 31.00000000000000711, 10.59408403752164851 ) ) ;
#31559=CARTESIAN_POINT ( 'NONE',  ( -92.09225407318750456, 40.00000000000000711, -6.144973693751363264 ) ) ;
#31569=DIRECTION ( 'NONE',  ( 0.000000000000000000, 1.000000000000000000, 0.000000000000000000 ) ) ;
#31575=CARTESIAN_POINT ( 'NONE',  ( -86.05617919112455638, 40.00000000000000711, 49.70311056393224192 ) ) ;
#31588=CARTESIAN_POINT ( 'NONE',  ( 3.798394181604433761, 40.00000000000000000, 29.10671710469611284 ) ) ;
#31593=DIRECTION ( 'NONE',  ( 0.000000000000000000, -1.000000000000000000, 5.297542245118643184E-16 ) ) ;
#31594=ORIENTED_EDGE ( 'NONE', *, *, #5750, .T. ) ;
#31599=CARTESIAN_POINT ( 'NONE',  ( -39.12533628356670334, 31.00000000000000355, -10.47265044290268499 ) ) ;
#31604=CARTESIAN_POINT ( 'NONE',  ( 24.81019160154284720, 31.00000000000000355, 73.04493173762017477 ) ) ;
#31606=CARTESIAN_POINT ( 'NONE',  ( -26.77709713317330653, 31.00000000000000355, 54.08981485145582013 ) ) ;
#31607=CARTESIAN_POINT ( 'NONE',  ( 85.10416666585589951, 39.99999999999999289, 5.563236982362346872 ) ) ;
#31623=CARTESIAN_POINT ( 'NONE',  ( -8.160545988181935328, 40.00000000000000000, -61.88879904071598048 ) ) ;
#31638=CARTESIAN_POINT ( 'NONE',  ( -15.99999999999997691, 40.00000000000000000, 5.571627607371296764E-15 ) ) ;
#31656=CARTESIAN_POINT ( 'NONE',  ( 6.197074855318628117, 31.00000000000000355, 46.98549035852928313 ) ) ;
#31661=CARTESIAN_POINT ( 'NONE',  ( -35.70415035507907930, 40.00000000000000000, 46.55071329160319493 ) ) ;
#31663=CARTESIAN_POINT ( 'NONE',  ( -49.80813925210025417, 40.00000000000000000, -17.00652635548005520 ) ) ;
#31669=CARTESIAN_POINT ( 'NONE',  ( 19.04566582976364941, 31.00000000000000355, -14.62000746238684989 ) ) ;
#31673=CARTESIAN_POINT ( 'NONE',  ( 8.528031178950213231, 40.00000000000000000, -31.86521141804621493 ) ) ;
#31685=AXIS2_PLACEMENT_3D ( 'NONE', #24628, #24853, #37880 ) ;
#31688=CARTESIAN_POINT ( 'NONE',  ( -41.82916961767931951, 31.00000000000000355, -72.66191475361131324 ) ) ;
#31697=CARTESIAN_POINT ( 'NONE',  ( -3.925388345519843725, 31.00000000000000355, 29.51202942214661462 ) ) ;
#31712=CARTESIAN_POINT ( 'NONE',  ( 92.36625196220676060, 31.00000000000000000, 24.73319171124347093 ) ) ;
#31716=CARTESIAN_POINT ( 'NONE',  ( 9.304442065600174061, 40.00000000000000000, 27.50946418541003169 ) ) ;
#31748=CARTESIAN_POINT ( 'NONE',  ( 20.11321884379921343, 31.00000000000000355, -40.61652209561064097 ) ) ;
#31757=CARTESIAN_POINT ( 'NONE',  ( -22.66037885604484359, 40.00000000000000000, 66.40833514169634100 ) ) ;
#31767=CARTESIAN_POINT ( 'NONE',  ( 20.30000058474805869, 31.00000000000000355, -59.80472289869057789 ) ) ;
#31782=CARTESIAN_POINT ( 'NONE',  ( 58.29702017945731285, 31.00000000000000000, 66.63806913872474524 ) ) ;
#31784=CARTESIAN_POINT ( 'NONE',  ( -71.82650799747224823, 40.00000000000000711, -41.60779115366585756 ) ) ;
#31788=ADVANCED_BREP_SHAPE_REPRESENTATION ( '', ( #42324, #13552 ), #18474 ) ;
#31791=ORIENTED_EDGE ( 'NONE', *, *, #4195, .F. ) ;
#31796=DIRECTION ( 'NONE',  ( 0.000000000000000000, -1.000000000000000000, 5.297542245118643184E-16 ) ) ;
#31813=CARTESIAN_POINT ( 'NONE',  ( -2.197745971917953511, 40.00000000000000000, -34.39891587002171747 ) ) ;
#31826=CARTESIAN_POINT ( 'NONE',  ( -37.46020281470095625, 31.00000000000000355, 12.72710441276525017 ) ) ;
#31832=CARTESIAN_POINT ( 'NONE',  ( -36.24314215638268877, 31.00000000000000355, -73.49571118816069770 ) ) ;
#31836=CARTESIAN_POINT ( 'NONE',  ( 17.81483206087466442, 31.00000000000000355, -52.17936214187551514 ) ) ;
#31837=CARTESIAN_POINT ( 'NONE',  ( -80.23695839127151430, 40.00000000000000711, 39.56677620416681407 ) ) ;
#31851=CARTESIAN_POINT ( 'NONE',  ( -45.35818215263140019, 40.00000000000000000, 51.72168634911185592 ) ) ;
#31872=AXIS2_PLACEMENT_3D ( 'NONE', #39597, #81, #36321 ) ;
#31879=EDGE_CURVE ( 'NONE', #25968, #11466, #29591, .T. ) ;
#31881=CARTESIAN_POINT ( 'NONE',  ( 23.58227068755204314, 31.00000000000000355, -47.84673847638903510 ) ) ;
#31888=CARTESIAN_POINT ( 'NONE',  ( 52.68777711438346500, 40.00000000000000000, 17.88338314711659294 ) ) ;
#31893=CARTESIAN_POINT ( 'NONE',  ( 14.35450763783260797, 31.00000000000000355, -18.72194639494853874 ) ) ;
#31897=CARTESIAN_POINT ( 'NONE',  ( 2.454369252093185239, 40.00000000000000000, 37.39583333513270702 ) ) ;
#31913=ORIENTED_EDGE ( 'NONE', *, *, #22193, .T. ) ;
#31915=CARTESIAN_POINT ( 'NONE',  ( -21.69137426901471954, 31.00000000000000355, -81.42030341110597647 ) ) ;
#31922=CARTESIAN_POINT ( 'NONE',  ( 26.53203760875093309, 31.00000000000000355, 7.134992448514335450 ) ) ;
#31936=CARTESIAN_POINT ( 'NONE',  ( -6.381360069252544953, 31.00000000000000355, 97.60416666604666602 ) ) ;
#31941=CARTESIAN_POINT ( 'NONE',  ( -28.63582912838407069, 40.00000000000000000, 7.677129336082076705 ) ) ;
#31942=CARTESIAN_POINT ( 'NONE',  ( -35.75974951333986240, 40.00000000000000000, 20.56794350806610794 ) ) ;
#31971=CARTESIAN_POINT ( 'NONE',  ( 51.84393115708665079, 31.00000000000000355, 25.66707601012906892 ) ) ;
#31976=CARTESIAN_POINT ( 'NONE',  ( 34.31975892712151222, 40.00000000000000000, 59.64049725130580271 ) ) ;
#31984=CARTESIAN_POINT ( 'NONE',  ( -54.82550897924149069, 31.00000000000000711, 42.06954809655981364 ) ) ;
#31989=CIRCLE ( 'NONE', #22958, 4.500000000000002665 ) ;
#31994=CARTESIAN_POINT ( 'NONE',  ( -5.410573124821301150, 31.00000000000000355, -84.40011308935179102 ) ) ;
#31995=CARTESIAN_POINT ( 'NONE',  ( -26.95034633362163845, 40.00000000000000000, -79.72278128421112342 ) ) ;
#32013=CARTESIAN_POINT ( 'NONE',  ( 27.10182830755124428, 31.00000000000000355, 1.799748011963437033 ) ) ;
#32024=CARTESIAN_POINT ( 'NONE',  ( 19.31996883371318674, 40.00000000000000000, 33.58758284028577634 ) ) ;
#32034=CARTESIAN_POINT ( 'NONE',  ( 14.71924655979513297, 31.00000000000000355, -29.87007926703815741 ) ) ;
#32040=CARTESIAN_POINT ( 'NONE',  ( 55.27058341129635721, 31.00000000000000000, -63.02248852588876105 ) ) ;
#32043=CARTESIAN_POINT ( 'NONE',  ( 29.31577600746836154, 31.00000000000000355, 50.95836110721448620 ) ) ;
#32044=CARTESIAN_POINT ( 'NONE',  ( 46.76839422406115432, 39.99999999999999289, -81.00140361174831583 ) ) ;
#32045=ORIENTED_EDGE ( 'NONE', *, *, #3610, .F. ) ;
#32050=ORIENTED_EDGE ( 'NONE', *, *, #22193, .F. ) ;
#32055=PRODUCT_DEFINITION ( 'UNKNOWN', '', #20536, #3803 ) ;
#32057=CARTESIAN_POINT ( 'NONE',  ( -62.26029918285335896, 40.00000000000000711, 30.70375207684418228 ) ) ;
#32086=CARTESIAN_POINT ( 'NONE',  ( 44.91824650936478491, 31.00000000000000355, 5.910997147197376123 ) ) ;
#32093=CARTESIAN_POINT ( 'NONE',  ( 20.30000058474805869, 40.00000000000000000, -59.80472289869057789 ) ) ;
#32105=CARTESIAN_POINT ( 'NONE',  ( 16.69935377588158332, 40.00000000000000000, -28.93150767131472989 ) ) ;
#32117=CARTESIAN_POINT ( 'NONE',  ( -25.88810397299713628, 31.00000000000000355, 75.89534075019484760 ) ) ;
#32124=CARTESIAN_POINT ( 'NONE',  ( -32.34013556242301490, 40.00000000000000000, 94.87070470178476000 ) ) ;
#32126=CARTESIAN_POINT ( 'NONE',  ( -80.34276469473088866, 40.00000000000000711, 61.48650092628135866 ) ) ;
#32141=CARTESIAN_POINT ( 'NONE',  ( -27.62299686580952240, 40.00000000000000000, -13.61136854378590577 ) ) ;
#32142=CARTESIAN_POINT ( 'NONE',  ( -40.27082278478597033, 40.00000000000000000, 10.71261860272680977 ) ) ;
#32168=CARTESIAN_POINT ( 'NONE',  ( 57.09498703527648900, 31.00000000000000355, 3.831922229400927637 ) ) ;
#32175=CARTESIAN_POINT ( 'NONE',  ( -63.15125318177969405, 40.00000000000000711, -36.59163237596791163 ) ) ;
#32187=CARTESIAN_POINT ( 'NONE',  ( -68.16583574478268304, 31.00000000000000711, -18.25112749842637427 ) ) ;
#32199=CARTESIAN_POINT ( 'NONE',  ( 84.84057271803867195, 31.00000000000000000, 49.13019966417499518 ) ) ;
#32200=CARTESIAN_POINT ( 'NONE',  ( -83.29221842949013421, 40.00000000000000711, -41.19657635676244922 ) ) ;
#32216=CARTESIAN_POINT ( 'NONE',  ( 17.33436897218374639, 31.00000000000000355, 22.64673195036552755 ) ) ;
#32227=CARTESIAN_POINT ( 'NONE',  ( -35.75974951333986240, 40.00000000000000000, 20.56794350806610794 ) ) ;
#32236=CARTESIAN_POINT ( 'NONE',  ( -33.98628324864968420, 31.00000000000000355, 19.63407011443918293 ) ) ;
#32238=SURFACE_SIDE_STYLE ('',( #11990 ) ) ;
#32245=CARTESIAN_POINT ( 'NONE',  ( -89.21153162435624040, 31.00000000000000711, 11.76024306507019901 ) ) ;
#32248=CARTESIAN_POINT ( 'NONE',  ( -52.09564885853935579, 31.00000000000000355, -3.498939618562641574 ) ) ;
#32262=CARTESIAN_POINT ( 'NONE',  ( 72.19657831791809599, 39.99999999999999289, -19.34484491892447622 ) ) ;
#32283=CARTESIAN_POINT ( 'NONE',  ( -15.99999999999997691, 31.00000000000000355, 5.571627607371296764E-15 ) ) ;
#32288=CARTESIAN_POINT ( 'NONE',  ( 28.40420691229738281, 31.00000000000000355, 49.17333623205379922 ) ) ;
#32295=CARTESIAN_POINT ( 'NONE',  ( -16.10381281257427943, 40.00000000000000000, -60.09637020943575436 ) ) ;
#32306=CARTESIAN_POINT ( 'NONE',  ( -20.88694679984194380, 40.00000000000000000, -36.15586224631631751 ) ) ;
#32320=CARTESIAN_POINT ( 'NONE',  ( 78.79907178683629354, 31.00000000000000000, 38.97904116289377185 ) ) ;
#32332=CARTESIAN_POINT ( 'NONE',  ( 1.472621547668719444, 31.00000000000000355, -22.60416666365413718 ) ) ;
#32338=CARTESIAN_POINT ( 'NONE',  ( -26.76192867387533170, 31.00000000000000355, -15.44647709060871321 ) ) ;
#32344=CARTESIAN_POINT ( 'NONE',  ( 24.60508655230852781, 40.00000000000000000, 6.583411914924224284 ) ) ;
#32345=CARTESIAN_POINT ( 'NONE',  ( -39.38196478160931946, 40.00000000000000000, 13.29643045357694753 ) ) ;
#32367=CARTESIAN_POINT ( 'NONE',  ( -23.88228986782336349, 40.00000000000000000, -89.13686966975919290 ) ) ;
#32375=CARTESIAN_POINT ( 'NONE',  ( 33.95200755730775199, 31.00000000000000355, -44.10258293179329314 ) ) ;
#32383=CARTESIAN_POINT ( 'NONE',  ( 69.81317433577432041, 39.99999999999999289, 34.54326205988235188 ) ) ;
#32396=CARTESIAN_POINT ( 'NONE',  ( -31.81163009274181519, 31.00000000000000355, -64.50738158386226928 ) ) ;
#32407=CARTESIAN_POINT ( 'NONE',  ( 12.87762912550514827, 31.00000000000000355, 98.66289914823325091 ) ) ;
#32408=CARTESIAN_POINT ( 'NONE',  ( 94.26586287999622016, 39.99999999999999289, 25.37251369638877563 ) ) ;
#32426=EDGE_CURVE ( 'NONE', #10195, #15282, #12928, .T. ) ;
#32427=CARTESIAN_POINT ( 'NONE',  ( -17.43724119492662794, 31.00000000000000355, -15.29674861594511448 ) ) ;
#32437=CARTESIAN_POINT ( 'NONE',  ( -41.52979953745317232, 40.00000000000000000, 5.398177843167591305 ) ) ;
#32449=CARTESIAN_POINT ( 'NONE',  ( -4.929261580875707871, 31.00000000000000355, 37.46659216873931797 ) ) ;
#32457=CARTESIAN_POINT ( 'NONE',  ( 77.05880969081472642, 31.00000000000000000, 37.98468489477117771 ) ) ;
#32461=CARTESIAN_POINT ( 'NONE',  ( -53.12901929300349479, 31.00000000000000355, 30.56653509229933618 ) ) ;
#32462=CARTESIAN_POINT ( 'NONE',  ( -43.11175393642376719, 40.00000000000000000, 56.02072642018850246 ) ) ;
#32463=CARTESIAN_POINT ( 'NONE',  ( -6.381360069252544953, 40.00000000000000000, 97.60416666604666602 ) ) ;
#32476=CARTESIAN_POINT ( 'NONE',  ( -70.10416666575086708, 40.00000000000000711, -4.581489278090966621 ) ) ;
#32507=CARTESIAN_POINT ( 'NONE',  ( -16.10381281257427943, 31.00000000000000355, -60.09637020943575436 ) ) ;
#32512=CARTESIAN_POINT ( 'NONE',  ( 35.58384423644163519, 31.00000000000000355, 12.14845634898874138 ) ) ;
#32514=CARTESIAN_POINT ( 'NONE',  ( 21.58803501788969115, 40.00000000000000000, 63.55567069162312777 ) ) ;
#32522=CARTESIAN_POINT ( 'NONE',  ( -39.12533628356670334, 40.00000000000000000, -10.47265044290268499 ) ) ;
#32538=CARTESIAN_POINT ( 'NONE',  ( -53.37462671637112521, 31.00000000000000711, 60.68184199296217685 ) ) ;
#32547=CARTESIAN_POINT ( 'NONE',  ( 49.34100556531813453, 40.00000000000000000, 85.68208892729249726 ) ) ;
#32555=CARTESIAN_POINT ( 'NONE',  ( -3.620280825866593055, 31.00000000000000355, 27.53105304817175636 ) ) ;
#32561=CARTESIAN_POINT ( 'NONE',  ( 11.92156526682413720, 40.00000000000000000, 35.08788755311113761 ) ) ;
#32563=CARTESIAN_POINT ( 'NONE',  ( -29.39530816626169596, 40.00000000000000000, -14.54745122861429252 ) ) ;
#32568=VECTOR ( 'NONE', #28273, 1000.000000000000000 ) ;
#32576=CARTESIAN_POINT ( 'NONE',  ( -99.67789407897798526, 31.00000000000000000, -5.066036069491916649 ) ) ;
#32591=LINE ( 'NONE', #25437, #644 ) ;
#32593=CARTESIAN_POINT ( 'NONE',  ( -13.02511903071888355, 31.00000000000000355, 48.29538318457647961 ) ) ;
#32602=CARTESIAN_POINT ( 'NONE',  ( -64.10496366469683949, 40.00000000000000711, 31.48763712508877077 ) ) ;
#32614=CARTESIAN_POINT ( 'NONE',  ( -25.13323546007955045, 31.00000000000000355, 74.03861446737784036 ) ) ;
#32626=CARTESIAN_POINT ( 'NONE',  ( -92.09225407318749035, 31.00000000000000711, -6.144973693751363264 ) ) ;
#32628=CARTESIAN_POINT ( 'NONE',  ( -13.16936484334534008, 40.00000000000000000, 99.04657264458933241 ) ) ;
#32646=CARTESIAN_POINT ( 'NONE',  ( -22.06642698273766356, 31.00000000000000355, -2.901557744773885616 ) ) ;
#32649=DIRECTION ( 'NONE',  ( 0.000000000000000000, 1.000000000000000000, 0.000000000000000000 ) ) ;
#32655=CARTESIAN_POINT ( 'NONE',  ( 31.88898475262399401, 40.00000000000000000, 36.48290236124523744 ) ) ;
#32661=EDGE_LOOP ( 'NONE', ( #10537, #4816, #30011, #38680 ) ) ;
#32667=CARTESIAN_POINT ( 'NONE',  ( 6.197074855318628117, 31.00000000000000355, 46.98549035852928313 ) ) ;
#32671=CARTESIAN_POINT ( 'NONE',  ( 74.49266661913014786, 31.00000000000000000, 43.00976416799198176 ) ) ;
#32675=CARTESIAN_POINT ( 'NONE',  ( -40.14822235767833547, 31.00000000000000355, 45.62378674120104449 ) ) ;
#32677=CARTESIAN_POINT ( 'NONE',  ( 41.67488199336423804, 40.00000000000000000, 54.49293397273886086 ) ) ;
#32683=AXIS2_PLACEMENT_3D ( 'NONE', #1402, #34796, #11254 ) ;
#32691=CARTESIAN_POINT ( 'NONE',  ( 9.510694223897102617, 40.00000000000000000, -72.24097909213479340 ) ) ;
#32717=CARTESIAN_POINT ( 'NONE',  ( 62.51641183113888900, 31.00000000000000000, -16.75201923384928548 ) ) ;
#32722=CARTESIAN_POINT ( 'NONE',  ( -18.66214908251421534, 31.00000000000000355, 24.25811346063288454 ) ) ;
#32725=CARTESIAN_POINT ( 'NONE',  ( 44.85399723358655422, 40.00000000000000000, -58.47732767552992073 ) ) ;
#32731=CARTESIAN_POINT ( 'NONE',  ( 2.781618486875130358, 40.00000000000000000, -42.60416666509636485 ) ) ;
#32745=CARTESIAN_POINT ( 'NONE',  ( 59.96221986557396377, 31.00000000000000355, 78.35452998770438171 ) ) ;
#32752=CARTESIAN_POINT ( 'NONE',  ( -99.67789407897798526, 17.11489954122025736, -5.066036069491909544 ) ) ;
#32761=CARTESIAN_POINT ( 'NONE',  ( 20.70971545910534672, 31.00000000000000355, 15.87948211774388518 ) ) ;
#32773=CARTESIAN_POINT ( 'NONE',  ( -2.781618486875174767, 40.00000000000000000, -42.39583333490362804 ) ) ;
#32774=CARTESIAN_POINT ( 'NONE',  ( -12.95950413119146205, 40.00000000000000000, 37.95406330258916938 ) ) ;
#32801=CARTESIAN_POINT ( 'NONE',  ( -30.89738163651153258, 31.00000000000000355, 40.13100860029957317 ) ) ;
#32809=CARTESIAN_POINT ( 'NONE',  ( 27.50146173784981229, 40.00000000000000000, -80.63904244945182143 ) ) ;
#32818=LINE ( 'NONE', #9482, #39318 ) ;
#32819=CARTESIAN_POINT ( 'NONE',  ( 75.10416666583130052, 31.00000000000000000, 4.908738512847474311 ) ) ;
#32832=CARTESIAN_POINT ( 'NONE',  ( 59.96221986557396377, 31.00000000000000355, 78.35452998770438171 ) ) ;
#32833=CARTESIAN_POINT ( 'NONE',  ( 63.29164158768324455, 39.99999999999999289, -71.97807289018581400 ) ) ;
#32851=DIRECTION ( 'NONE',  ( -0.3806385939525924744, 0.000000000000000000, 0.9247238835424298475 ) ) ;
#32853=CARTESIAN_POINT ( 'NONE',  ( 20.65150112226810819, 31.00000000000000355, -15.81946110361252522 ) ) ;
#32862=CARTESIAN_POINT ( 'NONE',  ( -17.88900094062007184, 40.00000000000000000, 36.12696699726038219 ) ) ;
#32873=CARTESIAN_POINT ( 'NONE',  ( -13.51098712749246467, 31.00000000000000355, -50.41620372279128048 ) ) ;
#32878=CARTESIAN_POINT ( 'NONE',  ( -80.23695839127151430, 31.00000000000000711, 39.56677620416681407 ) ) ;
#32882=CARTESIAN_POINT ( 'NONE',  ( -4.660665814385270167, 31.00000000000000355, 69.59371722956201722 ) ) ;
#32883=CARTESIAN_POINT ( 'NONE',  ( 54.03410584561684971, 40.00000000000000000, 41.58544482236945328 ) ) ;
#32884=CARTESIAN_POINT ( 'NONE',  ( -43.52407497442469264, 40.00000000000000000, 88.29422169633753015 ) ) ;
#32900=CARTESIAN_POINT ( 'NONE',  ( -56.48955861152074220, 40.00000000000000711, -43.32902275383659685 ) ) ;
#32929=CARTESIAN_POINT ( 'NONE',  ( -51.34291522965900612, 31.00000000000000355, 29.65708359768123970 ) ) ;
#32932=CARTESIAN_POINT ( 'NONE',  ( 31.41502175087182991, 31.00000000000000355, -18.07270130326418922 ) ) ;
#32933=CARTESIAN_POINT ( 'NONE',  ( -66.92166868300088822, 40.00000000000000711, -22.71661802240650019 ) ) ;
#32942=ORIENTED_EDGE ( 'NONE', *, *, #30969, .F. ) ;
#32943=CARTESIAN_POINT ( 'NONE',  ( -15.46676570949300000, 40.00000000000000000, 45.57083133015776610 ) ) ;
#32956=CARTESIAN_POINT ( 'NONE',  ( -5.980347265640405752, 31.00000000000000355, 89.59238221257746204 ) ) ;
#32973=CARTESIAN_POINT ( 'NONE',  ( -29.44516979616424024, 31.00000000000000355, -7.879824757621473275 ) ) ;
#32979=CARTESIAN_POINT ( 'NONE',  ( -37.46020281470095625, 40.00000000000000000, 12.72710441276525017 ) ) ;
#32981=CARTESIAN_POINT ( 'NONE',  ( -2.829072032612394594, 40.00000000000000000, -44.39959014221900446 ) ) ;
#33007=CARTESIAN_POINT ( 'NONE',  ( -30.31917247938466176, 31.00000000000000355, 52.30862930534038924 ) ) ;
#33018=CARTESIAN_POINT ( 'NONE',  ( 84.58694138809387653, 39.99999999999999289, 22.77597867319729374 ) ) ;
#33030=CARTESIAN_POINT ( 'NONE',  ( 68.07048008643859305, 31.00000000000000000, 33.55317283102968418 ) ) ;
#33040=CARTESIAN_POINT ( 'NONE',  ( 72.29027477042623673, 31.00000000000000000, -63.25088587033864229 ) ) ;
#33061=CARTESIAN_POINT ( 'NONE',  ( 36.20216622922067273, 31.00000000000000355, 9.761693653842600682 ) ) ;
#33071=CARTESIAN_POINT ( 'NONE',  ( -51.89982240185989326, 40.00000000000000000, 3.308651922604956219 ) ) ;
#33075=VERTEX_POINT ( 'NONE', #3865 ) ;
#33083=CARTESIAN_POINT ( 'NONE',  ( -36.80126402429788612, 31.00000000000000355, 32.28896105221774349 ) ) ;
#33091=CARTESIAN_POINT ( 'NONE',  ( 92.36625196220676060, 31.00000000000000000, 24.73319171124347093 ) ) ;
#33095=CARTESIAN_POINT ( 'NONE',  ( 4.329677741076777053, 31.00000000000000355, -64.59417075179258916 ) ) ;
#33096=CARTESIAN_POINT ( 'NONE',  ( 43.45541166192411708, 40.00000000000000000, -49.38773770141698805 ) ) ;
#33098=CARTESIAN_POINT ( 'NONE',  ( 48.45023387855729879, 40.00000000000000000, 83.88660019351674180 ) ) ;
#33110=CARTESIAN_POINT ( 'NONE',  ( -31.81163009274181519, 40.00000000000000000, -64.50738158386226928 ) ) ;
#33113=VERTEX_POINT ( 'NONE', #30737 ) ;
#33141=CARTESIAN_POINT ( 'NONE',  ( 2.965790448435745574, 31.00000000000000355, -22.56328348808469997 ) ) ;
#33148=CARTESIAN_POINT ( 'NONE',  ( 44.56294422764113250, 31.00000000000000355, 34.17917587534974189 ) ) ;
#33151=CARTESIAN_POINT ( 'NONE',  ( 23.40755275317545880, 31.00000000000000355, 30.61714766194360138 ) ) ;
#33153=CARTESIAN_POINT ( 'NONE',  ( -18.69663849766352826, 40.00000000000000000, -69.77653669617104981 ) ) ;
#33165=CARTESIAN_POINT ( 'NONE',  ( 43.96541952717798551, 40.00000000000000000, 11.76906328551413239 ) ) ;
#33177=CARTESIAN_POINT ( 'NONE',  ( 11.57239447661056353, 31.00000000000000355, 88.72710294830137912 ) ) ;
#33187=AXIS2_PLACEMENT_3D ( 'NONE', #25687, #5783, #38945 ) ;
#33201=CARTESIAN_POINT ( 'NONE',  ( -20.72449291656876369, 31.00000000000000355, -23.61699481730619610 ) ) ;
#33207=CARTESIAN_POINT ( 'NONE',  ( 28.83751338862256119, 40.00000000000000000, -32.88701605462710376 ) ) ;
#33208=CARTESIAN_POINT ( 'NONE',  ( -33.53193138075045709, 40.00000000000000000, 38.09769221459629307 ) ) ;
#33240=CARTESIAN_POINT ( 'NONE',  ( -53.12901929300349479, 31.00000000000000355, 30.56653509229933618 ) ) ;
#33248=CARTESIAN_POINT ( 'NONE',  ( -78.26717753304431824, 40.00000000000000711, -26.69481836930730978 ) ) ;
#33260=CARTESIAN_POINT ( 'NONE',  ( 36.74538074116732389, 31.00000000000000355, -63.64477163140654170 ) ) ;
#33272=CARTESIAN_POINT ( 'NONE',  ( -80.34276469477588023, 31.00000000000000711, 61.48650092630385444 ) ) ;
#33293=CARTESIAN_POINT ( 'NONE',  ( 9.304442065603227618, 31.00000000000000355, 27.50946418541002458 ) ) ;
#33301=CARTESIAN_POINT ( 'NONE',  ( 56.89991739620084843, 40.00000000000000000, -3.630084216720919521 ) ) ;
#33310=CARTESIAN_POINT ( 'NONE',  ( -12.41726970680908515, 31.00000000000000355, 46.38546114896210071 ) ) ;
#33313=ORIENTED_EDGE ( 'NONE', *, *, #2707, .F. ) ;
#33318=CARTESIAN_POINT ( 'NONE',  ( 83.17098260925966713, 31.00000000000000000, 48.02127090943169208 ) ) ;
#33323=AXIS2_PLACEMENT_3D ( 'NONE', #29478, #6332, #29063 ) ;
#33324=CARTESIAN_POINT ( 'NONE',  ( 77.09314031436156256, 31.00000000000000000, 5.156213784760050878 ) ) ;
#33325=CARTESIAN_POINT ( 'NONE',  ( 10.26812810425290579, 40.00000000000000000, 78.79123036454033979 ) ) ;
#33329=EDGE_CURVE ( 'NONE', #26923, #36284, #23094, .T. ) ;
#33341=CARTESIAN_POINT ( 'NONE',  ( 52.74436945453300041, 40.00000000000000000, 68.73989242669851762 ) ) ;
#33353=CARTESIAN_POINT ( 'NONE',  ( 26.89767027507547326, 40.00000000000000000, -1.736414864505229305 ) ) ;
#33359=DIRECTION ( 'NONE',  ( 0.000000000000000000, 1.000000000000000000, 0.000000000000000000 ) ) ;
#33368=CARTESIAN_POINT ( 'NONE',  ( 58.80104710710317306, 31.00000000000000000, -45.11949705600698479 ) ) ;
#33371=CARTESIAN_POINT ( 'NONE',  ( 21.72498709342646706, 31.00000000000000355, -28.22316639787266013 ) ) ;
#33373=CARTESIAN_POINT ( 'NONE',  ( 64.89583333437747115, 39.99999999999999289, -4.254240043327834009 ) ) ;
#33383=CARTESIAN_POINT ( 'NONE',  ( -33.94102792873697183, 40.00000000000000000, -38.68473105385043453 ) ) ;
#33390=ORIENTED_EDGE ( 'NONE', *, *, #9536, .F. ) ;
#33395=CARTESIAN_POINT ( 'NONE',  ( -29.11455967534192979, 31.00000000000000355, 85.38284731564058916 ) ) ;
#33414=CARTESIAN_POINT ( 'NONE',  ( -10.91816144241376563, 31.00000000000000355, -40.73603723627661566 ) ) ;
#33420=CARTESIAN_POINT ( 'NONE',  ( 5.583751958424166162, 40.00000000000000000, -42.43436172917101601 ) ) ;
#33422=CARTESIAN_POINT ( 'NONE',  ( -46.12092335263332643, 40.00000000000000000, 22.64177125690310177 ) ) ;
#33447=CARTESIAN_POINT ( 'NONE',  ( 60.82800096162477388, 31.00000000000000000, 30.10617641798563682 ) ) ;
#33453=CARTESIAN_POINT ( 'NONE',  ( 83.84057477258951963, 39.99999999999999289, -22.33845567676512900 ) ) ;
#33467=CARTESIAN_POINT ( 'NONE',  ( -21.28946418274055929, 31.00000000000000355, -79.45670318283352174 ) ) ;
#33483=AXIS2_PLACEMENT_3D ( 'NONE', #15883, #19585, #19163 ) ;
#33498=CARTESIAN_POINT ( 'NONE',  ( -26.24023198663968515, 31.00000000000000355, -20.19409642360271917 ) ) ;
#33505=CARTESIAN_POINT ( 'NONE',  ( 15.70068437845367093, 40.00000000000000000, 46.50252577712053892 ) ) ;
#33520=CARTESIAN_POINT ( 'NONE',  ( 11.12085686420672381, 31.00000000000000355, -41.54537790535560760 ) ) ;
#33526=CARTESIAN_POINT ( 'NONE',  ( -49.27414759474276451, 31.00000000000000711, 85.34056160678568403 ) ) ;
#33530=CARTESIAN_POINT ( 'NONE',  ( -10.54315780145427617, 31.00000000000000355, 79.17709703063970039 ) ) ;
#33531=CARTESIAN_POINT ( 'NONE',  ( -53.37462671635322664, 40.00000000000000711, 60.68184199298008252 ) ) ;
#33545=CARTESIAN_POINT ( 'NONE',  ( -70.72766149062127283, 40.00000000000000711, 54.26934393422349956 ) ) ;
#33557=VERTEX_POINT ( 'NONE', #23728 ) ;
#33558=CARTESIAN_POINT ( 'NONE',  ( 24.14050371820133023, 40.00000000000000000, 13.97356841391088444 ) ) ;
#33576=CARTESIAN_POINT ( 'NONE',  ( 8.815036365794538753, 31.00000000000000355, 66.85656860134390911 ) ) ;
#33580=CARTESIAN_POINT ( 'NONE',  ( -41.52979953746218911, 31.00000000000000355, 5.398177843165337109 ) ) ;
#33582=CARTESIAN_POINT ( 'NONE',  ( -80.10416666582359824, 40.00000000000000711, -5.235987747607834031 ) ) ;
#33592=CARTESIAN_POINT ( 'NONE',  ( -44.33513214241411760, 40.00000000000000000, 38.89722855811361768 ) ) ;
#33605=CARTESIAN_POINT ( 'NONE',  ( -88.68107738130200346, 31.00000000000000711, 23.63280646692842524 ) ) ;
#33621=CARTESIAN_POINT ( 'NONE',  ( 11.92156526682413720, 31.00000000000000355, 35.08788755311113761 ) ) ;
#33629=CARTESIAN_POINT ( 'NONE',  ( -3.436116956419240864, 40.00000000000000000, -52.39583333462812931 ) ) ;
#33630=CARTESIAN_POINT ( 'NONE',  ( -26.44890248586417414, 40.00000000000000000, -34.59877114778964113 ) ) ;
#33633=DIRECTION ( 'NONE',  ( 0.000000000000000000, -7.709882115452474222E-16, -1.000000000000000000 ) ) ;
#33639=CARTESIAN_POINT ( 'NONE',  ( -1.799870782497340782, 40.00000000000000000, 27.60416666422008802 ) ) ;
#33655=CARTESIAN_POINT ( 'NONE',  ( -56.33579487689731735, 31.00000000000000355, -27.88694065509425002 ) ) ;
#33663=CARTESIAN_POINT ( 'NONE',  ( -71.82650799747224823, 40.00000000000000711, -41.60779115366585756 ) ) ;
#33669=MECHANICAL_DESIGN_GEOMETRIC_PRESENTATION_REPRESENTATION('',(#26029),#19759);
#33677=CARTESIAN_POINT ( 'NONE',  ( -84.90650804512098659, 31.00000000000000711, 28.83788733109305014 ) ) ;
#33706=CARTESIAN_POINT ( 'NONE',  ( 25.29542371717656835, 31.00000000000000355, 28.93716311998947788 ) ) ;
#33714=CARTESIAN_POINT ( 'NONE',  ( 24.55685208795062380, 40.00000000000000000, -49.59815698162134368 ) ) ;
#33727=CARTESIAN_POINT ( 'NONE',  ( -59.89583333444493718, 31.00000000000000711, 3.926990808566372060 ) ) ;
#33734=CARTESIAN_POINT ( 'NONE',  ( 20.96880926229634312, 40.00000000000000000, -12.11681000168150213 ) ) ;
#33739=CARTESIAN_POINT ( 'NONE',  ( -71.33925323112771366, 31.00000000000000711, 9.290813765106920030 ) ) ;
#33740=CARTESIAN_POINT ( 'NONE',  ( 69.81317433577432041, 39.99999999999999289, 34.54326205988235188 ) ) ;
#33748=ADVANCED_FACE ( 'NONE', ( #1417 ), #41331, .T. ) ;
#33759=CARTESIAN_POINT ( 'NONE',  ( -54.00384411202717416, 40.00000000000000711, 70.40394205935166383 ) ) ;
#33770=CARTESIAN_POINT ( 'NONE',  ( 21.18498618631003438, 40.00000000000000000, 18.62224443192851098 ) ) ;
#33783=VECTOR ( 'NONE', #20353, 1000.000000000000114 ) ;
#33791=CARTESIAN_POINT ( 'NONE',  ( -4.745113895469965648, 31.00000000000000355, -72.39583333427917466 ) ) ;
#33793=CARTESIAN_POINT ( 'NONE',  ( 6.367266499441480043, 31.00000000000000355, 48.98256792610027333 ) ) ;
#33794=CARTESIAN_POINT ( 'NONE',  ( 60.46509673945340779, 39.99999999999999289, 46.37897171328766888 ) ) ;
#33809=CARTESIAN_POINT ( 'NONE',  ( -7.547223091130065953, 40.00000000000000000, 57.33767041057931380 ) ) ;
#33841=CARTESIAN_POINT ( 'NONE',  ( -18.51709390187839688, 31.00000000000000355, -37.54239277154294996 ) ) ;
#33844=LINE ( 'NONE', #27532, #20537 ) ;
#33851=CARTESIAN_POINT ( 'NONE',  ( -6.238242335983215092, 40.00000000000000000, 47.40213128959678102 ) ) ;
#33852=CARTESIAN_POINT ( 'NONE',  ( 36.58905133581346547, 40.00000000000000000, -27.97030060560320308 ) ) ;
#33853=VECTOR ( 'NONE', #7360, 1000.000000000000114 ) ;
#33863=CARTESIAN_POINT ( 'NONE',  ( -7.231618336280544845, 40.00000000000000000, 27.02512817425793656 ) ) ;
#33883=CARTESIAN_POINT ( 'NONE',  ( -58.00742674159663892, 31.00000000000000711, -44.63796826975934096 ) ) ;
#33889=VECTOR ( 'NONE', #4745, 1000.000000000000000 ) ;
#33891=CARTESIAN_POINT ( 'NONE',  ( 83.51212062389942048, 39.99999999999999289, -48.08891344038907079 ) ) ;
#33893=CARTESIAN_POINT ( 'NONE',  ( -105.9879088449591933, 31.00000000000000355, -0.3807199291576673361 ) ) ;
#33902=CARTESIAN_POINT ( 'NONE',  ( 80.16187752211510542, 31.00000000000000000, -27.22680903928618434 ) ) ;
#33912=CARTESIAN_POINT ( 'NONE',  ( -98.36195137685432144, 31.00000000000000711, 26.22212808231157055 ) ) ;
#33914=EDGE_CURVE ( 'NONE', #29860, #41658, #36498, .T. ) ;
#33928=DIRECTION ( 'NONE',  ( 0.000000000000000000, -7.709882115452471264E-16, -1.000000000000000000 ) ) ;
#33934=CARTESIAN_POINT ( 'NONE',  ( -30.58448433907586761, 31.00000000000000355, 8.146263651248247584 ) ) ;
#33941=CARTESIAN_POINT ( 'NONE',  ( -51.46673615999394968, 40.00000000000000000, 6.691140578787329041 ) ) ;
#33950=ORIENTED_EDGE ( 'NONE', *, *, #31879, .T. ) ;
#33955=CARTESIAN_POINT ( 'NONE',  ( 13.71368254939966036, 31.00000000000000355, -51.22554439249349656 ) ) ;
#33961=CARTESIAN_POINT ( 'NONE',  ( -96.39699453480135105, 31.00000000000000711, 25.82690913164849889 ) ) ;
#33965=CARTESIAN_POINT ( 'NONE',  ( -56.48168293059611500, 31.00000000000000711, 43.19841958068096233 ) ) ;
#33966=CARTESIAN_POINT ( 'NONE',  ( 50.06853320189533463, 39.99999999999999289, -56.91684085114077618 ) ) ;
#33982=CARTESIAN_POINT ( 'NONE',  ( -86.71682804797315214, 40.00000000000000711, 23.23408344657299196 ) ) ;
#33984=APPLICATION_CONTEXT ( 'automotive_design' ) ;
#33995=CARTESIAN_POINT ( 'NONE',  ( -21.37212791037562098, 40.00000000000000000, -7.253704819186252983 ) ) ;
#33998=DIRECTION ( 'NONE',  ( -0.9979848074931935153, 0.000000000000000000, -0.06345332152672163162 ) ) ;
#34009=CARTESIAN_POINT ( 'NONE',  ( 20.96880926229634312, 31.00000000000000355, -12.11681000168150213 ) ) ;
#34016=CARTESIAN_POINT ( 'NONE',  ( -17.60292107714122878, 31.00000000000000355, 65.74579412301164894 ) ) ;
#34018=CARTESIAN_POINT ( 'NONE',  ( -37.13421060599358725, 31.00000000000000355, -21.52932707635455500 ) ) ;
#34019=CARTESIAN_POINT ( 'NONE',  ( 57.37208743749949491, 40.00000000000000000, 50.31438278193533620 ) ) ;
#34032=ORIENTED_EDGE ( 'NONE', *, *, #42224, .F. ) ;
#34033=CARTESIAN_POINT ( 'NONE',  ( 42.30435120181500963, 40.00000000000000000, 37.09784777058769123 ) ) ;
#34047=CARTESIAN_POINT ( 'NONE',  ( -61.42214656768812375, 31.00000000000000711, 79.86467493626638259 ) ) ;
#34066=CARTESIAN_POINT ( 'NONE',  ( 28.83751338862256119, 31.00000000000000355, -32.88701605462710376 ) ) ;
#34073=CARTESIAN_POINT ( 'NONE',  ( -38.53741714288415210, 40.00000000000000000, -33.79371401777069650 ) ) ;
#34074=CARTESIAN_POINT ( 'NONE',  ( 36.84045577241590763, 40.00000000000000000, -41.86038302679909151 ) ) ;
#34080=CARTESIAN_POINT ( 'NONE',  ( 20.96880926229634312, 40.00000000000000000, -12.11681000168150213 ) ) ;
#34098=CARTESIAN_POINT ( 'NONE',  ( 69.81317433577432041, 31.00000000000000000, 34.54326205989952570 ) ) ;
#34104=CARTESIAN_POINT ( 'NONE',  ( 42.30527206516848793, 40.00000000000000000, -85.53883208674149330 ) ) ;
#34117=CARTESIAN_POINT ( 'NONE',  ( 81.87674480462379734, 31.00000000000000000, -21.93767060400471891 ) ) ;
#34121=CARTESIAN_POINT ( 'NONE',  ( -22.06642698273767067, 40.00000000000000000, -2.901557744773887393 ) ) ;
#34145=CARTESIAN_POINT ( 'NONE',  ( -24.78443185005114557, 31.00000000000000355, 32.19086620116432584 ) ) ;
#34150=CARTESIAN_POINT ( 'NONE',  ( 32.82854187708761629, 40.00000000000000000, -56.64543409044760125 ) ) ;
#34160=CARTESIAN_POINT ( 'NONE',  ( 14.80739997004469366, 31.00000000000000355, 55.25628696611591550 ) ) ;
#34161=DIRECTION ( 'NONE',  ( -0.3806385939525924744, 0.000000000000000000, 0.9247238835424298475 ) ) ;
#34162=EDGE_LOOP ( 'NONE', ( #37823, #41311, #37191, #42514 ) ) ;
#34168=CARTESIAN_POINT ( 'NONE',  ( -19.19493090124598922, 40.00000000000000000, -25.00897302100653263 ) ) ;
#34176=CARTESIAN_POINT ( 'NONE',  ( -43.11175393642376008, 31.00000000000000355, 56.02072642018850246 ) ) ;
#34177=CARTESIAN_POINT ( 'NONE',  ( 24.27443280711675655, 40.00000000000000000, -71.15176282235543681 ) ) ;
#34190=CARTESIAN_POINT ( 'NONE',  ( 28.03234818517180216, 40.00000000000000000, 82.53419278363811884 ) ) ;
#34192=EDGE_CURVE ( 'NONE', #27469, #33113, #42881, .T. ) ;
#34204=CARTESIAN_POINT ( 'NONE',  ( 25.29542371717657545, 40.00000000000000000, 28.93716311999360613 ) ) ;
#34217=CARTESIAN_POINT ( 'NONE',  ( 15.62097837807030842, 31.00000000000000355, -17.81927981957692353 ) ) ;
#34225=CARTESIAN_POINT ( 'NONE',  ( -67.35649507452052376, 31.00000000000000711, 18.04843207638801772 ) ) ;
#34227=CARTESIAN_POINT ( 'NONE',  ( -14.09736097164098823, 31.00000000000000355, -41.75563764759219509 ) ) ;
#34229=CARTESIAN_POINT ( 'NONE',  ( -77.03666156126601550, 40.00000000000000711, 20.64125776147949409 ) ) ;
#34240=CARTESIAN_POINT ( 'NONE',  ( 52.83624534446448706, 40.00000000000000000, -14.15919354876300318 ) ) ;
#34249=ORIENTED_EDGE ( 'NONE', *, *, #23817, .F. ) ;
#34255=CARTESIAN_POINT ( 'NONE',  ( -87.85203729257557370, 31.00000000000000711, 50.59313708110082786 ) ) ;
#34272=CARTESIAN_POINT ( 'NONE',  ( -16.93500259178182432, 31.00000000000000355, 34.36424406943201149 ) ) ;
#34281=CARTESIAN_POINT ( 'NONE',  ( 32.65420139560029611, 40.00000000000000000, -42.57517516360295673 ) ) ;
#34282=CARTESIAN_POINT ( 'NONE',  ( 14.32751628686350287, 40.00000000000000000, -53.13354968558886071 ) ) ;
#34289=CARTESIAN_POINT ( 'NONE',  ( 11.68784703496123711, 40.00000000000000000, -20.25319168173327355 ) ) ;
#34308=CARTESIAN_POINT ( 'NONE',  ( -71.90006454728114704, 31.00000000000000711, 4.599370544632132685 ) ) ;
#34315=CARTESIAN_POINT ( 'NONE',  ( -12.22491041697691294, 40.00000000000000000, -93.69500887688228374 ) ) ;
#34326=CARTESIAN_POINT ( 'NONE',  ( 64.90595555533579386, 31.00000000000000000, 56.92265028768127166 ) ) ;
#34330=AXIS2_PLACEMENT_3D ( 'NONE', #591, #23555, #37249 ) ;
#34331=CARTESIAN_POINT ( 'NONE',  ( -17.43724119492421565, 40.00000000000000000, -15.29674861594511803 ) ) ;
#34359=CARTESIAN_POINT ( 'NONE',  ( -39.38196478161825809, 31.00000000000000355, 13.29643045357694398 ) ) ;
#34365=CARTESIAN_POINT ( 'NONE',  ( -40.14822235766499148, 40.00000000000000000, 45.62378674120105160 ) ) ;
#34375=CARTESIAN_POINT ( 'NONE',  ( 7.506055610550203205, 31.00000000000000355, 56.92102948000351148 ) ) ;
#34378=EDGE_CURVE ( 'NONE', #10114, #26923, #42656, .T. ) ;
#34380=CARTESIAN_POINT ( 'NONE',  ( 16.69935377588158332, 40.00000000000000000, -28.93150767131472989 ) ) ;
#34384=CARTESIAN_POINT ( 'NONE',  ( -23.42519174998115616, 31.00000000000000355, 87.00664592748896098 ) ) ;
#34385=CARTESIAN_POINT ( 'NONE',  ( -88.68107738130200346, 40.00000000000000711, 23.63280646693861087 ) ) ;
#34400=CARTESIAN_POINT ( 'NONE',  ( -78.67873774631718220, 40.00000000000000711, 60.36924185307643143 ) ) ;
#34412=ORIENTED_EDGE ( 'NONE', *, *, #28095, .F. ) ;
#34414=CARTESIAN_POINT ( 'NONE',  ( -31.99444157863030114, 40.00000000000000000, -4.262017635501984536 ) ) ;
#34426=CARTESIAN_POINT ( 'NONE',  ( -9.022452542771789652, 31.00000000000000355, 26.59230923919664491 ) ) ;
#34434=CARTESIAN_POINT ( 'NONE',  ( 38.42722039544141666, 31.00000000000000355, 66.52996821281629991 ) ) ;
#34437=CARTESIAN_POINT ( 'NONE',  ( -28.59133019391535768, 31.00000000000000355, -32.71076623427349261 ) ) ;
#34439=CARTESIAN_POINT ( 'NONE',  ( 77.05880969081472642, 39.99999999999999289, 37.98468489477117771 ) ) ;
#34451=CARTESIAN_POINT ( 'NONE',  ( 63.32575250126041055, 39.99999999999999289, 16.95471465585521997 ) ) ;
#34481=CARTESIAN_POINT ( 'NONE',  ( 3.436116956419347002, 31.00000000000000355, -52.60416666537189911 ) ) ;
#34491=CARTESIAN_POINT ( 'NONE',  ( 28.34477777927418529, 40.00000000000000000, 36.93558740410973229 ) ) ;
#34493=CARTESIAN_POINT ( 'NONE',  ( -3.998040010416403334, 40.00000000000000000, 59.59469406578620720 ) ) ;
#34499=CARTESIAN_POINT ( 'NONE',  ( -18.08361268445098347, 31.00000000000000355, -10.43497034982449456 ) ) ;
#34502=CARTESIAN_POINT ( 'NONE',  ( -2.924622967158192921, 40.00000000000000000, -22.14664255385889291 ) ) ;
#34511=EDGE_LOOP ( 'NONE', ( #12044, #9142, #17201, #25573 ) ) ;
#34516=CARTESIAN_POINT ( 'NONE',  ( 60.45897909542819804, 31.00000000000000000, -46.24578392211154210 ) ) ;
#34527=CARTESIAN_POINT ( 'NONE',  ( 84.84057271799511568, 39.99999999999999289, 49.13019966419678752 ) ) ;
#34541=CARTESIAN_POINT ( 'NONE',  ( 74.49266661913014786, 31.00000000000000000, 43.00976416799198176 ) ) ;
#34546=CARTESIAN_POINT ( 'NONE',  ( -31.89861325429239258, 40.00000000000000000, 2.042328591206914012 ) ) ;
#34553=CARTESIAN_POINT ( 'NONE',  ( -22.00000000000000000, 40.00000000000000000, 0.000000000000000000 ) ) ;
#34576=CARTESIAN_POINT ( 'NONE',  ( -20.27214883179046367, 31.00000000000000355, 34.96734655410254788 ) ) ;
#34582=CARTESIAN_POINT ( 'NONE',  ( 66.75914267698914273, 39.99999999999999289, 8.899205196614580871 ) ) ;
#34590=CIRCLE ( 'NONE', #15143, 4.500000000000000888 ) ;
#34594=CARTESIAN_POINT ( 'NONE',  ( 55.10416666547021691, 31.00000000000000355, 3.599741573803287853 ) ) ;
#34597=ORIENTED_EDGE ( 'NONE', *, *, #30321, .F. ) ;
#34601=CARTESIAN_POINT ( 'NONE',  ( 22.22924588317381023, 40.00000000000000000, -25.35314793696836588 ) ) ;
#34606=CARTESIAN_POINT ( 'NONE',  ( -81.90010630563853056, 31.00000000000000711, 5.248159452637419342 ) ) ;
#34607=CARTESIAN_POINT ( 'NONE',  ( 86.24314314301659579, 39.99999999999999289, -11.24622374122959201 ) ) ;
#34622=CARTESIAN_POINT ( 'NONE',  ( -99.14707074559267141, 40.00000000000000711, 13.06922382031732610 ) ) ;
#34627=CARTESIAN_POINT ( 'NONE',  ( -20.64238946400878305, 17.11489954122026447, 3.177240882809045708 ) ) ;
#34638=CARTESIAN_POINT ( 'NONE',  ( -14.91913624998189825, 40.00000000000000000, -30.37684071747814230 ) ) ;
#34650=CARTESIAN_POINT ( 'NONE',  ( 8.699408683037360035, 31.00000000000000355, 25.59862650653646909 ) ) ;
#34660=CARTESIAN_POINT ( 'NONE',  ( 10.81967497908702214, 31.00000000000000355, -82.17651821321413763 ) ) ;
#34665=CARTESIAN_POINT ( 'NONE',  ( 3.665567271000699012, 31.00000000000000355, -54.59530427605618996 ) ) ;
#34666=CARTESIAN_POINT ( 'NONE',  ( 64.90595555531619709, 39.99999999999999289, 56.92265028770086843 ) ) ;
#34678=CARTESIAN_POINT ( 'NONE',  ( 21.58803501788969115, 40.00000000000000000, 63.55567069162312777 ) ) ;
#34686=ORIENTED_EDGE ( 'NONE', *, *, #22006, .T. ) ;
#34693=CARTESIAN_POINT ( 'NONE',  ( -66.59699903142619348, 31.00000000000000711, 75.74378954611491110 ) ) ;
#34708=CARTESIAN_POINT ( 'NONE',  ( -16.75480014238754478, 31.00000000000000355, -49.32177912249007790 ) ) ;
#34711=CARTESIAN_POINT ( 'NONE',  ( -20.39032260654148487, 31.00000000000000355, 1.150830359615497178 ) ) ;
#34718=CARTESIAN_POINT ( 'NONE',  ( 52.83624534446448706, 40.00000000000000000, -14.15919354876300318 ) ) ;
#34720=CARTESIAN_POINT ( 'NONE',  ( 57.09498703527649610, 40.00000000000000000, 3.831922229401318880 ) ) ;
#34730=CARTESIAN_POINT ( 'NONE',  ( -9.654069774896838041, 31.00000000000000355, -19.56573356436190636 ) ) ;
#34732=CARTESIAN_POINT ( 'NONE',  ( -8.325335757348113930, 40.00000000000000000, -31.05587074991522201 ) ) ;
#34746=CARTESIAN_POINT ( 'NONE',  ( -53.44803860757283331, 31.00000000000000355, 46.73995993579659114 ) ) ;
#34756=CARTESIAN_POINT ( 'NONE',  ( 73.86091552542920624, 39.99999999999999289, 64.94433634442138725 ) ) ;
#34757=CARTESIAN_POINT ( 'NONE',  ( 21.18498618631003083, 31.00000000000000355, 18.62224443192850387 ) ) ;
#34768=CARTESIAN_POINT ( 'NONE',  ( 83.17098260925966713, 31.00000000000000000, 48.02127090943169208 ) ) ;
#34771=CARTESIAN_POINT ( 'NONE',  ( 25.73918080462997082, 40.00000000000000000, -6.871072672212912735 ) ) ;
#34796=DIRECTION ( 'NONE',  ( 0.000000000000000000, 1.000000000000000000, 0.000000000000000000 ) ) ;
#34798=CARTESIAN_POINT ( 'NONE',  ( -41.89947471387618805, 31.00000000000000355, 2.670153906482984674 ) ) ;
#34799=EDGE_CURVE ( 'NONE', #41039, #6230, #18305, .T. ) ;
#34805=CARTESIAN_POINT ( 'NONE',  ( -61.40313508883502891, 40.00000000000000711, 7.989450542818913092 ) ) ;
#34818=CARTESIAN_POINT ( 'NONE',  ( 4.745113895470035814, 31.00000000000000355, -72.60416666572081112 ) ) ;
#34826=CARTESIAN_POINT ( 'NONE',  ( 11.57239447661056353, 31.00000000000000355, 88.72710294830137912 ) ) ;
#34827=CARTESIAN_POINT ( 'NONE',  ( 64.75392801420538547, 39.99999999999999289, -56.64582372546511380 ) ) ;
#34840=CARTESIAN_POINT ( 'NONE',  ( -74.47060461443528823, 40.00000000000000711, 65.33029858165178894 ) ) ;
#34856=CARTESIAN_POINT ( 'NONE',  ( 35.42814233786123879, 40.00000000000000000, -9.427541829740359702 ) ) ;
#34868=CARTESIAN_POINT ( 'NONE',  ( -25.29482881991252086, 31.00000000000000355, -32.96004927633274662 ) ) ;
#34874=CARTESIAN_POINT ( 'NONE',  ( 34.02738612458995959, 31.00000000000000355, 69.00154638599002510 ) ) ;
#34876=CARTESIAN_POINT ( 'NONE',  ( 50.61746024623598572, 31.00000000000000355, -24.85206051842254737 ) ) ;
#34878=CARTESIAN_POINT ( 'NONE',  ( -66.93673649651354651, 40.00000000000000711, 58.72203107584222437 ) ) ;
#34890=CARTESIAN_POINT ( 'NONE',  ( 64.78932475141161262, 39.99999999999999289, 8.528958657501300777 ) ) ;
#34922=CARTESIAN_POINT ( 'NONE',  ( 40.56819808336118882, 31.00000000000000355, -35.59309480518532354 ) ) ;
#34931=CARTESIAN_POINT ( 'NONE',  ( 34.44467569804516671, 40.00000000000000000, 44.88666365967159777 ) ) ;
#34932=CARTESIAN_POINT ( 'NONE',  ( 43.74200748489512591, 40.00000000000000000, 38.49442098324160355 ) ) ;
#34937=CARTESIAN_POINT ( 'NONE',  ( 21.81281596512078025, 31.00000000000000355, -10.76194779073239083 ) ) ;
#34939=CARTESIAN_POINT ( 'NONE',  ( -28.96462450050677973, 40.00000000000000000, -9.827991688575851370 ) ) ;
#34947=ORIENTED_EDGE ( 'NONE', *, *, #34192, .F. ) ;
#34954=CARTESIAN_POINT ( 'NONE',  ( 44.33290732825512492, 31.00000000000000355, 77.00207852755224280 ) ) ;
#34959=ORIENTED_EDGE ( 'NONE', *, *, #34799, .F. ) ;
#34965=CARTESIAN_POINT ( 'NONE',  ( -22.10416666678001008, 31.00000000000000355, -1.441157586896874898 ) ) ;
#34976=CARTESIAN_POINT ( 'NONE',  ( -99.89583333318432778, 31.00000000000000711, 6.544984695199788760 ) ) ;
#34979=CARTESIAN_POINT ( 'NONE',  ( 26.89767027507547326, 40.00000000000000000, -1.736414864505229305 ) ) ;
#35007=CARTESIAN_POINT ( 'NONE',  ( 44.12914893500597202, 31.00000000000000355, -14.89880614700436112 ) ) ;
#35016=CARTESIAN_POINT ( 'NONE',  ( -15.62887661519555493, 40.00000000000000000, 57.97203279869352599 ) ) ;
#35028=CARTESIAN_POINT ( 'NONE',  ( -18.69663849766352826, 31.00000000000000355, -69.77653669617104981 ) ) ;
#35036=CARTESIAN_POINT ( 'NONE',  ( -21.69137426901471954, 31.00000000000000355, -81.42030341110597647 ) ) ;
#35037=CARTESIAN_POINT ( 'NONE',  ( -55.31949386280459180, 40.00000000000000711, 71.91600076662652441 ) ) ;
#35053=LINE ( 'NONE', #34627, #33889 ) ;
#35062=CARTESIAN_POINT ( 'NONE',  ( 36.89914868738106435, 40.00000000000000000, -2.354335741662294978 ) ) ;
#35069=VERTEX_POINT ( 'NONE', #16078 ) ;
#35075=CARTESIAN_POINT ( 'NONE',  ( -2.454369252093152376, 31.00000000000000355, 37.60416666486730009 ) ) ;
#35080=CARTESIAN_POINT ( 'NONE',  ( -34.66105084696506822, 31.00000000000000355, 70.31756248751102589 ) ) ;
#35085=CARTESIAN_POINT ( 'NONE',  ( -51.46673616000524021, 31.00000000000000355, 6.691140578787329041 ) ) ;
#35088=CARTESIAN_POINT ( 'NONE',  ( -22.78857244739539212, 40.00000000000000000, 85.10612709700112077 ) ) ;
#35100=CARTESIAN_POINT ( 'NONE',  ( -41.80404827410195168, 40.00000000000000000, 54.50178954758867889 ) ) ;
#35127=DIRECTION ( 'NONE',  ( 0.9470131699890049770, 1.701542661702850483E-16, 0.3211947320043963550 ) ) ;
#35129=CARTESIAN_POINT ( 'NONE',  ( -3.436116956419240864, 31.00000000000000355, -52.39583333462812931 ) ) ;
#35138=CARTESIAN_POINT ( 'NONE',  ( 54.85378563033546584, 40.00000000000000000, 7.219977902337870290 ) ) ;
#35145=CARTESIAN_POINT ( 'NONE',  ( -18.63466726053507472, 31.00000000000000355, -9.179856479542758407 ) ) ;
#35148=CARTESIAN_POINT ( 'NONE',  ( 2.127120017302678523, 40.00000000000000000, -32.60416666460785962 ) ) ;
#35160=DIRECTION ( 'NONE',  ( -0.9470131699890049770, 0.000000000000000000, -0.3211947320043963550 ) ) ;
#35161=CARTESIAN_POINT ( 'NONE',  ( -78.26717753304431824, 31.00000000000000711, -26.69481836928899554 ) ) ;
#35168=CARTESIAN_POINT ( 'NONE',  ( 16.96065435355024320, 31.00000000000000355, -19.31014141889295388 ) ) ;
#35170=DIRECTION ( 'NONE',  ( 0.000000000000000000, 0.000000000000000000, -1.000000000000000000 ) ) ;
#35181=CARTESIAN_POINT ( 'NONE',  ( -25.38139813252123034, 31.00000000000000355, 94.78629358389331117 ) ) ;
#35188=CARTESIAN_POINT ( 'NONE',  ( 11.33656872182470643, 40.00000000000000000, -33.21392199183605953 ) ) ;
#35217=CARTESIAN_POINT ( 'NONE',  ( 3.148395399070833989, 31.00000000000000355, 49.39975974383467872 ) ) ;
#35220=CARTESIAN_POINT ( 'NONE',  ( -19.99999999999999645, 31.00000000000000355, 2.168407390121265812E-15 ) ) ;
#35225=CARTESIAN_POINT ( 'NONE',  ( -72.09351246578157202, 40.00000000000000711, -4.825959690424619808 ) ) ;
#35229=CARTESIAN_POINT ( 'NONE',  ( -105.9879088449591933, 40.00000000000000000, -0.3807199291576673361 ) ) ;
#35233=CARTESIAN_POINT ( 'NONE',  ( 65.10416666562252885, 31.00000000000000000, 4.254240043327690124 ) ) ;
#35245=CARTESIAN_POINT ( 'NONE',  ( 76.16439905407254685, 31.00000000000000000, 44.11546174421767574 ) ) ;
#35247=CARTESIAN_POINT ( 'NONE',  ( 84.58694138809387653, 39.99999999999999289, 22.77597867319729374 ) ) ;
#35248=EDGE_CURVE ( 'NONE', #15357, #19261, #28395, .T. ) ;
#35266=CARTESIAN_POINT ( 'NONE',  ( 25.13348990051749254, 31.00000000000000355, -8.510361017572021680 ) ) ;
#35279=CARTESIAN_POINT ( 'NONE',  ( -5.264430561742839743, 40.00000000000000000, 39.44269128746232411 ) ) ;
#35292=CARTESIAN_POINT ( 'NONE',  ( 16.69935377588158332, 31.00000000000000355, -28.93150767131472989 ) ) ;
#35299=CARTESIAN_POINT ( 'NONE',  ( 36.87680687886029318, 31.00000000000000355, -74.81172728975037955 ) ) ;
#35302=CARTESIAN_POINT ( 'NONE',  ( 7.251580242022521716, 31.00000000000000355, -54.34182998361462325 ) ) ;
#35303=CARTESIAN_POINT ( 'NONE',  ( 41.30831894254264824, 40.00000000000000000, -83.80005689411834169 ) ) ;
#35314=CARTESIAN_POINT ( 'NONE',  ( -19.99999999999999645, 40.00000000000000000, 1.283214542831033755 ) ) ;
#35320=CARTESIAN_POINT ( 'NONE',  ( 50.84997085138504502, 39.99999999999999289, -39.01959913716785167 ) ) ;
#35321=CARTESIAN_POINT ( 'NONE',  ( -22.00000000000000000, 31.00000000000000355, 0.000000000000000000 ) ) ;
#35346=AXIS2_PLACEMENT_3D ( 'NONE', #21095, #733, #14097 ) ;
#35352=CARTESIAN_POINT ( 'NONE',  ( -24.21661388771557100, 31.00000000000000355, 41.94898165618241137 ) ) ;
#35357=CARTESIAN_POINT ( 'NONE',  ( -30.90996028308246224, 40.00000000000000000, -53.51249422725337013 ) ) ;
#35368=CARTESIAN_POINT ( 'NONE',  ( -35.29531037056285214, 40.00000000000000000, 17.40921588598563119 ) ) ;
#35384=CARTESIAN_POINT ( 'NONE',  ( 86.90011881125596460, 31.00000000000000000, -5.573058087428397478 ) ) ;
#35394=CARTESIAN_POINT ( 'NONE',  ( -98.36195137680903144, 40.00000000000000711, 26.22212808230024805 ) ) ;
#35406=CARTESIAN_POINT ( 'NONE',  ( 6.381360069253262601, 31.00000000000000355, 97.39583333395333398 ) ) ;
#35410=CARTESIAN_POINT ( 'NONE',  ( 7.028922914820973311, 40.00000000000000000, 26.21578750688660264 ) ) ;
#35411=CARTESIAN_POINT ( 'NONE',  ( 2.511863649308039736, 40.00000000000000000, 39.39933062585536305 ) ) ;
#35423=DIRECTION ( 'NONE',  ( 0.000000000000000000, 1.000000000000000000, -1.060184893785364939E-15 ) ) ;
#35434=DIRECTION ( 'NONE',  ( 0.000000000000000000, 1.000000000000000000, 0.000000000000000000 ) ) ;
#35436=CARTESIAN_POINT ( 'NONE',  ( -50.71442127988192539, 31.00000000000000355, -13.67646662467867991 ) ) ;
#35444=CARTESIAN_POINT ( 'NONE',  ( 77.09314031436157677, 39.99999999999999289, 5.156213784760051766 ) ) ;
#35454=CARTESIAN_POINT ( 'NONE',  ( -70.10416666575086708, 31.00000000000000711, -4.581489278090966621 ) ) ;
#35464=CARTESIAN_POINT ( 'NONE',  ( -91.90012763196533285, 31.00000000000000711, 5.898218105444796855 ) ) ;
#35465=CARTESIAN_POINT ( 'NONE',  ( 72.29027477046881245, 39.99999999999999289, -63.25088587038124643 ) ) ;
#35473=ORIENTED_EDGE ( 'NONE', *, *, #36834, .F. ) ;
#35478=CARTESIAN_POINT ( 'NONE',  ( 21.18498618631003083, 31.00000000000000355, 18.62224443192850387 ) ) ;
#35488=CARTESIAN_POINT ( 'NONE',  ( -15.99999999999997691, 17.11489954122026447, 4.500000000000005329 ) ) ;
#35489=CARTESIAN_POINT ( 'NONE',  ( 20.11321884379431779, 40.00000000000000000, -40.61652209560084259 ) ) ;
#35501=CARTESIAN_POINT ( 'NONE',  ( 32.11716166826300167, 31.00000000000000355, 15.82712457579038912 ) ) ;
#35507=CARTESIAN_POINT ( 'NONE',  ( 84.89583333414414312, 31.00000000000000000, -5.563236982362012029 ) ) ;
#35513=CARTESIAN_POINT ( 'NONE',  ( -45.80426865612386678, 31.00000000000000355, -26.55377233851146812 ) ) ;
#35525=CARTESIAN_POINT ( 'NONE',  ( 64.36038921521112854, 39.99999999999999289, -37.17434371002195803 ) ) ;
#35552=CARTESIAN_POINT ( 'NONE',  ( 50.84997085137049311, 31.00000000000000000, -39.01959913718239648 ) ) ;
#35557=CARTESIAN_POINT ( 'NONE',  ( -3.763366191185464782, 40.00000000000000000, 57.60416666550938203 ) ) ;
#35570=CARTESIAN_POINT ( 'NONE',  ( -42.66459923921424036, 40.00000000000000000, 24.64557685607233140 ) ) ;
#35582=CARTESIAN_POINT ( 'NONE',  ( -26.95034633362163845, 31.00000000000000355, -79.72278128421110921 ) ) ;
#35597=CARTESIAN_POINT ( 'NONE',  ( -19.76500330823589735, 31.00000000000000355, -5.286999072153966139 ) ) ;
#35606=CARTESIAN_POINT ( 'NONE',  ( 23.79574588541966662, 40.00000000000000000, -6.380716493563439506 ) ) ;
#35607=CARTESIAN_POINT ( 'NONE',  ( -8.786317949316114095, 40.00000000000000000, -33.00646673686679833 ) ) ;
#35631=CARTESIAN_POINT ( 'NONE',  ( 29.96647033545507455, 40.00000000000000000, -88.27250603610892199 ) ) ;
#35637=CARTESIAN_POINT ( 'NONE',  ( -3.331996295684063192, 31.00000000000000355, 49.59602437330212865 ) ) ;
#35644=CARTESIAN_POINT ( 'NONE',  ( -36.82253293460209420, 40.00000000000000000, -63.98115709648401150 ) ) ;
#35655=CARTESIAN_POINT ( 'NONE',  ( -35.92146702467432817, 31.00000000000000355, -62.19081021767443218 ) ) ;
#35666=CARTESIAN_POINT ( 'NONE',  ( -73.90312034494817794, 31.00000000000000711, -56.84521418461152109 ) ) ;
#35667=CARTESIAN_POINT ( 'NONE',  ( -89.42636861580037078, 40.00000000000000711, -24.07434901465519417 ) ) ;
#35685=CARTESIAN_POINT ( 'NONE',  ( 26.89767027507546615, 31.00000000000000355, -1.736414864505229527 ) ) ;
#35692=CARTESIAN_POINT ( 'NONE',  ( 11.72132095739929625, 40.00000000000000000, -43.45763713125776917 ) ) ;
#35702=CARTESIAN_POINT ( 'NONE',  ( -31.00354902519490352, 31.00000000000000355, -27.18544651223506392 ) ) ;
#35706=CARTESIAN_POINT ( 'NONE',  ( -58.57471716409879292, 31.00000000000000711, 66.78942258476980953 ) ) ;
#35709=CARTESIAN_POINT ( 'NONE',  ( -60.39136959358631174, 31.00000000000000711, -16.27924862579292054 ) ) ;
#35711=CARTESIAN_POINT ( 'NONE',  ( 66.90003082753170816, 39.99999999999999289, -4.275635516647131595 ) ) ;
#35716=AXIS2_PLACEMENT_3D ( 'NONE', #32283, #2367, #39674 ) ;
#35726=CARTESIAN_POINT ( 'NONE',  ( 68.07048008643859305, 39.99999999999999289, 33.55317283102968418 ) ) ;
#35749=CARTESIAN_POINT ( 'NONE',  ( -8.160545988181935328, 31.00000000000000355, -61.88879904071598048 ) ) ;
#35753=CARTESIAN_POINT ( 'NONE',  ( 5.076274692534474831, 31.00000000000000355, 39.04542013319161953 ) ) ;
#35756=CARTESIAN_POINT ( 'NONE',  ( -41.80404827410195168, 40.00000000000000000, 54.50178954758867889 ) ) ;
#35765=CARTESIAN_POINT ( 'NONE',  ( 15.14372185054182651, 40.00000000000000000, 44.57714859939663654 ) ) ;
#35780=CARTESIAN_POINT ( 'NONE',  ( 58.29702017945731285, 31.00000000000000000, 66.63806913872474524 ) ) ;
#35781=ORIENTED_EDGE ( 'NONE', *, *, #23994, .T. ) ;
#35799=CARTESIAN_POINT ( 'NONE',  ( 23.12883206328222130, 31.00000000000000355, 11.39561251172168355 ) ) ;
#35805=CARTESIAN_POINT ( 'NONE',  ( 42.20483333784007840, 40.00000000000000000, -14.33818270462009359 ) ) ;
#35808=CARTESIAN_POINT ( 'NONE',  ( 30.20675218207097501, 40.00000000000000000, 23.25504409023340813 ) ) ;
#35832=CARTESIAN_POINT ( 'NONE',  ( 57.05379307147669721, 39.99999999999999289, -74.37948018729004218 ) ) ;
#35836=ORIENTED_EDGE ( 'NONE', *, *, #19364, .T. ) ;
#35839=CARTESIAN_POINT ( 'NONE',  ( -25.29816761085220378, 31.00000000000000355, 43.63644233510515846 ) ) ;
#35847=CARTESIAN_POINT ( 'NONE',  ( -35.33737842959504860, 40.00000000000000000, 60.98257694382487415 ) ) ;
#35862=CARTESIAN_POINT ( 'NONE',  ( -72.56464488860213180, 31.00000000000000711, -35.76892886290303863 ) ) ;
#35865=ADVANCED_FACE ( 'NONE', ( #20833 ), #17548, .T. ) ;
#35872=CARTESIAN_POINT ( 'NONE',  ( -26.02152878260477564, 31.00000000000000355, 96.68563202202810203 ) ) ;
#35873=CARTESIAN_POINT ( 'NONE',  ( 25.57473013256711880, 40.00000000000000000, 95.94174708832935039 ) ) ;
#35893=ORIENTED_EDGE ( 'NONE', *, *, #33329, .T. ) ;
#35901=CARTESIAN_POINT ( 'NONE',  ( 41.46880187714432253, 40.00000000000000000, 24.04226233541896107 ) ) ;
#35919=CARTESIAN_POINT ( 'NONE',  ( -49.89583333467011528, 31.00000000000000355, 3.272492339034415831 ) ) ;
#35927=CARTESIAN_POINT ( 'NONE',  ( 84.73112319332513209, 31.00000000000000000, -41.78253223598262167 ) ) ;
#35930=CARTESIAN_POINT ( 'NONE',  ( -28.16914340538000161, 31.00000000000000355, -57.36152490105312296 ) ) ;
#35931=CARTESIAN_POINT ( 'NONE',  ( -64.10496366469683949, 40.00000000000000711, 31.48763712508877077 ) ) ;
#35944=CARTESIAN_POINT ( 'NONE',  ( -5.072363130230006512, 40.00000000000000000, 77.60416666578095146 ) ) ;
#35978=CARTESIAN_POINT ( 'NONE',  ( -58.48566925783705983, 31.00000000000000711, -15.65830181327787862 ) ) ;
#35983=CARTESIAN_POINT ( 'NONE',  ( 36.20216622922067273, 31.00000000000000355, 9.761693653842600682 ) ) ;
#35984=CARTESIAN_POINT ( 'NONE',  ( 8.815036365794538753, 40.00000000000000000, 66.85656860134390911 ) ) ;
#35993=CARTESIAN_POINT ( 'NONE',  ( 5.583751958424166162, 40.00000000000000000, -42.43436172917101601 ) ) ;
#35996=ORIENTED_EDGE ( 'NONE', *, *, #20205, .T. ) ;
#36008=CARTESIAN_POINT ( 'NONE',  ( 86.58052584568748955, 31.00000000000000000, -42.55516686010645344 ) ) ;
#36027=CARTESIAN_POINT ( 'NONE',  ( 22.42277067908921850, 31.00000000000000355, 12.94072372014797701 ) ) ;
#36035=CARTESIAN_POINT ( 'NONE',  ( -25.53337963587170023, 40.00000000000000000, 29.12008199578403023 ) ) ;
#36037=CARTESIAN_POINT ( 'NONE',  ( -31.36635120280305955, 40.00000000000000000, -8.451140850655482595 ) ) ;
#36066=CARTESIAN_POINT ( 'NONE',  ( 3.665567271000699012, 31.00000000000000355, -54.59530427605618996 ) ) ;
#36077=CARTESIAN_POINT ( 'NONE',  ( 37.84579180138899090, 40.00000000000000000, -65.31998993212283722 ) ) ;
#36088=CARTESIAN_POINT ( 'NONE',  ( -39.25113411183426848, 31.00000000000000355, 67.98392962655870519 ) ) ;
#36099=CARTESIAN_POINT ( 'NONE',  ( -56.91377077966711084, 31.00000000000000355, -74.37798324515208037 ) ) ;
#36101=CARTESIAN_POINT ( 'NONE',  ( 93.52153384685561832, 39.99999999999999289, -24.92737483788710762 ) ) ;
#36127=CARTESIAN_POINT ( 'NONE',  ( -34.17541447290003020, 40.00000000000000000, -26.31327426976606887 ) ) ;
#36128=DIRECTION ( 'NONE',  ( 0.000000000000000000, 1.000000000000000000, 0.000000000000000000 ) ) ;
#36133=VERTEX_POINT ( 'NONE', #7187 ) ;
#36141=CARTESIAN_POINT ( 'NONE',  ( 39.77940265867437120, 31.00000000000000355, 22.96373720238702276 ) ) ;
#36145=CARTESIAN_POINT ( 'NONE',  ( 94.17930118497612568, 31.00000000000000000, -12.41473344271720691 ) ) ;
#36148=CARTESIAN_POINT ( 'NONE',  ( 41.67488199336423804, 31.00000000000000355, 54.49293397273885375 ) ) ;
#36149=CARTESIAN_POINT ( 'NONE',  ( 59.60939625460783731, 39.99999999999999289, -29.27517545779414831 ) ) ;
#36167=CARTESIAN_POINT ( 'NONE',  ( 32.44529481510334534, 40.00000000000000000, -65.82339768528792945 ) ) ;
#36192=CARTESIAN_POINT ( 'NONE',  ( -17.44537629401976631, 39.99999999999999289, -4.261559264950514958 ) ) ;
#36196=CARTESIAN_POINT ( 'NONE',  ( 25.16436199730139123, 31.00000000000000355, 51.02488717759543135 ) ) ;
#36198=CARTESIAN_POINT ( 'NONE',  ( -20.28213647682921206, 31.00000000000000355, 23.06128528321892546 ) ) ;
#36199=CARTESIAN_POINT ( 'NONE',  ( -51.86900026051868196, 40.00000000000000000, 45.50549606403863123 ) ) ;
#36208=CARTESIAN_POINT ( 'NONE',  ( 45.10416666515585860, 40.00000000000000000, 2.945243104263102651 ) ) ;
#36222=CARTESIAN_POINT ( 'NONE',  ( 87.78546986788515483, 31.00000000000000000, 43.41392487578124104 ) ) ;
#36236=CARTESIAN_POINT ( 'NONE',  ( 25.10416666396844576, 31.00000000000000355, 1.636246165087044124 ) ) ;
#36245=CARTESIAN_POINT ( 'NONE',  ( 2.454369252093185239, 40.00000000000000000, 37.39583333513270702 ) ) ;
#36246=CARTESIAN_POINT ( 'NONE',  ( 27.84166646521873645, 40.00000000000000000, -36.16032403486059366 ) ) ;
#36260=B_SPLINE_CURVE_WITH_KNOTS ( 'NONE', 3,
 ( #2660, #26898, #11190, #40172, #7232, #20827, #27331, #20375, #17757, #20592, #37772, #37564, #3951, #40821, #3719, #34502, #4170, #17104, #17335, #30610, #23860, #13604, #34289, #31030, #677, #14038, #24310, #34080, #30389, #27123, #16890, #7022, #23653, #1118, #14471, #893, #40598, #17541, #36913, #10310, #4385, #10974, #7675, #21040, #30172, #13829, #230, #10740, #37126, #33639, #27782, #33863, #24078, #466, #14244, #40391, #41038, #10524, #37343, #30816, #27549, #7889, #7462, #24521, #21252, #5051, #8328, #24732, #34939, #27996, #42105, #12054, #18410, #18200, #12264, #14688, #25169, #8534, #34732, #41701, #4839, #35148, #31469, #31673, #1772, #11621, #32105, #1555, #28840, #25371, #15545, #38628, #25591, #15125, #38417, #14902, #28204, #28429, #8112, #8754, #38849, #11841, #5267, #11399, #41254, #22109, #21893, #8972, #22318, #2184, #41472, #18634, #31897, #24963, #1983, #37989, #28633, #21479, #15341, #41905, #38212, #4612, #21686, #17988, #35368, #31257, #1339, #5485, #18843, #39902, #23171, #32522, #42331, #16179, #29476, #3019, #6530, #43181, #12481, #32306, #29695, #25994, #39252, #42966, #13338, #32731, #35993, #2388, #26421, #9178, #25793, #39478, #5896, #26634, #9384, #12898, #16630, #19892, #2815, #26206, #22740, #36208, #13128, #33165, #6118, #10029, #9616, #19469, #29061, #42740, #39053, #22530, #39685, #35765, #22964, #19253, #6330, #19676, #29268, #2612, #32943, #16389, #42536, #3249, #15974, #29921, #9819, #35570, #36417, #5689, #19044, #15755, #12685, #36865, #20539, #26845, #845, #4336, #7625, #24256, #30336, #33383, #40768, #23812, #30976, #40995, #20986, #17050, #3896, #10689, #3672, #37079, #16845, #4120, #13550, #40552, #627, #13773, #7413, #1064, #23604, #413, #34240, #17706, #30126, #23374, #27726, #10922, #20330, #183, #17280, #30564, #34033, #37518, #14417, #40121, #20123, #17488, #30769, #13983, #27282, #36638, #33809, #7182, #3467, #14198, #10254, #6970, #24026, #33592, #6762, #40341, #37293, #27072, #10472, #20772, #27495, #41420, #1719, #11140, #14640, #11570, #28798, #15074, #24913, #4557, #18363, #17935, #31206, #5214, #1293, #31623, #11350, #28382, #21641, #4795, #8058, #41651, #22059, #18152, #8286, #11800, #35320, #2141, #41202, #27947, #14853, #38164, #28152, #24681, #34890, #34451, #5438, #18581, #5007, #37938, #18803, #21199, #25126, #38371, #21428, #34678, #24468, #8489, #31420, #38579, #1504, #37722, #15503, #41860, #21854, #35100, #31851, #1936, #15302, #25327, #32057, #28590, #7840, #12010, #8701, #32476, #6281, #19846, #39211, #42493, #8929, #32900, #15707, #5643, #2768, #12436, #33110, #15927, #19425, #23127, #13083, #9339, #32691, #29224, #16131, #36167, #26380, #12639, #16580, #29433, #25952, #35525, #6073, #19006, #32262, #19630, #2341, #42697, #42283, #12850, #22693, #35726, #39007, #26158, #9775, #39433, #9570, #22921, #36376, #3199, #29015, #25755, #2568, #35944, #2976, #9131, #16340, #22278, #6487, #29645, #42924, #22485, #42060, #5852, #39647, #12219, #25542, #19208, #38800, #17228, #16793, #17002, #30288, #36816, #14153, #30079, #10865, #37243, #40718, #7357, #24203, #40293, #7138, #40064, #139, #36588, #30720, #796, #13938, #357, #30514, #6713, #39857, #4070, #13724, #37466, #4286, #27444, #23551, #10429, #586, #10202, #27026, #23332, #10643, #37030, #13502, #27232, #26796, #7579, #33341, #20938, #6925, #34190, #20077, #23762, #9982, #29878, #20716, #20493, #20281, #43142, #3425, #33759, #3841, #23977, #33545, #13290, #40504, #3630, #33982, #17444, #26587, #2451, #4505, #42395, #25653, #29122, #38911, #12538, #28103, #38111, #27895, #31154, #14802, #19105, #32367, #1667, #4740, #4955, #24420, #27675, #35631, #18102, #25853, #35832, #15815, #11299, #41366, #18310, #41150, #31367, #11092, #41597, #7791, #8236, #8007, #15021, #39119, #17877, #5747, #1012, #11517, #1242, #9240, #22589, #17660, #40945, #30926, #22381, #21594, #28328, #14362, #24631, #37673, #21151, #12328, #9028, #24857, #34840, #34400, #31575, #14589, #37884, #21372, #34622, #1449, #16902 ),
 .UNSPECIFIED., .F., .F.,
 ( 4, 2, 2, 2, 2, 2, 2, 2, 2, 2, 2, 2, 2, 2, 2, 2, 2, 2, 2, 2, 2, 2, 2, 2, 2, 2, 2, 2, 2, 2, 2, 2, 2, 2, 2, 2, 2, 2, 2, 2, 2, 2, 2, 2, 2, 2, 2, 2, 2, 2, 2, 2, 2, 2, 2, 2, 2, 2, 2, 2, 2, 2, 2, 2, 2, 2, 2, 2, 2, 2, 2, 2, 2, 2, 2, 2, 2, 2, 2, 2, 2, 2, 2, 2, 2, 2, 2, 2, 2, 2, 2, 2, 2, 2, 2, 2, 2, 2, 2, 2, 2, 2, 2, 2, 2, 2, 2, 2, 2, 2, 2, 2, 2, 2, 2, 2, 2, 2, 2, 2, 2, 2, 2, 2, 2, 2, 2, 2, 2, 2, 2, 2, 2, 2, 2, 2, 2, 2, 2, 2, 2, 2, 2, 2, 2, 2, 2, 2, 2, 2, 2, 2, 2, 2, 2, 2, 2, 2, 2, 2, 2, 2, 2, 2, 2, 2, 2, 2, 2, 2, 2, 2, 2, 2, 2, 2, 2, 2, 2, 2, 2, 2, 2, 2, 2, 2, 2, 2, 2, 2, 2, 2, 2, 2, 2, 2, 2, 2, 2, 2, 2, 2, 2, 2, 2, 2, 2, 2, 2, 2, 2, 2, 2, 2, 2, 2, 2, 2, 2, 2, 2, 2, 2, 2, 2, 2, 2, 2, 2, 2, 2, 2, 2, 2, 2, 2, 2, 2, 2, 2, 2, 2, 2, 2, 2, 2, 2, 2, 2, 2, 2, 2, 2, 2, 2, 2, 4 ),
 ( 0.000000000000000000, 0.003906250000000000000, 0.007812500000000000000, 0.01171875000000000000, 0.01562500000000000000, 0.01953125000000000000, 0.02343750000000000000, 0.02734375000000000000, 0.03125000000000000000, 0.03515625000000000000, 0.03906250000000000000, 0.04296875000000000000, 0.04687500000000000000, 0.05078125000000000000, 0.05468750000000000000, 0.05859375000000000000, 0.06250000000000000000, 0.06640625000000000000, 0.07031250000000000000, 0.07421875000000000000, 0.07812500000000000000, 0.08203125000000000000, 0.08593750000000000000, 0.08984375000000000000, 0.09375000000000000000, 0.09765625000000000000, 0.1015625000000000000, 0.1054687500000000000, 0.1093750000000000000, 0.1132812500000000000, 0.1171875000000000000, 0.1210937500000000000, 0.1250000000000000000, 0.1289062500000000000, 0.1328125000000000000, 0.1367187500000000000, 0.1406250000000000000, 0.1445312500000000000, 0.1484375000000000000, 0.1523437500000000000, 0.1562500000000000000, 0.1601562500000000000, 0.1640625000000000000, 0.1679687500000000000, 0.1718750000000000000, 0.1757812500000000000, 0.1796875000000000000, 0.1835937500000000000, 0.1875000000000000000, 0.1914062500000000000, 0.1953125000000000000, 0.1992187500000000000, 0.2031250000000000000, 0.2070312500000000000, 0.2109375000000000000, 0.2148437500000000000, 0.2187500000000000000, 0.2226562500000000000, 0.2265625000000000000, 0.2304687500000000000, 0.2343750000000000000, 0.2382812500000000000, 0.2421875000000000000, 0.2460937500000000000, 0.2500000000000000000, 0.2539062500000000000, 0.2578125000000000000, 0.2617187500000000000, 0.2656250000000000000, 0.2695312500000000000, 0.2734375000000000000, 0.2773437500000000000, 0.2812500000000000000, 0.2851562500000000000, 0.2890625000000000000, 0.2929687500000000000, 0.2968750000000000000, 0.3007812500000000000, 0.3046875000000000000, 0.3085937500000000000, 0.3125000000000000000, 0.3164062500000000000, 0.3203125000000000000, 0.3242187500000000000, 0.3281250000000000000, 0.3320312500000000000, 0.3359375000000000000, 0.3398437500000000000, 0.3437500000000000000, 0.3476562500000000000, 0.3515625000000000000, 0.3554687500000000000, 0.3593750000000000000, 0.3632812500000000000, 0.3671875000000000000, 0.3710937500000000000, 0.3750000000000000000, 0.3789062500000000000, 0.3828125000000000000, 0.3867187500000000000, 0.3906250000000000000, 0.3945312500000000000, 0.3984375000000000000, 0.4023437500000000000, 0.4062500000000000000, 0.4101562500000000000, 0.4140625000000000000, 0.4179687500000000000, 0.4218750000000000000, 0.4257812500000000000, 0.4296875000000000000, 0.4335937500000000000, 0.4375000000000000000, 0.4414062500000000000, 0.4453125000000000000, 0.4492187500000000000, 0.4531250000000000000, 0.4570312500000000000, 0.4609375000000000000, 0.4648437500000000000, 0.4687500000000000000, 0.4726562500000000000, 0.4765625000000000000, 0.4804687500000000000, 0.4843750000000000000, 0.4882812500000000000, 0.4921875000000000000, 0.4960937500000000000, 0.5000000000000000000, 0.5039062500000000000, 0.5078125000000000000, 0.5117187500000000000, 0.5156250000000000000, 0.5195312500000000000, 0.5234375000000000000, 0.5273437500000000000, 0.5312500000000000000, 0.5351562500000000000, 0.5390625000000000000, 0.5429687500000000000, 0.5468750000000000000, 0.5507812500000000000, 0.5546875000000000000, 0.5585937500000000000, 0.5625000000000000000, 0.5664062500000000000, 0.5703125000000000000, 0.5742187500000000000, 0.5781250000000000000, 0.5820312500000000000, 0.5859375000000000000, 0.5898437500000000000, 0.5937500000000000000, 0.5976562500000000000, 0.6015625000000000000, 0.6054687500000000000, 0.6093750000000000000, 0.6132812500000000000, 0.6171875000000000000, 0.6210937500000000000, 0.6250000000000000000, 0.6289062500000000000, 0.6328125000000000000, 0.6367187500000000000, 0.6406250000000000000, 0.6445312500000000000, 0.6484375000000000000, 0.6523437500000000000, 0.6562500000000000000, 0.6601562500000000000, 0.6640625000000000000, 0.6679687500000000000, 0.6718750000000000000, 0.6757812500000000000, 0.6796875000000000000, 0.6835937500000000000, 0.6875000000000000000, 0.6914062500000000000, 0.6953125000000000000, 0.6992187500000000000, 0.7031250000000000000, 0.7070312500000000000, 0.7109375000000000000, 0.7148437500000000000, 0.7187500000000000000, 0.7226562500000000000, 0.7265625000000000000, 0.7304687500000000000, 0.7343750000000000000, 0.7382812500000000000, 0.7421875000000000000, 0.7460937500000000000, 0.7500000000000000000, 0.7539062500000000000, 0.7578125000000000000, 0.7617187500000000000, 0.7656250000000000000, 0.7695312500000000000, 0.7734375000000000000, 0.7773437500000000000, 0.7812500000000000000, 0.7851562500000000000, 0.7890625000000000000, 0.7929687500000000000, 0.7968750000000000000, 0.8007812500000000000, 0.8046875000000000000, 0.8085937500000000000, 0.8125000000000000000, 0.8164062500000000000, 0.8203125000000000000, 0.8242187500000000000, 0.8281250000000000000, 0.8320312500000000000, 0.8359375000000000000, 0.8398437500000000000, 0.8437500000000000000, 0.8476562500000000000, 0.8515625000000000000, 0.8554687500000000000, 0.8593750000000000000, 0.8632812500000000000, 0.8671875000000000000, 0.8710937500000000000, 0.8750000000000000000, 0.8789062500000000000, 0.8828125000000000000, 0.8867187500000000000, 0.8906250000000000000, 0.8945312500000000000, 0.8984375000000000000, 0.9023437500000000000, 0.9062500000000000000, 0.9101562500000000000, 0.9140625000000000000, 0.9179687500000000000, 0.9218750000000000000, 0.9257812500000000000, 0.9296875000000000000, 0.9335937500000000000, 0.9375000000000000000, 0.9414062500000000000, 0.9453125000000000000, 0.9492187500000000000, 0.9531250000000000000, 0.9570312500000000000, 0.9609375000000000000, 0.9648437500000000000, 0.9687500000000000000, 0.9726562500000000000, 0.9765625000000000000, 0.9804687500000000000, 0.9843750000000000000, 0.9882812500000000000, 0.9921875000000000000, 0.9960937500000000000, 1.000000000000000000 ),
 .UNSPECIFIED. ) ;
#36277=CARTESIAN_POINT ( 'NONE',  ( -16.51797447735581059, 31.00000000000000355, -62.05742538355529803 ) ) ;
#36284=VERTEX_POINT ( 'NONE', #4799 ) ;
#36285=CARTESIAN_POINT ( 'NONE',  ( 82.09539989320980169, 39.99999999999999289, -27.75477508813643723 ) ) ;
#36298=CARTESIAN_POINT ( 'NONE',  ( -40.93297376624923345, 31.00000000000000355, -70.86912620794510076 ) ) ;
#36308=CARTESIAN_POINT ( 'NONE',  ( -41.44813913998980581, 31.00000000000000355, -84.33308812960441969 ) ) ;
#36321=DIRECTION ( 'NONE',  ( 0.000000000000000000, 0.000000000000000000, 1.000000000000000000 ) ) ;
#36327=CARTESIAN_POINT ( 'NONE',  ( 37.09854380387523776, 31.00000000000000355, 2.490183985263670685 ) ) ;
#36333=AXIS2_PLACEMENT_3D ( 'NONE', #32752, #2632, #5509 ) ;
#36335=CARTESIAN_POINT ( 'NONE',  ( 44.54779904932823342, 40.00000000000000000, -34.05916983163054113 ) ) ;
#36348=CARTESIAN_POINT ( 'NONE',  ( -47.99616210117395099, 31.00000000000000355, 12.86278070621785119 ) ) ;
#36355=CARTESIAN_POINT ( 'NONE',  ( -85.90019077458921970, 31.00000000000000711, -29.16093118951848240 ) ) ;
#36359=CARTESIAN_POINT ( 'NONE',  ( -50.06114249714176623, 31.00000000000000355, -38.53249520213265811 ) ) ;
#36360=CARTESIAN_POINT ( 'NONE',  ( -41.78821403078462282, 40.00000000000000000, -47.79414628086202299 ) ) ;
#36361=CARTESIAN_POINT ( 'NONE',  ( -49.27414759474276451, 40.00000000000000711, 85.34056160678568403 ) ) ;
#36376=CARTESIAN_POINT ( 'NONE',  ( 34.02738612458995959, 40.00000000000000000, 69.00154638599002510 ) ) ;
#36397=CARTESIAN_POINT ( 'NONE',  ( -10.86393331615775892, 31.00000000000000355, -18.79923026442779843 ) ) ;
#36398=EDGE_CURVE ( 'NONE', #42546, #36284, #22870, .T. ) ;
#36407=CARTESIAN_POINT ( 'NONE',  ( -44.33513214241411760, 31.00000000000000355, 38.89722855811361768 ) ) ;
#36409=CARTESIAN_POINT ( 'NONE',  ( -12.95950413119362743, 31.00000000000000355, 37.95406330259781669 ) ) ;
#36410=CARTESIAN_POINT ( 'NONE',  ( 64.37268382102905662, 39.99999999999999289, -8.487791176987355968 ) ) ;
#36417=CARTESIAN_POINT ( 'NONE',  ( -44.28363997456384737, 40.00000000000000000, 21.84072794957603492 ) ) ;
#36430=CARTESIAN_POINT ( 'NONE',  ( -91.90012763196533285, 31.00000000000000711, 5.898218105444796855 ) ) ;
#36450=CARTESIAN_POINT ( 'NONE',  ( 30.80114556864472775, 31.00000000000000355, -15.19345985420777190 ) ) ;
#36455=ADVANCED_FACE ( 'NONE', ( #43090 ), #13239, .T. ) ;
#36457=CARTESIAN_POINT ( 'NONE',  ( -13.53264355869793967, 40.00000000000000000, -39.83251807627727459 ) ) ;
#36458=CARTESIAN_POINT ( 'NONE',  ( -51.89982240185989326, 40.00000000000000000, 3.308651922604956219 ) ) ;
#36485=CARTESIAN_POINT ( 'NONE',  ( -15.62887661520211857, 31.00000000000000355, 57.97203279869351888 ) ) ;
#36491=ORIENTED_EDGE ( 'NONE', *, *, #3820, .T. ) ;
#36493=CARTESIAN_POINT ( 'NONE',  ( 64.75392801420538547, 39.99999999999999289, -56.64582372546511380 ) ) ;
#36498=LINE ( 'NONE', #13417, #21378 ) ;
#36506=CARTESIAN_POINT ( 'NONE',  ( 38.42722039544141666, 31.00000000000000355, 66.52996821281629991 ) ) ;
#36526=EDGE_LOOP ( 'NONE', ( #30243, #292, #29297, #1272 ) ) ;
#36536=CARTESIAN_POINT ( 'NONE',  ( 7.507699080471219588, 31.00000000000000355, 28.16210111025598195 ) ) ;
#36545=CARTESIAN_POINT ( 'NONE',  ( 27.80911911934546055, 40.00000000000000000, -47.97225535894359894 ) ) ;
#36556=CARTESIAN_POINT ( 'NONE',  ( -6.238242335983215092, 31.00000000000000355, 47.40213128959678102 ) ) ;
#36565=CARTESIAN_POINT ( 'NONE',  ( 90.64482129758324902, 31.00000000000000000, 30.77200948131585889 ) ) ;
#36572=CARTESIAN_POINT ( 'NONE',  ( 59.60939625460783731, 31.00000000000000000, -29.27517545780145269 ) ) ;
#36574=CARTESIAN_POINT ( 'NONE',  ( -20.51812799677388455, 40.00000000000000000, -60.74091093256832607 ) ) ;
#36588=CARTESIAN_POINT ( 'NONE',  ( 5.399612364985509672, 40.00000000000000000, -82.60416666586320389 ) ) ;
#36602=EDGE_LOOP ( 'NONE', ( #11901, #4683, #24462, #42965 ) ) ;
#36603=CARTESIAN_POINT ( 'NONE',  ( 3.245924575715140481, 40.00000000000000000, -24.54795925723446359 ) ) ;
#36623=CARTESIAN_POINT ( 'NONE',  ( 64.36038921521112854, 31.00000000000000000, -37.17434371002195803 ) ) ;
#36625=CARTESIAN_POINT ( 'NONE',  ( -4.434938641671373638, 31.00000000000000355, -34.07637162043106116 ) ) ;
#36627=CARTESIAN_POINT ( 'NONE',  ( 29.59587406094124873, 40.00000000000000000, 60.01321678176139329 ) ) ;
#36638=CARTESIAN_POINT ( 'NONE',  ( -3.763366191185464782, 40.00000000000000000, 57.60416666550938203 ) ) ;
#36651=CARTESIAN_POINT ( 'NONE',  ( -30.16842255227261660, 31.00000000000000355, -89.21315370691763746 ) ) ;
#36662=ADVANCED_FACE ( 'NONE', ( #17824 ), #1840, .F. ) ;
#36670=CARTESIAN_POINT ( 'NONE',  ( 32.71557229150619861, 31.00000000000000355, -11.11602612089219910 ) ) ;
#36678=CARTESIAN_POINT ( 'NONE',  ( -30.97228021248666607, 40.00000000000000000, 23.76985434021725041 ) ) ;
#36679=CARTESIAN_POINT ( 'NONE',  ( -49.95450512539639476, 40.00000000000000000, 13.28959769214884545 ) ) ;
#36691=DIRECTION ( 'NONE',  ( 0.9247238835424299586, 4.035472873002398249E-16, 0.3806385939525924744 ) ) ;
#36712=CARTESIAN_POINT ( 'NONE',  ( 66.75914267695947046, 31.00000000000000000, 8.899205196610871837 ) ) ;
#36718=B_SPLINE_SURFACE_WITH_KNOTS ( 'NONE', 1, 3, ( 
 ( #21890, #5264, #11838, #25368, #38844, #35145, #34499, #4609, #17984, #31255, #18632, #8109, #34730, #8325, #4837, #25167, #21684, #18198, #28426, #31465, #1552, #41470, #11619, #31893, #24958, #1981, #31669, #38209, #34937, #5047, #1769, #15123, #19709, #36236, #954, #23409, #19285, #35799, #36027, #32761, #6152, #9209, #19498, #12512, #26664, #39719, #2849, #42365, #25824, #29728, #32555, #6359, #2643, #26239, #16002, #29506, #16662, #9419, #19930, #12931, #23200, #29091, #6564, #3281, #16210, #42773, #9849, #32973, #29300, #42570, #32338, #22558, #39087, #33201, #29948, #16425, #39510, #3053, #5927, #12718, #13370, #9648, #39931, #6793, #10065, #26022, #22995, #43000, #39284, #13157, #22775, #26450, #36450, #36670, #2421, #15787, #4151, #27761, #20360, #7657, #3497, #17316, #7003, #1096, #14452, #21020, #30158, #41021, #24288, #33621, #24058, #3705, #14016, #17083, #30595, #4366, #40374, #34272, #659, #10957, #16875, #37545, #17737, #3930, #7216, #27529, #37327, #30368, #450, #20154, #10291, #26881, #31008, #11167, #17521, #20572, #7443, #40154, #213, #24503, #33841, #37754, #33414, #13584, #13810, #27313, #20803, #27108, #40582, #23638, #873, #36894, #34066, #10720, #10505, #30798, #23845, #37110, #14227, #40801, #5034, #37969, #32086, #2169, #38610, #17967, #28826, #12042, #11827, #18616, #18831, #1533, #15530, #25357, #8731, #31656, #41451, #11602, #15327, #42092, #18390, #8312, #35352, #25150, #28184, #5470, #38403, #21460, #12244, #24943, #28413, #25572, #22095, #1750, #41682, #38192, #8521, #7871, #11381, #4591, #8091, #21231, #21669, #28616, #15108, #34708, #41887, #21877, #35129, #34481, #31238, #5247, #14885, #31881, #1968, #1325, #14668, #34922, #27975, #41237, #24712, #4824, #18182, #31447, #42311, #42521, #39238, #12669, #15735, #25980, #19029, #33148, #3007, #9368, #5671, #32288, #36196, #9803, #19879, #16614, #2373, #43170, #6517, #26187, #22952, #16161, #29678, #13324, #39463, #36407, #39677, #32929, #29907, #9601, #16375, #23154, #22724, #38834, #29463, #35978, #29045, #2799, #12467, #25781, #42952, #39035, #42726, #9160, #12881, #6105, #32507, #35749, #6311, #3233, #2597, #19453, #19662, #13112, #22514, #8957, #15957, #22306, #35552, #29257, #5881, #19235, #32717, #26410, #30546, #37063, #3455, #20314, #13969, #40101, #4102, #13756, #7390, #13534, #1047, #27265, #26830, #27060, #40326, #33576, #10902, #10238, #7609, #34016, #37499, #17475, #20970, #7168, #3877, #36850, #23586, #23795, #30110, #30752, #34225, #24236, #27478, #3661, #17033, #614, #26617, #20751, #827, #14180, #39886, #6957, #10015, #20525, #30320, #168, #40752, #393, #33791, #10460, #10673, #17263, #4318, #40534, #17689, #24010, #30958, #23361, #33368, #36623, #6745, #20109, #37275, #16828, #38144, #8270, #25109, #28573, #22043, #21182, #11122, #8472, #21834, #21624, #18342, #34434, #34874, #31604, #4988, #1918, #40976, #1700, #21408, #15057, #38357, #35080, #24451, #14835, #28363, #41631, #11782, #25312, #5420, #1277, #17915, #18136, #28133, #31400, #4538, #1484, #37705, #8681, #5194, #41401, #7825, #31190, #18561, #14621, #31832, #27928, #15284, #41184, #11551, #41843, #34660, #11993, #38557, #35299, #11332, #18786, #32040, #24893, #14397, #27709, #24663, #37920, #8041, #4779, #35507, #8909, #2957, #16320, #29414, #32457, #32671, #22261, #12198, #19610, #2545, #9754, #19824, #29626, #38988, #25934, #2749, #25737, #15907, #38779, #26138, #5626, #19406, #22674, #35706, #42680, #23108, #2323, #32878, #28783, #42474, #32245, #26362, #39628, #42901, #25523, #36355, #6261, #6054, #12829, #13062, #9113, #6468, #2124, #15487, #39194, #5833, #19189, #9550, #42043, #12621, #29206, #18988, #16114, #22466, #15688, #39413, #28994, #42260, #9317, #35927, #12417, #22903, #36145, #10406, #20261, #23739, #33091, #36565, #29858, #33318, #10845, #23530, #10622, #335, #3404, #40483, #17422, #10181, #20694, #13701, #23953, #43121, #7332, #4048, #16982, #33526, #37220, #7118, #16772, #116, #3179, #23310, #39836, #33961, #30700, #17205, #3611 ),
 ( #36796, #40274, #30061, #30489, #13482, #24178, #6693, #776, #6902, #14131, #27425, #9961, #16553, #37440, #40693, #26773, #20053, #27002, #37011, #567, #7560, #13268, #40044, #26565, #27213, #30265, #20472, #33734, #3819, #13918, #35606, #2429, #42374, #14341, #25832, #32344, #8794, #5525, #41942, #12303, #39094, #22152, #19080, #22359, #15580, #12518, #35410, #28879, #5725, #7985, #20918, #12092, #21348, #27653, #28675, #40920, #11072, #42146, #24400, #25410, #21132, #38670, #31941, #14570, #17856, #18882, #15792, #27871, #18679, #32141, #2221, #37651, #29097, #41128, #34168, #4268, #11278, #30904, #17640, #991, #24611, #25627, #2018, #7772, #37864, #38892, #34380, #9008, #34601, #4480, #31132, #1219, #4716, #15382, #3289, #19291, #9656, #39729, #9856, #13164, #20162, #219, #39293, #12725, #12942, #23001, #26246, #29308, #39517, #32561, #3506, #16668, #36245, #2649, #16009, #6572, #9428, #26457, #22782, #3061, #36035, #6368, #36678, #29513, #39939, #32979, #8, #5933, #26670, #23417, #19716, #16433, #29954, #23208, #6159, #19504, #9214, #42576, #26028, #10071, #6800, #36457, #29737, #19938, #32773, #2856, #33420, #43007, #16883, #26891, #30165, #16216, #33207, #13378, #42780, #13592, #22565, #35805, #30379, #14234, #17532, #30601, #24296, #4602, #40380, #27770, #23644, #37335, #27116, #21238, #34491, #41028, #7013, #17976, #1108, #882, #7664, #7881, #33851, #31246, #14461, #11177, #20813, #666, #14027, #4373, #1332, #7449, #40588, #24513, #27538, #17323, #37762, #40813, #10516, #14675, #27322, #30806, #40161, #10299, #34073, #10965, #10726, #37555, #36902, #457, #20366, #23851, #33629, #24066, #17746, #4157, #37116, #31016, #21030, #34281, #3711, #17089, #13817, #3939, #7224, #20579, #34718, #4832, #22101, #18189, #35138, #28190, #31888, #38411, #21675, #24952, #15334, #38839, #34931, #25157, #28622, #1975, #31457, #28832, #5040, #35557, #19035, #18400, #37976, #22312, #8103, #31661, #41896, #8527, #1544, #1757, #12048, #41460, #5478, #15117, #8741, #14892, #2378, #25363, #11611, #28418, #41691, #11832, #12250, #38200, #8963, #35357, #5680, #18835, #32295, #21883, #5256, #8318, #18624, #38614, #32093, #2175, #27987, #25582, #42098, #15536, #41245, #11388, #24721, #21467, #23164, #36410, #33373, #12677, #42320, #39468, #22729, #19241, #6522, #19459, #22957, #42525, #42957, #25985, #36627, #32514, #43174, #35984, #26621, #13328, #22522, #15743, #20113, #3239, #39245, #35756, #9606, #36199, #26415, #29911, #23364, #5885, #12472, #9807, #19884, #6319, #19668, #2601, #32933, #39894, #10020, #6750, #9168, #29049, #25785, #3011, #13117, #16378, #33153, #39042, #29683, #15967, #16619, #29261, #9373, #39680, #6109, #32725, #2804, #16169, #29469, #42730, #12886, #26193, #20762, #17038, #13762, #3458, #36856, #10244, #4323, #17693, #30755, #33794, #34019, #23590, #13541, #20973, #3886, #11130, #21186, #30963, #40331, #27269, #4107, #27063, #17269, #40105, #27483, #6961, #17478, #24016, #37069, #834, #24455, #3664, #34229, #30117, #618, #33582, #27716, #40979, #1050, #26833, #37708, #7613, #7395, #14184, #14403, #10464, #7830, #16832, #172, #40541, #7173, #20530, #10908, #20317, #13972, #30550, #30327, #40756, #23799, #397, #24242, #10677, #37279, #37506, #11786, #15490, #5427, #31607, #25114, #21629, #38360, #34439, #37924, #31195, #34666, #12204, #24897, #11996, #1704, #4782, #41847, #8476, #21839, #22046, #17920, #35088, #41408, #41638, #1924, #28579, #1281, #34878, #5200, #18564, #31837, #2128, #25528, #21413, #8044, #38152, #4992, #8273, #11337, #18351, #14626, #28787, #25316, #15061, #27936, #41188, #15287, #18141, #38561, #31404, #28367, #1491, #8689, #18789, #11554, #35303, #32044, #42047, #24668, #38783, #8916, #4542, #14840, #28136, #2758, #29211, #25742, #13068, #25939, #29420, #5839, #6270, #19196, #43127, #38996, #6473, #42482, #33098, #19831, #28998, #22266, #26572, #9761, #32463, #42267, #16120, #42686, #32884, #36361, #29866, #12424, #18993, #16326, #29633, #12835, #26146, #9118, #39419, #3184, #16562 ) ),
 .UNSPECIFIED., .F., .F., .F.,
 ( 2, 2 ),
 ( 4, 2, 2, 2, 2, 2, 2, 2, 2, 2, 2, 2, 2, 2, 2, 2, 2, 2, 2, 2, 2, 2, 2, 2, 2, 2, 2, 2, 2, 2, 2, 2, 2, 2, 2, 2, 2, 2, 2, 2, 2, 2, 2, 2, 2, 2, 2, 2, 2, 2, 2, 2, 2, 2, 2, 2, 2, 2, 2, 2, 2, 2, 2, 2, 2, 2, 2, 2, 2, 2, 2, 2, 2, 2, 2, 2, 2, 2, 2, 2, 2, 2, 2, 2, 2, 2, 2, 2, 2, 2, 2, 2, 2, 2, 2, 2, 2, 2, 2, 2, 2, 2, 2, 2, 2, 2, 2, 2, 2, 2, 2, 2, 2, 2, 2, 2, 2, 2, 2, 2, 2, 2, 2, 2, 2, 2, 2, 2, 2, 2, 2, 2, 2, 2, 2, 2, 2, 2, 2, 2, 2, 2, 2, 2, 2, 2, 2, 2, 2, 2, 2, 2, 2, 2, 2, 2, 2, 2, 2, 2, 2, 2, 2, 2, 2, 2, 2, 2, 2, 2, 2, 2, 2, 2, 2, 2, 2, 2, 2, 2, 2, 2, 2, 2, 2, 2, 2, 2, 2, 2, 2, 2, 2, 2, 2, 2, 2, 2, 2, 2, 2, 2, 2, 2, 2, 2, 2, 2, 2, 2, 2, 2, 2, 2, 2, 2, 2, 2, 2, 2, 2, 2, 2, 2, 2, 2, 2, 2, 2, 2, 2, 2, 2, 2, 2, 2, 2, 2, 2, 2, 2, 2, 2, 2, 2, 2, 2, 2, 2, 2, 2, 2, 2, 2, 2, 2, 4 ),
 ( 0.000000000000000000, 0.4090909090909088941 ),
 ( 0.000000000000000000, 0.003906250000000000000, 0.007812500000000000000, 0.01171875000000000000, 0.01562500000000000000, 0.01953125000000000000, 0.02343750000000000000, 0.02734375000000000000, 0.03125000000000000000, 0.03515625000000000000, 0.03906250000000000000, 0.04296875000000000000, 0.04687500000000000000, 0.05078125000000000000, 0.05468750000000000000, 0.05859375000000000000, 0.06250000000000000000, 0.06640625000000000000, 0.07031250000000000000, 0.07421875000000000000, 0.07812500000000000000, 0.08203125000000000000, 0.08593750000000000000, 0.08984375000000000000, 0.09375000000000000000, 0.09765625000000000000, 0.1015625000000000000, 0.1054687500000000000, 0.1093750000000000000, 0.1132812500000000000, 0.1171875000000000000, 0.1210937500000000000, 0.1250000000000000000, 0.1289062500000000000, 0.1328125000000000000, 0.1367187500000000000, 0.1406250000000000000, 0.1445312500000000000, 0.1484375000000000000, 0.1523437500000000000, 0.1562500000000000000, 0.1601562500000000000, 0.1640625000000000000, 0.1679687500000000000, 0.1718750000000000000, 0.1757812500000000000, 0.1796875000000000000, 0.1835937500000000000, 0.1875000000000000000, 0.1914062500000000000, 0.1953125000000000000, 0.1992187500000000000, 0.2031250000000000000, 0.2070312500000000000, 0.2109375000000000000, 0.2148437500000000000, 0.2187500000000000000, 0.2226562500000000000, 0.2265625000000000000, 0.2304687500000000000, 0.2343750000000000000, 0.2382812500000000000, 0.2421875000000000000, 0.2460937500000000000, 0.2500000000000000000, 0.2539062500000000000, 0.2578125000000000000, 0.2617187500000000000, 0.2656250000000000000, 0.2695312500000000000, 0.2734375000000000000, 0.2773437500000000000, 0.2812500000000000000, 0.2851562500000000000, 0.2890625000000000000, 0.2929687500000000000, 0.2968750000000000000, 0.3007812500000000000, 0.3046875000000000000, 0.3085937500000000000, 0.3125000000000000000, 0.3164062500000000000, 0.3203125000000000000, 0.3242187500000000000, 0.3281250000000000000, 0.3320312500000000000, 0.3359375000000000000, 0.3398437500000000000, 0.3437500000000000000, 0.3476562500000000000, 0.3515625000000000000, 0.3554687500000000000, 0.3593750000000000000, 0.3632812500000000000, 0.3671875000000000000, 0.3710937500000000000, 0.3750000000000000000, 0.3789062500000000000, 0.3828125000000000000, 0.3867187500000000000, 0.3906250000000000000, 0.3945312500000000000, 0.3984375000000000000, 0.4023437500000000000, 0.4062500000000000000, 0.4101562500000000000, 0.4140625000000000000, 0.4179687500000000000, 0.4218750000000000000, 0.4257812500000000000, 0.4296875000000000000, 0.4335937500000000000, 0.4375000000000000000, 0.4414062500000000000, 0.4453125000000000000, 0.4492187500000000000, 0.4531250000000000000, 0.4570312500000000000, 0.4609375000000000000, 0.4648437500000000000, 0.4687500000000000000, 0.4726562500000000000, 0.4765625000000000000, 0.4804687500000000000, 0.4843750000000000000, 0.4882812500000000000, 0.4921875000000000000, 0.4960937500000000000, 0.5000000000000000000, 0.5039062500000000000, 0.5078125000000000000, 0.5117187500000000000, 0.5156250000000000000, 0.5195312500000000000, 0.5234375000000000000, 0.5273437500000000000, 0.5312500000000000000, 0.5351562500000000000, 0.5390625000000000000, 0.5429687500000000000, 0.5468750000000000000, 0.5507812500000000000, 0.5546875000000000000, 0.5585937500000000000, 0.5625000000000000000, 0.5664062500000000000, 0.5703125000000000000, 0.5742187500000000000, 0.5781250000000000000, 0.5820312500000000000, 0.5859375000000000000, 0.5898437500000000000, 0.5937500000000000000, 0.5976562500000000000, 0.6015625000000000000, 0.6054687500000000000, 0.6093750000000000000, 0.6132812500000000000, 0.6171875000000000000, 0.6210937500000000000, 0.6250000000000000000, 0.6289062500000000000, 0.6328125000000000000, 0.6367187500000000000, 0.6406250000000000000, 0.6445312500000000000, 0.6484375000000000000, 0.6523437500000000000, 0.6562500000000000000, 0.6601562500000000000, 0.6640625000000000000, 0.6679687500000000000, 0.6718750000000000000, 0.6757812500000000000, 0.6796875000000000000, 0.6835937500000000000, 0.6875000000000000000, 0.6914062500000000000, 0.6953125000000000000, 0.6992187500000000000, 0.7031250000000000000, 0.7070312500000000000, 0.7109375000000000000, 0.7148437500000000000, 0.7187500000000000000, 0.7226562500000000000, 0.7265625000000000000, 0.7304687500000000000, 0.7343750000000000000, 0.7382812500000000000, 0.7421875000000000000, 0.7460937500000000000, 0.7500000000000000000, 0.7539062500000000000, 0.7578125000000000000, 0.7617187500000000000, 0.7656250000000000000, 0.7695312500000000000, 0.7734375000000000000, 0.7773437500000000000, 0.7812500000000000000, 0.7851562500000000000, 0.7890625000000000000, 0.7929687500000000000, 0.7968750000000000000, 0.8007812500000000000, 0.8046875000000000000, 0.8085937500000000000, 0.8125000000000000000, 0.8164062500000000000, 0.8203125000000000000, 0.8242187500000000000, 0.8281250000000000000, 0.8320312500000000000, 0.8359375000000000000, 0.8398437500000000000, 0.8437500000000000000, 0.8476562500000000000, 0.8515625000000000000, 0.8554687500000000000, 0.8593750000000000000, 0.8632812500000000000, 0.8671875000000000000, 0.8710937500000000000, 0.8750000000000000000, 0.8789062500000000000, 0.8828125000000000000, 0.8867187500000000000, 0.8906250000000000000, 0.8945312500000000000, 0.8984375000000000000, 0.9023437500000000000, 0.9062500000000000000, 0.9101562500000000000, 0.9140625000000000000, 0.9179687500000000000, 0.9218750000000000000, 0.9257812500000000000, 0.9296875000000000000, 0.9335937500000000000, 0.9375000000000000000, 0.9414062500000000000, 0.9453125000000000000, 0.9492187500000000000, 0.9531250000000000000, 0.9570312500000000000, 0.9609375000000000000, 0.9648437500000000000, 0.9687500000000000000, 0.9726562500000000000, 0.9765625000000000000, 0.9804687500000000000, 0.9843750000000000000, 0.9882812500000000000, 0.9921875000000000000, 0.9960937500000000000, 1.000000000000000000 ),
 .UNSPECIFIED. ) ;
#36720=CARTESIAN_POINT ( 'NONE',  ( -25.88810397297939403, 40.00000000000000000, 75.89534075015936310 ) ) ;
#36723=CARTESIAN_POINT ( 'NONE',  ( -105.9879088449591933, 31.00000000000000000, -4.880719929157669945 ) ) ;
#36732=CARTESIAN_POINT ( 'NONE',  ( 74.89583333416871369, 31.00000000000000000, -4.908738512848213276 ) ) ;
#36756=DIRECTION ( 'NONE',  ( 0.000000000000000000, -7.709882115452474222E-16, -1.000000000000000000 ) ) ;
#36765=CARTESIAN_POINT ( 'NONE',  ( -3.925388345519843725, 31.00000000000000355, 29.51202942214661462 ) ) ;
#36774=CARTESIAN_POINT ( 'NONE',  ( 33.95200755731382714, 40.00000000000000000, -44.10258293181757949 ) ) ;
#36787=CARTESIAN_POINT ( 'NONE',  ( -42.66459923921424036, 31.00000000000000355, 24.64557685607233140 ) ) ;
#36796=CARTESIAN_POINT ( 'NONE',  ( -19.99999999999999645, 40.00000000000000000, 0.000000000000000000 ) ) ;
#36798=VECTOR ( 'NONE', #24087, 1000.000000000000000 ) ;
#36802=CARTESIAN_POINT ( 'NONE',  ( 34.80713033128647993, 31.00000000000000355, 70.84796410819511436 ) ) ;
#36803=CARTESIAN_POINT ( 'NONE',  ( -40.35386350238497499, 40.00000000000000000, 69.65762217234959053 ) ) ;
#36812=EDGE_CURVE ( 'NONE', #29181, #42330, #6395, .T. ) ;
#36816=CARTESIAN_POINT ( 'NONE',  ( -72.56464488860213180, 40.00000000000000711, -35.76892886290303863 ) ) ;
#36819=CARTESIAN_POINT ( 'NONE',  ( -20.39032260654148132, 40.00000000000000000, 1.150830359615497844 ) ) ;
#36831=CARTESIAN_POINT ( 'NONE',  ( 22.71825314374767402, 40.00000000000000000, -13.09499307598873941 ) ) ;
#36834=EDGE_CURVE ( 'NONE', #35069, #7867, #32591, .T. ) ;
#36841=FILL_AREA_STYLE ('',( #27641 ) ) ;
#36843=CARTESIAN_POINT ( 'NONE',  ( -18.08361268445098347, 31.00000000000000355, -10.43497034982449456 ) ) ;
#36850=CARTESIAN_POINT ( 'NONE',  ( -51.86900026051868196, 31.00000000000000355, 45.50549606403863123 ) ) ;
#36855=CARTESIAN_POINT ( 'NONE',  ( 45.06603723660748528, 31.00000000000000355, 15.38899812203272788 ) ) ;
#36856=CARTESIAN_POINT ( 'NONE',  ( 74.72486387243833406, 39.99999999999999289, 9.837939412698395003 ) ) ;
#36865=CARTESIAN_POINT ( 'NONE',  ( -50.10416666532988472, 40.00000000000000000, -3.272492339034341224 ) ) ;
#36877=CARTESIAN_POINT ( 'NONE',  ( 28.55926749297819711, 31.00000000000000355, 84.46800049165048563 ) ) ;
#36890=CARTESIAN_POINT ( 'NONE',  ( -21.03271207055027503, 40.00000000000000000, 3.044856699593507354 ) ) ;
#36894=CARTESIAN_POINT ( 'NONE',  ( 26.55430347651023837, 31.00000000000000355, -34.62409890758566178 ) ) ;
#36902=CARTESIAN_POINT ( 'NONE',  ( -22.94860596549062848, 40.00000000000000000, -46.53072237555588231 ) ) ;
#36903=CARTESIAN_POINT ( 'NONE',  ( 11.72132095739929625, 40.00000000000000000, -43.45763713125776917 ) ) ;
#36913=CARTESIAN_POINT ( 'NONE',  ( 22.42277067908921850, 40.00000000000000000, 12.94072372014797701 ) ) ;
#36928=CARTESIAN_POINT ( 'NONE',  ( 49.67886955982877595, 31.00000000000000355, -43.43868092391004865 ) ) ;
#36936=CARTESIAN_POINT ( 'NONE',  ( 5.650912336215121456, 40.00000000000000000, -84.59266001511657862 ) ) ;
#36949=CARTESIAN_POINT ( 'NONE',  ( 75.74279358916429317, 31.00000000000000000, -37.35102017232331661 ) ) ;
#36980=CARTESIAN_POINT ( 'NONE',  ( 35.58384423644163519, 31.00000000000000355, 12.14845634898874138 ) ) ;
#36989=CARTESIAN_POINT ( 'NONE',  ( -23.74678488968044832, 40.00000000000000000, -48.36925102894097961 ) ) ;
#36999=DIRECTION ( 'NONE',  ( 0.000000000000000000, 1.000000000000000000, 0.000000000000000000 ) ) ;
#37001=CARTESIAN_POINT ( 'NONE',  ( -4.090615425948576522, 31.00000000000000355, -62.39583333438447710 ) ) ;
#37011=CARTESIAN_POINT ( 'NONE',  ( 2.965790448435745574, 40.00000000000000000, -22.56328348808469997 ) ) ;
#37016=CARTESIAN_POINT ( 'NONE',  ( 74.90833963775308746, 31.00000000000000000, 20.17845691862754975 ) ) ;
#37017=CARTESIAN_POINT ( 'NONE',  ( 76.90008882636699639, 39.99999999999999289, -4.923574515426283327 ) ) ;
#37030=CARTESIAN_POINT ( 'NONE',  ( 77.05880969081472642, 39.99999999999999289, 37.98468489477117771 ) ) ;
#37045=CARTESIAN_POINT ( 'NONE',  ( 11.19416946702162718, 40.00000000000000000, -22.66942529387992522 ) ) ;
#37063=CARTESIAN_POINT ( 'NONE',  ( 65.10416666562252885, 31.00000000000000000, 4.254240043327690124 ) ) ;
#37067=CARTESIAN_POINT ( 'NONE',  ( 15.70068437845899290, 31.00000000000000355, 46.50252577710988078 ) ) ;
#37069=CARTESIAN_POINT ( 'NONE',  ( -62.77658523491555798, 40.00000000000000711, 48.16944601536268777 ) ) ;
#37079=CARTESIAN_POINT ( 'NONE',  ( 13.71368254939966036, 40.00000000000000000, -51.22554439249349656 ) ) ;
#37105=PLANE ( 'NONE',  #38145 ) ;
#37110=CARTESIAN_POINT ( 'NONE',  ( 42.20483333784007840, 31.00000000000000355, -14.33818270462009359 ) ) ;
#37116=CARTESIAN_POINT ( 'NONE',  ( 17.07784400123870938, 40.00000000000000000, -50.31546185293520779 ) ) ;
#37117=CARTESIAN_POINT ( 'NONE',  ( 24.31498657911848227, 40.00000000000000000, 42.27453502171530175 ) ) ;
#37126=CARTESIAN_POINT ( 'NONE',  ( 1.799870782497353439, 40.00000000000000000, 27.39583333577991908 ) ) ;
#37142=CARTESIAN_POINT ( 'NONE',  ( 40.05902963217418744, 31.00000000000000355, -52.04757428483648596 ) ) ;
#37150=CARTESIAN_POINT ( 'NONE',  ( 22.12670472277728706, 40.00000000000000000, -82.16725659058069198 ) ) ;
#37162=CARTESIAN_POINT ( 'NONE',  ( -12.08748825390017068, 31.00000000000000355, -91.69541640458645304 ) ) ;
#37191=ORIENTED_EDGE ( 'NONE', *, *, #17270, .F. ) ;
#37192=CARTESIAN_POINT ( 'NONE',  ( 23.59836588145513048, 31.00000000000000355, -26.81698947917456266 ) ) ;
#37200=DIRECTION ( 'NONE',  ( 0.000000000000000000, 1.000000000000000000, -1.060184893785364939E-15 ) ) ;
#37201=CARTESIAN_POINT ( 'NONE',  ( -38.36856355434107968, 40.00000000000000000, 33.53830235993100217 ) ) ;
#37213=CARTESIAN_POINT ( 'NONE',  ( -51.34291522965900612, 31.00000000000000355, 29.65708359768123970 ) ) ;
#37220=CARTESIAN_POINT ( 'NONE',  ( -60.10374203099167545, 31.00000000000000711, 78.35501831527777483 ) ) ;
#37225=CARTESIAN_POINT ( 'NONE',  ( -23.73339997550686675, 31.00000000000000355, -70.23208777904191891 ) ) ;
#37226=CARTESIAN_POINT ( 'NONE',  ( -44.72205690102931896, 40.00000000000000000, -58.47036224960022111 ) ) ;
#37228=AXIS2_PLACEMENT_3D ( 'NONE', #18535, #41378, #28759 ) ;
#37243=CARTESIAN_POINT ( 'NONE',  ( -53.76583044639610165, 40.00000000000000000, -61.28633540801820345 ) ) ;
#37249=DIRECTION ( 'NONE',  ( 0.000000000000000000, -7.709882115452471264E-16, -1.000000000000000000 ) ) ;
#37250=ADVANCED_FACE ( 'NONE', ( #25807 ), #21906, .F. ) ;
#37268=DIRECTION ( 'NONE',  ( -0.000000000000000000, 5.297542245118643184E-16, 1.000000000000000000 ) ) ;
#37269=CARTESIAN_POINT ( 'NONE',  ( -21.73352778766994575, 31.00000000000000355, 19.07242603999910457 ) ) ;
#37275=CARTESIAN_POINT ( 'NONE',  ( 72.19657831791809599, 31.00000000000000000, -19.34484491892447622 ) ) ;
#37277=CARTESIAN_POINT ( 'NONE',  ( -6.590854309045712789, 31.00000000000000355, 49.37518673228670707 ) ) ;
#37279=CARTESIAN_POINT ( 'NONE',  ( 75.74279358916429317, 39.99999999999999289, -37.35102017232331661 ) ) ;
#37293=CARTESIAN_POINT ( 'NONE',  ( -53.27196957865878346, 40.00000000000000711, 26.27224001323269320 ) ) ;
#37311=CARTESIAN_POINT ( 'NONE',  ( -13.16936484334534008, 31.00000000000000355, 99.04657264463375554 ) ) ;
#37327=CARTESIAN_POINT ( 'NONE',  ( -38.31599561464027914, 31.00000000000000355, 10.26995502114586678 ) ) ;
#37335=CARTESIAN_POINT ( 'NONE',  ( 36.61186797162192619, 40.00000000000000000, 28.07927795628900469 ) ) ;
#37336=CARTESIAN_POINT ( 'NONE',  ( 42.13926417418816328, 40.00000000000000000, -36.83769365845790134 ) ) ;
#37343=CARTESIAN_POINT ( 'NONE',  ( -23.02120395722396395, 40.00000000000000000, 17.66995642160909696 ) ) ;
#37363=CARTESIAN_POINT ( 'NONE',  ( 76.30724621508588257, 31.00000000000000000, -9.942258256679791018 ) ) ;
#37374=CARTESIAN_POINT ( 'NONE',  ( -79.17211738000736432, 40.00000000000000711, 45.58486055166100215 ) ) ;
#37383=CARTESIAN_POINT ( 'NONE',  ( 28.03234818517180216, 31.00000000000000355, 82.53419278363811884 ) ) ;
#37411=CARTESIAN_POINT ( 'NONE',  ( -42.09738266246711191, 31.00000000000000355, -2.828681863544771691 ) ) ;
#37412=LINE ( 'NONE', #24148, #20991 ) ;
#37421=CARTESIAN_POINT ( 'NONE',  ( -37.00582609754565766, 40.00000000000000000, 48.07482304778140758 ) ) ;
#37434=CARTESIAN_POINT ( 'NONE',  ( 48.45771864870608425, 31.00000000000000355, 27.97524394371832202 ) ) ;
#37436=VERTEX_POINT ( 'NONE', #3263 ) ;
#37440=CARTESIAN_POINT ( 'NONE',  ( -7.088330391075835735, 40.00000000000000000, -20.85399598300688595 ) ) ;
#37447=CARTESIAN_POINT ( 'NONE',  ( 60.45897909542819804, 31.00000000000000000, -46.24578392211154210 ) ) ;
#37448=CARTESIAN_POINT ( 'NONE',  ( 46.16409756962309530, 40.00000000000000000, -59.99419878592187416 ) ) ;
#37466=CARTESIAN_POINT ( 'NONE',  ( 73.03870520561201829, 39.99999999999999289, -42.18585045165268355 ) ) ;
#37478=CARTESIAN_POINT ( 'NONE',  ( 28.62564328229377608, 40.00000000000000000, -21.88780996305825965 ) ) ;
#37493=CARTESIAN_POINT ( 'NONE',  ( 17.42035916340572399, 31.00000000000000355, 19.85006075799527991 ) ) ;
#37499=CARTESIAN_POINT ( 'NONE',  ( -21.91107887650263564, 31.00000000000000355, 64.54935342160338507 ) ) ;
#37503=CARTESIAN_POINT ( 'NONE',  ( -34.17541447290002310, 31.00000000000000355, -26.31327426976606176 ) ) ;
#37506=CARTESIAN_POINT ( 'NONE',  ( 80.16187752211510542, 39.99999999999999289, -27.22680903928618434 ) ) ;
#37518=CARTESIAN_POINT ( 'NONE',  ( 37.24516168167158270, 40.00000000000000000, 42.45166511289891531 ) ) ;
#37532=CARTESIAN_POINT ( 'NONE',  ( -101.9001375416480499, 31.00000000000000711, 6.549163350515033954 ) ) ;
#37541=CARTESIAN_POINT ( 'NONE',  ( -15.99999999999997691, 17.11489954122026447, 2.500000000000006217 ) ) ;
#37545=CARTESIAN_POINT ( 'NONE',  ( -29.26739590608564967, 31.00000000000000355, 25.68069354617348665 ) ) ;
#37555=CARTESIAN_POINT ( 'NONE',  ( -25.89845354150052259, 40.00000000000000000, -44.83417823681238445 ) ) ;
#37556=CARTESIAN_POINT ( 'NONE',  ( -26.77709713318651552, 40.00000000000000000, 54.08981485145582724 ) ) ;
#37564=CARTESIAN_POINT ( 'NONE',  ( -10.86393331615775892, 40.00000000000000000, -18.79923026442779843 ) ) ;
#37580=CARTESIAN_POINT ( 'NONE',  ( -64.10496366466531981, 31.00000000000000711, 31.48763712508877077 ) ) ;
#37587=CARTESIAN_POINT ( 'NONE',  ( 47.87658044100083288, 39.99999999999999289, -82.67148682534872250 ) ) ;
#37596=CARTESIAN_POINT ( 'NONE',  ( -89.62817255407412631, 31.00000000000000711, -11.80141054548196422 ) ) ;
#37601=CARTESIAN_POINT ( 'NONE',  ( -14.30682334061562422, 40.00000000000000000, -18.65445469299709202 ) ) ;
#37604=CARTESIAN_POINT ( 'NONE',  ( -105.9879088449591933, 17.11489954122026447, -0.3807199291576673361 ) ) ;
#37626=CARTESIAN_POINT ( 'NONE',  ( 29.49207856985708176, 31.00000000000000355, 38.57905506995707867 ) ) ;
#37633=CARTESIAN_POINT ( 'NONE',  ( -3.998040010416403334, 40.00000000000000000, 59.59469406578620720 ) ) ;
#37641=LINE ( 'NONE', #324, #24837 ) ;
#37643=CARTESIAN_POINT ( 'NONE',  ( -37.49462465745612860, 31.00000000000000355, -48.86220178749748300 ) ) ;
#37651=CARTESIAN_POINT ( 'NONE',  ( -24.68525358734468611, 40.00000000000000000, -18.92943107747915832 ) ) ;
#37657=CARTESIAN_POINT ( 'NONE',  ( 76.90008882636698218, 31.00000000000000000, -4.923574515426284215 ) ) ;
#37658=CARTESIAN_POINT ( 'NONE',  ( 34.80713033128647993, 40.00000000000000000, 70.84796410819511436 ) ) ;
#37673=CARTESIAN_POINT ( 'NONE',  ( -31.57754862722326905, 40.00000000000000000, 93.01713655900283584 ) ) ;
#37678=LINE ( 'NONE', #11755, #12732 ) ;
#37686=CARTESIAN_POINT ( 'NONE',  ( -22.00208165626150603, 40.00000000000000000, -25.16137218361809857 ) ) ;
#37698=CARTESIAN_POINT ( 'NONE',  ( -29.89583333557403222, 31.00000000000000355, 1.963495399902740690 ) ) ;
#37705=CARTESIAN_POINT ( 'NONE',  ( -76.41092972884307244, 31.00000000000000711, -25.93877460596726436 ) ) ;
#37707=CARTESIAN_POINT ( 'NONE',  ( -39.38196478161825809, 31.00000000000000355, 13.29643045357694398 ) ) ;
#37708=CARTESIAN_POINT ( 'NONE',  ( -70.15350862410126354, 40.00000000000000711, -40.50401079722123399 ) ) ;
#37722=CARTESIAN_POINT ( 'NONE',  ( -17.60292107714122878, 40.00000000000000000, 65.74579412301164894 ) ) ;
#37736=ORIENTED_EDGE ( 'NONE', *, *, #38389, .F. ) ;
#37754=CARTESIAN_POINT ( 'NONE',  ( -13.53264355869793967, 31.00000000000000355, -39.83251807627727459 ) ) ;
#37762=CARTESIAN_POINT ( 'NONE',  ( -49.89583333467011528, 40.00000000000000000, 3.272492339034415831 ) ) ;
#37763=CARTESIAN_POINT ( 'NONE',  ( 50.61746024623599993, 40.00000000000000000, -24.85206051842255093 ) ) ;
#37765=DIRECTION ( 'NONE',  ( 0.000000000000000000, 0.000000000000000000, 1.000000000000000000 ) ) ;
#37772=CARTESIAN_POINT ( 'NONE',  ( -13.09503298281258132, 40.00000000000000000, -17.05789676611946959 ) ) ;
#37788=CARTESIAN_POINT ( 'NONE',  ( -18.22940504111061344, 31.00000000000000355, 67.64968002090884625 ) ) ;
#37798=CARTESIAN_POINT ( 'NONE',  ( 76.36627019849126441, 39.99999999999999289, -58.43797548694632127 ) ) ;
#37808=CARTESIAN_POINT ( 'NONE',  ( 43.43872713698582544, 31.00000000000000355, 75.20828420317944563 ) ) ;
#37812=CARTESIAN_POINT ( 'NONE',  ( -23.27229071022945561, 40.00000000000000000, 20.35677778009942074 ) ) ;
#37823=ORIENTED_EDGE ( 'NONE', *, *, #12975, .F. ) ;
#37828=ORIENTED_EDGE ( 'NONE', *, *, #34378, .F. ) ;
#37835=CARTESIAN_POINT ( 'NONE',  ( 2.996940313443769099, 31.00000000000000355, -44.59688583547567475 ) ) ;
#37844=CARTESIAN_POINT ( 'NONE',  ( 8.570044366896553356, 40.00000000000000000, -64.27561742002654910 ) ) ;
#37857=CARTESIAN_POINT ( 'NONE',  ( -3.763366191185464782, 31.00000000000000355, 57.60416666550938203 ) ) ;
#37864=CARTESIAN_POINT ( 'NONE',  ( 10.63353083439206870, 40.00000000000000000, -31.33693976183458219 ) ) ;
#37868=CARTESIAN_POINT ( 'NONE',  ( 22.12670472278668399, 31.00000000000000355, -82.16725659058067777 ) ) ;
#37869=CARTESIAN_POINT ( 'NONE',  ( 22.12670472277728706, 40.00000000000000000, -82.16725659058069198 ) ) ;
#37880=DIRECTION ( 'NONE',  ( -0.9470131699890049770, 0.000000000000000000, -0.3211947320043963550 ) ) ;
#37883=CIRCLE ( 'NONE', #29521, 2.000000000000000888 ) ;
#37884=CARTESIAN_POINT ( 'NONE',  ( -94.39576909109665337, 40.00000000000000711, 32.06004391471374504 ) ) ;
#37899=CARTESIAN_POINT ( 'NONE',  ( -9.709369018688819963, 40.00000000000000000, 28.47525938324995920 ) ) ;
#37913=CARTESIAN_POINT ( 'NONE',  ( 20.70971545910534672, 31.00000000000000355, 15.87948211774388518 ) ) ;
#37918=AXIS2_PLACEMENT_3D ( 'NONE', #31638, #28606, #11586 ) ;
#37920=CARTESIAN_POINT ( 'NONE',  ( 80.16187752211510542, 31.00000000000000000, -27.22680903928618434 ) ) ;
#37922=CARTESIAN_POINT ( 'NONE',  ( -40.56882557770292408, 31.00000000000000355, 31.01417895415301373 ) ) ;
#37924=CARTESIAN_POINT ( 'NONE',  ( 74.49266661913014786, 39.99999999999999289, 43.00976416799198176 ) ) ;
#37938=CARTESIAN_POINT ( 'NONE',  ( 52.51402048354923835, 40.00000000000000000, 40.27907379435107060 ) ) ;
#37969=CARTESIAN_POINT ( 'NONE',  ( 45.10416666515585860, 31.00000000000000355, 2.945243104263102651 ) ) ;
#37976=CARTESIAN_POINT ( 'NONE',  ( -18.68892229297488683, 40.00000000000000000, 55.06009237583231197 ) ) ;
#37978=CARTESIAN_POINT ( 'NONE',  ( 55.55275676651330485, 40.00000000000000000, 14.97830846782891712 ) ) ;
#37989=CARTESIAN_POINT ( 'NONE',  ( -9.824444021593908616, 40.00000000000000000, 36.70529466175499778 ) ) ;
#38002=CARTESIAN_POINT ( 'NONE',  ( -9.228224334391116557, 31.00000000000000355, 69.24269282083176336 ) ) ;
#38013=CARTESIAN_POINT ( 'NONE',  ( 86.58052584568750376, 39.99999999999999289, -42.55516686010646765 ) ) ;
#38014=CARTESIAN_POINT ( 'NONE',  ( 3.798394181603659270, 31.00000000000000355, 29.10671710469610574 ) ) ;
#38028=CARTESIAN_POINT ( 'NONE',  ( 94.89583333399441756, 31.00000000000000000, -6.217735451874103703 ) ) ;
#38031=CARTESIAN_POINT ( 'NONE',  ( -9.709369018688819963, 40.00000000000000000, 28.47525938324995920 ) ) ;
#38053=CARTESIAN_POINT ( 'NONE',  ( -15.99999999999997691, 40.00000000000000000, 5.571627607371296764E-15 ) ) ;
#38064=CARTESIAN_POINT ( 'NONE',  ( -41.52979953746218911, 31.00000000000000355, 5.398177843165337109 ) ) ;
#38071=CARTESIAN_POINT ( 'NONE',  ( 66.90003082753170816, 39.99999999999999289, -4.275635516647131595 ) ) ;
#38083=CARTESIAN_POINT ( 'NONE',  ( -69.89583333424914713, 31.00000000000000711, 4.581489278091138040 ) ) ;
#38093=CARTESIAN_POINT ( 'NONE',  ( -5.980347265640405752, 31.00000000000000355, 89.59238221257746204 ) ) ;
#38094=CARTESIAN_POINT ( 'NONE',  ( 22.98560153735141043, 40.00000000000000000, 86.26083236265425569 ) ) ;
#38099=EDGE_LOOP ( 'NONE', ( #2154, #589, #1835, #5637 ) ) ;
#38111=CARTESIAN_POINT ( 'NONE',  ( -60.37409795221152109, 40.00000000000000711, -68.82020352599361956 ) ) ;
#38126=CARTESIAN_POINT ( 'NONE',  ( -31.89861325429239258, 40.00000000000000000, 2.042328591206914012 ) ) ;
#38138=CARTESIAN_POINT ( 'NONE',  ( -30.10416666442597844, 31.00000000000000355, -1.963495399902747574 ) ) ;
#38144=CARTESIAN_POINT ( 'NONE',  ( 74.89583333416871369, 31.00000000000000000, -4.908738512848213276 ) ) ;
#38145=AXIS2_PLACEMENT_3D ( 'NONE', #7210, #2846, #39927 ) ;
#38150=CARTESIAN_POINT ( 'NONE',  ( -15.62887661520211857, 31.00000000000000355, 57.97203279869351888 ) ) ;
#38152=CARTESIAN_POINT ( 'NONE',  ( -90.10416666596678681, 40.00000000000000711, -5.890486217120279200 ) ) ;
#38164=CARTESIAN_POINT ( 'NONE',  ( 64.37268382102905662, 39.99999999999999289, -8.487791176987355968 ) ) ;
#38169=CARTESIAN_POINT ( 'NONE',  ( -16.80298683001096904, 40.00000000000000000, -2.367532924972506336 ) ) ;
#38185=EDGE_CURVE ( 'NONE', #19261, #6230, #19603, .T. ) ;
#38192=CARTESIAN_POINT ( 'NONE',  ( -48.80550277073417931, 31.00000000000000355, -13.06547612810710035 ) ) ;
#38200=CARTESIAN_POINT ( 'NONE',  ( -40.54929543462775143, 40.00000000000000000, -46.21859917192507794 ) ) ;
#38203=CARTESIAN_POINT ( 'NONE',  ( 24.55685208795062380, 40.00000000000000000, -49.59815698162134368 ) ) ;
#38209=CARTESIAN_POINT ( 'NONE',  ( 20.96880926229634312, 31.00000000000000355, -12.11681000168150213 ) ) ;
#38212=CARTESIAN_POINT ( 'NONE',  ( -25.53337963587170023, 40.00000000000000000, 29.12008199578403023 ) ) ;
#38226=CARTESIAN_POINT ( 'NONE',  ( -70.06919973877657526, 31.00000000000000711, -18.87919424805730984 ) ) ;
#38236=CARTESIAN_POINT ( 'NONE',  ( 6.473670811831355287, 31.00000000000000355, -24.11571013580713441 ) ) ;
#38247=CARTESIAN_POINT ( 'NONE',  ( 41.30831894254264824, 31.00000000000000355, -83.80005689411834169 ) ) ;
#38251=CARTESIAN_POINT ( 'NONE',  ( 22.27703560431449148, 40.00000000000000000, 17.12883495622503816 ) ) ;
#38257=LINE ( 'NONE', #34553, #19247 ) ;
#38277=CARTESIAN_POINT ( 'NONE',  ( -37.13421060599358725, 31.00000000000000355, -21.52932707635455500 ) ) ;
#38283=CYLINDRICAL_SURFACE ( 'NONE', #448, 4.500000000000000888 ) ;
#38284=CARTESIAN_POINT ( 'NONE',  ( -30.31917247939794180, 40.00000000000000000, 52.30862930535366928 ) ) ;
#38299=CARTESIAN_POINT ( 'NONE',  ( 62.51641183113888900, 31.00000000000000000, -16.75201923384928548 ) ) ;
#38306=CARTESIAN_POINT ( 'NONE',  ( -81.66074000183850501, 31.00000000000000711, -10.87165890510346422 ) ) ;
#38307=CARTESIAN_POINT ( 'NONE',  ( 83.84057477258951963, 39.99999999999999289, -22.33845567676512900 ) ) ;
#38333=CARTESIAN_POINT ( 'NONE',  ( 36.20216622922067984, 40.00000000000000000, 9.761693653842600682 ) ) ;
#38350=CARTESIAN_POINT ( 'NONE',  ( 27.23661496637203427, 31.00000000000000355, 23.88131275951389654 ) ) ;
#38357=CARTESIAN_POINT ( 'NONE',  ( -25.13323546007955045, 31.00000000000000355, 74.03861446737784036 ) ) ;
#38359=CARTESIAN_POINT ( 'NONE',  ( 51.84393115708665079, 31.00000000000000355, 25.66707601012906892 ) ) ;
#38360=CARTESIAN_POINT ( 'NONE',  ( 81.15556025174309696, 39.99999999999999289, 27.54985289775053658 ) ) ;
#38371=CARTESIAN_POINT ( 'NONE',  ( 33.41571365387085280, 40.00000000000000000, 57.85165222247763239 ) ) ;
#38389=EDGE_CURVE ( 'NONE', #1383, #19619, #26125, .T. ) ;
#38403=CARTESIAN_POINT ( 'NONE',  ( -38.92335646797288717, 31.00000000000000355, 29.86975225897632313 ) ) ;
#38411=CARTESIAN_POINT ( 'NONE',  ( 50.09382087749727930, 40.00000000000000000, 24.69014870349942825 ) ) ;
#38417=CARTESIAN_POINT ( 'NONE',  ( 33.47591237148697729, 40.00000000000000000, -8.973542178613062248 ) ) ;
#38431=CARTESIAN_POINT ( 'NONE',  ( -81.66074000183850501, 31.00000000000000711, -10.87165890510346422 ) ) ;
#38438=CARTESIAN_POINT ( 'NONE',  ( -61.42214656771047743, 40.00000000000000711, 79.86467493626639680 ) ) ;
#38440=CARTESIAN_POINT ( 'NONE',  ( -11.85532105537472525, 31.00000000000000355, -20.54123584193516550 ) ) ;
#38442=CARTESIAN_POINT ( 'NONE',  ( -22.00000000000000000, 17.11489954122026447, 0.000000000000000000 ) ) ;
#38451=CARTESIAN_POINT ( 'NONE',  ( -86.05617919112455638, 31.00000000000000711, 49.70311056393224192 ) ) ;
#38454=CARTESIAN_POINT ( 'NONE',  ( 4.597210615070504325, 40.00000000000000000, -34.47704375835832025 ) ) ;
#38482=CARTESIAN_POINT ( 'NONE',  ( 54.55067978551168295, 31.00000000000000355, 18.62288743479739139 ) ) ;
#38490=CARTESIAN_POINT ( 'NONE',  ( 17.81064159970942384, 40.00000000000000000, 66.89829513328324140 ) ) ;
#38503=CARTESIAN_POINT ( 'NONE',  ( -51.86900026051868196, 31.00000000000000355, 45.50549606403863123 ) ) ;
#38506=EDGE_CURVE ( 'NONE', #26923, #42412, #28892, .T. ) ;
#38511=CARTESIAN_POINT ( 'NONE',  ( 53.86549405311983918, 31.00000000000000355, 70.40131829849023859 ) ) ;
#38512=CARTESIAN_POINT ( 'NONE',  ( 58.29702017945731995, 39.99999999999999289, 66.63806913872475945 ) ) ;
#38523=ORIENTED_EDGE ( 'NONE', *, *, #25433, .T. ) ;
#38540=CARTESIAN_POINT ( 'NONE',  ( 2.996940313443920978, 40.00000000000000000, -44.59688583547568896 ) ) ;
#38553=CARTESIAN_POINT ( 'NONE',  ( -2.781618486875174767, 31.00000000000000355, -42.39583333490362804 ) ) ;
#38557=CARTESIAN_POINT ( 'NONE',  ( 26.74431375183570481, 31.00000000000000355, -78.78324499025107741 ) ) ;
#38560=CARTESIAN_POINT ( 'NONE',  ( 56.43498182460272972, 31.00000000000000355, -7.339809665447901921 ) ) ;
#38561=CARTESIAN_POINT ( 'NONE',  ( -23.88228986782336349, 40.00000000000000000, -89.13686966975919290 ) ) ;
#38579=CARTESIAN_POINT ( 'NONE',  ( -4.417864660710832503, 40.00000000000000000, 67.60416666563759236 ) ) ;
#38610=CARTESIAN_POINT ( 'NONE',  ( 43.19851606872948935, 31.00000000000000355, 14.66122656362567689 ) ) ;
#38614=CARTESIAN_POINT ( 'NONE',  ( 16.30650823456882748, 40.00000000000000000, -60.90571087954511142 ) ) ;
#38628=CARTESIAN_POINT ( 'NONE',  ( 29.64712525329720449, 40.00000000000000000, -17.12831674356021239 ) ) ;
#38644=CARTESIAN_POINT ( 'NONE',  ( 86.24314314301659579, 31.00000000000000000, -11.24622374123920920 ) ) ;
#38651=CARTESIAN_POINT ( 'NONE',  ( 31.77777543000702565, 40.00000000000000000, 93.95825142774114624 ) ) ;
#38652=CARTESIAN_POINT ( 'NONE',  ( -1.974796425974089331, 31.00000000000000355, 29.60085432090884439 ) ) ;
#38656=CARTESIAN_POINT ( 'NONE',  ( -19.99999999999999645, 31.00000000000000355, 1.283214542831032867 ) ) ;
#38665=CARTESIAN_POINT ( 'NONE',  ( 42.89041025189590783, 31.00000000000000355, 86.97820559439793442 ) ) ;
#38670=CARTESIAN_POINT ( 'NONE',  ( -27.97094176822542977, 40.00000000000000000, 9.504947828999611659 ) ) ;
#38671=CARTESIAN_POINT ( 'NONE',  ( 15.66220904948252546, 40.00000000000000000, -31.63873590539992975 ) ) ;
#38680=ORIENTED_EDGE ( 'NONE', *, *, #3696, .T. ) ;
#38692=AXIS2_PLACEMENT_3D ( 'NONE', #12918, #27093, #23190 ) ;
#38701=CARTESIAN_POINT ( 'NONE',  ( 35.58199112953183629, 31.00000000000000355, 46.53705319858424616 ) ) ;
#38708=CARTESIAN_POINT ( 'NONE',  ( -71.90006454724937157, 40.00000000000000711, 4.599370544632132685 ) ) ;
#38718=CARTESIAN_POINT ( 'NONE',  ( -62.26029918285335896, 31.00000000000000711, 30.70375207684418228 ) ) ;
#38730=CARTESIAN_POINT ( 'NONE',  ( -11.85673204380701939, 31.00000000000000355, 89.11174773313419450 ) ) ;
#38732=CARTESIAN_POINT ( 'NONE',  ( 11.57239447660066567, 40.00000000000000000, 88.72710294830137912 ) ) ;
#38737=ORIENTED_EDGE ( 'NONE', *, *, #1361, .T. ) ;
#38749=EDGE_LOOP ( 'NONE', ( #31913, #8825, #29223, #32942 ) ) ;
#38750=CARTESIAN_POINT ( 'NONE',  ( 24.14050371820132668, 31.00000000000000355, 13.97356841391235704 ) ) ;
#38759=CARTESIAN_POINT ( 'NONE',  ( 22.78600399168703916, 40.00000000000000000, -39.30137845373389638 ) ) ;
#38771=CARTESIAN_POINT ( 'NONE',  ( 20.45440555730427690, 31.00000000000000355, -26.67302265141799467 ) ) ;
#38779=CARTESIAN_POINT ( 'NONE',  ( -22.78857244739539212, 31.00000000000000355, 85.10612709700112077 ) ) ;
#38782=CARTESIAN_POINT ( 'NONE',  ( 57.09498703527648900, 31.00000000000000355, 3.831922229400927637 ) ) ;
#38783=CARTESIAN_POINT ( 'NONE',  ( 70.70367055548476287, 39.99999999999999289, -62.02616482874480397 ) ) ;
#38800=CARTESIAN_POINT ( 'NONE',  ( -79.89583333417640176, 40.00000000000000711, 5.235987747608064957 ) ) ;
#38802=AXIS2_PLACEMENT_3D ( 'NONE', #33893, #6617, #707 ) ;
#38834=CARTESIAN_POINT ( 'NONE',  ( -60.10416666555506993, 31.00000000000000711, -3.926990808566252156 ) ) ;
#38839=CARTESIAN_POINT ( 'NONE',  ( 37.24516168167158270, 40.00000000000000000, 42.45166511289891531 ) ) ;
#38844=CARTESIAN_POINT ( 'NONE',  ( -19.47536345555549886, 31.00000000000000355, -6.605835105517199324 ) ) ;
#38849=CARTESIAN_POINT ( 'NONE',  ( 33.70925502316616473, 40.00000000000000000, 11.43906998022225707 ) ) ;
#38863=CARTESIAN_POINT ( 'NONE',  ( -73.09555549758189841, 31.00000000000000711, 35.91380138263622257 ) ) ;
#38871=CARTESIAN_POINT ( 'NONE',  ( 3.245924575715138705, 31.00000000000000355, -24.54795925723445649 ) ) ;
#38892=CARTESIAN_POINT ( 'NONE',  ( 14.71924655979513297, 40.00000000000000000, -29.87007926703815741 ) ) ;
#38893=CARTESIAN_POINT ( 'NONE',  ( 32.80084743084300669, 40.00000000000000000, 19.01436317119532760 ) ) ;
#38903=ORIENTED_EDGE ( 'NONE', *, *, #23994, .F. ) ;
#38911=CARTESIAN_POINT ( 'NONE',  ( -78.83182461418512332, 40.00000000000000711, -45.51551753872077910 ) ) ;
#38919=CARTESIAN_POINT ( 'NONE',  ( -40.56882557770292408, 31.00000000000000355, 31.01417895415301373 ) ) ;
#38924=CARTESIAN_POINT ( 'NONE',  ( -23.73339997550686675, 40.00000000000000000, -70.23208777907456124 ) ) ;
#38929=ORIENTED_EDGE ( 'NONE', *, *, #517, .T. ) ;
#38934=CARTESIAN_POINT ( 'NONE',  ( -45.35818215263140019, 31.00000000000000355, 51.72168634911185592 ) ) ;
#38945=DIRECTION ( 'NONE',  ( 0.000000000000000000, 0.000000000000000000, 1.000000000000000000 ) ) ;
#38946=CARTESIAN_POINT ( 'NONE',  ( -45.36921519482122278, 31.00000000000000711, 78.33339762288051134 ) ) ;
#38947=CARTESIAN_POINT ( 'NONE',  ( 83.51212062389942048, 39.99999999999999289, -48.08891344038907079 ) ) ;
#38961=CARTESIAN_POINT ( 'NONE',  ( 1.622176940739286310, 31.00000000000000355, -24.60292901074088334 ) ) ;
#38968=VERTEX_POINT ( 'NONE', #35314 ) ;
#38971=CARTESIAN_POINT ( 'NONE',  ( 45.11287655886649617, 40.00000000000000000, -12.00022417491798521 ) ) ;
#38982=CARTESIAN_POINT ( 'NONE',  ( -39.95047694894377344, 31.00000000000000355, -5.256506769647570465 ) ) ;
#38984=SURFACE_STYLE_USAGE ( .BOTH. , #32238 ) ;
#38988=CARTESIAN_POINT ( 'NONE',  ( 22.58587702529213104, 31.00000000000000355, 84.29678642628191199 ) ) ;
#38994=CARTESIAN_POINT ( 'NONE',  ( -41.78821403078461572, 31.00000000000000355, -47.79414628086201589 ) ) ;
#38995=CARTESIAN_POINT ( 'NONE',  ( -35.33737842959504860, 40.00000000000000000, 60.98257694382487415 ) ) ;
#38996=CARTESIAN_POINT ( 'NONE',  ( 72.43982367323130234, 39.99999999999999289, 63.53091779346544143 ) ) ;
#39007=CARTESIAN_POINT ( 'NONE',  ( 65.81435062899562638, 39.99999999999999289, 37.99825742656441463 ) ) ;
#39035=CARTESIAN_POINT ( 'NONE',  ( -40.54929543462775143, 31.00000000000000355, -46.21859917192507794 ) ) ;
#39041=CARTESIAN_POINT ( 'NONE',  ( 17.12248163736668261, 31.00000000000000355, 34.87662400048955647 ) ) ;
#39042=CARTESIAN_POINT ( 'NONE',  ( -9.469526743414824921, 40.00000000000000000, -71.82433816204535049 ) ) ;
#39053=CARTESIAN_POINT ( 'NONE',  ( 28.34477777927418529, 40.00000000000000000, 36.93558740410973229 ) ) ;
#39066=CARTESIAN_POINT ( 'NONE',  ( 11.20008397362390618, 31.00000000000000355, -84.14439686172904942 ) ) ;
#39087=CARTESIAN_POINT ( 'NONE',  ( -23.46968090759046888, 31.00000000000000355, -20.57717900685300449 ) ) ;
#39094=CARTESIAN_POINT ( 'NONE',  ( 19.70274684888802952, 40.00000000000000000, 17.27304525429847359 ) ) ;
#39095=CARTESIAN_POINT ( 'NONE',  ( 32.62694724487211317, 40.00000000000000000, -16.02036196159510339 ) ) ;
#39119=CARTESIAN_POINT ( 'NONE',  ( 90.64482129758324902, 39.99999999999999289, 30.77200948131585889 ) ) ;
#39126=CARTESIAN_POINT ( 'NONE',  ( 53.62204311759385433, 31.00000000000000355, -18.10832464707264577 ) ) ;
#39132=CARTESIAN_POINT ( 'NONE',  ( 30.38134496340388324, 40.00000000000000000, 61.85720693096894252 ) ) ;
#39142=CARTESIAN_POINT ( 'NONE',  ( 10.81967497908702214, 31.00000000000000355, -82.17651821321413763 ) ) ;
#39151=CARTESIAN_POINT ( 'NONE',  ( 87.78546986788515483, 31.00000000000000000, 43.41392487578124104 ) ) ;
#39152=CARTESIAN_POINT ( 'NONE',  ( 86.58052584568750376, 39.99999999999999289, -42.55516686010646765 ) ) ;
#39160=EDGE_CURVE ( 'NONE', #37436, #10195, #3498, .T. ) ;
#39170=CARTESIAN_POINT ( 'NONE',  ( -3.169834189307652927, 31.00000000000000355, -24.13593742708953016 ) ) ;
#39179=CARTESIAN_POINT ( 'NONE',  ( 42.86166521172830102, 40.00000000000000000, 21.22462828019262204 ) ) ;
#39189=CARTESIAN_POINT ( 'NONE',  ( -27.33276042269523387, 31.00000000000000355, -31.15086293565511966 ) ) ;
#39194=CARTESIAN_POINT ( 'NONE',  ( -29.64342647699677613, 31.00000000000000355, -87.27882330658468391 ) ) ;
#39197=CARTESIAN_POINT ( 'NONE',  ( 45.08926718328532246, 31.00000000000000355, 51.56349680124436219 ) ) ;
#39199=CARTESIAN_POINT ( 'NONE',  ( 45.08926718327026606, 40.00000000000000000, 51.56349680124436219 ) ) ;
#39209=CARTESIAN_POINT ( 'NONE',  ( -105.0363123600777442, 40.00000000000000000, -2.692529638013756887 ) ) ;
#39211=CARTESIAN_POINT ( 'NONE',  ( -66.92166868300088822, 40.00000000000000711, -22.71661802240650019 ) ) ;
#39216=ADVANCED_FACE ( 'NONE', ( #3378 ), #13248, .T. ) ;
#39221=CARTESIAN_POINT ( 'NONE',  ( -20.64238946400878305, 40.00000000000000000, 3.177240882809045708 ) ) ;
#39238=CARTESIAN_POINT ( 'NONE',  ( 54.85378563033546584, 31.00000000000000355, 7.219977902337870290 ) ) ;
#39243=CARTESIAN_POINT ( 'NONE',  ( -8.786317949316114095, 31.00000000000000355, -33.00646673688142840 ) ) ;
#39245=CARTESIAN_POINT ( 'NONE',  ( -34.23962737045593485, 40.00000000000000000, 59.30561363632230609 ) ) ;
#39252=CARTESIAN_POINT ( 'NONE',  ( -10.91816144241376563, 40.00000000000000000, -40.73603723627661566 ) ) ;
#39255=CARTESIAN_POINT ( 'NONE',  ( -101.9959696149863930, 31.00000000000000355, -0.1269066430507536924 ) ) ;
#39266=CARTESIAN_POINT ( 'NONE',  ( 68.41293481155882716, 31.00000000000000000, -52.34142988146868447 ) ) ;
#39284=CARTESIAN_POINT ( 'NONE',  ( 22.22924588317381023, 31.00000000000000355, -25.35314793696836588 ) ) ;
#39293=CARTESIAN_POINT ( 'NONE',  ( 31.10108666877329853, 40.00000000000000000, 17.95223046116557697 ) ) ;
#39295=CARTESIAN_POINT ( 'NONE',  ( -30.84436395684957333, 40.00000000000000000, -10.52363363425145337 ) ) ;
#39318=VECTOR ( 'NONE', #9263, 999.9999999999998863 ) ;
#39323=CARTESIAN_POINT ( 'NONE',  ( 17.81483206087466442, 31.00000000000000355, -52.17936214187551514 ) ) ;
#39332=CARTESIAN_POINT ( 'NONE',  ( -69.31868535678037802, 40.00000000000000711, 18.45717643660483986 ) ) ;
#39346=CARTESIAN_POINT ( 'NONE',  ( 48.66231590553977071, 31.00000000000000000, -55.48862040801125062 ) ) ;
#39349=DIRECTION ( 'NONE',  ( 0.000000000000000000, 1.000000000000000000, 0.000000000000000000 ) ) ;
#39357=CARTESIAN_POINT ( 'NONE',  ( 96.90013369365226481, 31.00000000000000000, -6.223598210838602540 ) ) ;
#39358=CARTESIAN_POINT ( 'NONE',  ( 30.72743980831338462, 40.00000000000000000, -90.12673907452091271 ) ) ;
#39366=ORIENTED_EDGE ( 'NONE', *, *, #26522, .T. ) ;
#39380=CARTESIAN_POINT ( 'NONE',  ( 3.245924575715138705, 31.00000000000000355, -24.54795925723445649 ) ) ;
#39389=CARTESIAN_POINT ( 'NONE',  ( 12.49611804805956439, 40.00000000000000000, 37.00809541493615740 ) ) ;
#39390=CARTESIAN_POINT ( 'NONE',  ( -101.1532682021072134, 17.11489954122026447, -3.256983028635321187 ) ) ;
#39404=CARTESIAN_POINT ( 'NONE',  ( -22.94860596549062848, 31.00000000000000355, -46.53072237555588231 ) ) ;
#39413=CARTESIAN_POINT ( 'NONE',  ( 61.87885091699251916, 31.00000000000000000, -70.55635664373320992 ) ) ;
#39416=CARTESIAN_POINT ( 'NONE',  ( 28.99662776679064891, 31.00000000000000355, -58.58186007941694129 ) ) ;
#39417=CARTESIAN_POINT ( 'NONE',  ( -4.113979049837106494, 40.00000000000000000, -64.40000927351898952 ) ) ;
#39419=CARTESIAN_POINT ( 'NONE',  ( -99.14707074559267141, 40.00000000000000711, 13.06922382031732610 ) ) ;
#39433=CARTESIAN_POINT ( 'NONE',  ( 50.46169669344906339, 40.00000000000000000, 57.51940134901310131 ) ) ;
#39440=VERTEX_POINT ( 'NONE', #20239 ) ;
#39463=CARTESIAN_POINT ( 'NONE',  ( -38.74991464700507748, 31.00000000000000355, 44.18781823130588293 ) ) ;
#39467=CARTESIAN_POINT ( 'NONE',  ( -31.89861325429239258, 31.00000000000000355, 2.042328591206914012 ) ) ;
#39468=CARTESIAN_POINT ( 'NONE',  ( 63.32575250126041055, 39.99999999999999289, 16.95471465585521997 ) ) ;
#39478=CARTESIAN_POINT ( 'NONE',  ( 26.55430347651023837, 40.00000000000000000, -34.62409890758566178 ) ) ;
#39490=EDGE_CURVE ( 'NONE', #36133, #5078, #25444, .T. ) ;
#39494=CARTESIAN_POINT ( 'NONE',  ( -80.50242771303932443, 31.00000000000000711, -46.62292012068298419 ) ) ;
#39502=APPLICATION_CONTEXT ( 'automotive_design' ) ;
#39510=CARTESIAN_POINT ( 'NONE',  ( -14.08558183832706234, 31.00000000000000355, -28.55406316770863739 ) ) ;
#39516=LINE ( 'NONE', #6571, #29936 ) ;
#39517=CARTESIAN_POINT ( 'NONE',  ( 16.30133787010129254, 40.00000000000000000, 33.04822796959624753 ) ) ;
#39519=CARTESIAN_POINT ( 'NONE',  ( -30.89738163651703928, 40.00000000000000000, 40.13100860032159289 ) ) ;
#39549=CARTESIAN_POINT ( 'NONE',  ( 34.31975892712151222, 31.00000000000000355, 59.64049725130579560 ) ) ;
#39557=CARTESIAN_POINT ( 'NONE',  ( -101.9959696149863788, 40.00000000000000711, -0.1269066430510139010 ) ) ;
#39560=CARTESIAN_POINT ( 'NONE',  ( -62.56443097449947288, 40.00000000000000000, -55.02758207457567607 ) ) ;
#39571=CARTESIAN_POINT ( 'NONE',  ( 5.072363130230502115, 31.00000000000000355, 77.39583333421907696 ) ) ;
#39582=CARTESIAN_POINT ( 'NONE',  ( 24.72345498302141920, 31.00000000000000355, -91.84610802666480822 ) ) ;
#39584=CARTESIAN_POINT ( 'NONE',  ( 77.87745995356456774, 39.99999999999999289, 59.89653754212418590 ) ) ;
#39597=CARTESIAN_POINT ( 'NONE',  ( -15.99999999999997691, 40.00000000000000000, 5.571627607371296764E-15 ) ) ;
#39602=CARTESIAN_POINT ( 'NONE',  ( -10.89792128226954127, 31.00000000000000355, -32.25956908330170592 ) ) ;
#39607=DIRECTION ( 'NONE',  ( 0.000000000000000000, 0.000000000000000000, 1.000000000000000000 ) ) ;
#39612=CARTESIAN_POINT ( 'NONE',  ( -13.02511903071888533, 40.00000000000000000, 48.29538318457647961 ) ) ;
#39623=CARTESIAN_POINT ( 'NONE',  ( -44.11856065373272173, 31.00000000000000355, -25.46949057303769948 ) ) ;
#39628=CARTESIAN_POINT ( 'NONE',  ( -90.10416666596678681, 31.00000000000000711, -5.890486217120279200 ) ) ;
#39632=CARTESIAN_POINT ( 'NONE',  ( -8.314562429035724733, 31.00000000000000355, -63.88718494334916187 ) ) ;
#39633=CARTESIAN_POINT ( 'NONE',  ( 66.75914267698914273, 39.99999999999999289, 8.899205196614580871 ) ) ;
#39643=DIRECTION ( 'NONE',  ( 0.000000000000000000, 0.000000000000000000, -1.000000000000000000 ) ) ;
#39647=CARTESIAN_POINT ( 'NONE',  ( -71.24862878704732339, 40.00000000000000711, 35.13526414049667324 ) ) ;
#39659=CARTESIAN_POINT ( 'NONE',  ( -19.99999999999999645, 40.00000000000000000, 0.000000000000000000 ) ) ;
#39672=CARTESIAN_POINT ( 'NONE',  ( -19.47536345555549886, 31.00000000000000355, -6.605835105517199324 ) ) ;
#39674=DIRECTION ( 'NONE',  ( 0.000000000000000000, 0.000000000000000000, -1.000000000000000000 ) ) ;
#39677=CARTESIAN_POINT ( 'NONE',  ( -46.87443272357899815, 31.00000000000000355, 35.96965017775951878 ) ) ;
#39678=VERTEX_POINT ( 'NONE', #39557 ) ;
#39679=CARTESIAN_POINT ( 'NONE',  ( -23.27229071023271700, 31.00000000000000355, 20.35677778009614869 ) ) ;
#39680=CARTESIAN_POINT ( 'NONE',  ( 32.44529481510334534, 40.00000000000000000, -65.82339768528792945 ) ) ;
#39685=CARTESIAN_POINT ( 'NONE',  ( 20.73284993368543638, 40.00000000000000000, 42.03655757353646294 ) ) ;
#39702=CARTESIAN_POINT ( 'NONE',  ( -89.42636861580037078, 31.00000000000000711, -24.07434901466544730 ) ) ;
#39719=CARTESIAN_POINT ( 'NONE',  ( 8.699408683037360035, 31.00000000000000355, 25.59862650653646909 ) ) ;
#39729=CARTESIAN_POINT ( 'NONE',  ( 35.10416666475790493, 40.00000000000000000, 2.290744634698880233 ) ) ;
#39730=CARTESIAN_POINT ( 'NONE',  ( 31.88898475262399401, 40.00000000000000000, 36.48290236124523744 ) ) ;
#39740=CARTESIAN_POINT ( 'NONE',  ( -30.61154013076160751, 40.00000000000002842, 25.77968906985393716 ) ) ;
#39745=ADVANCED_FACE ( 'NONE', ( #488 ), #10548, .T. ) ;
#39757=CARTESIAN_POINT ( 'NONE',  ( 30.38134496340387969, 31.00000000000000355, 61.85720693093856681 ) ) ;
#39766=CARTESIAN_POINT ( 'NONE',  ( 42.86165537668587433, 40.00000000000000000, -73.99543480067944756 ) ) ;
#39778=CARTESIAN_POINT ( 'NONE',  ( 74.72486387243833406, 31.00000000000000000, 9.837939412698395003 ) ) ;
#39780=CARTESIAN_POINT ( 'NONE',  ( -19.99999999999999645, 40.00000000000000000, 0.000000000000000000 ) ) ;
#39808=CARTESIAN_POINT ( 'NONE',  ( -24.93870012978733541, 31.00000000000000355, -21.94074674037795702 ) ) ;
#39816=CARTESIAN_POINT ( 'NONE',  ( 42.13926417418816328, 40.00000000000000000, -36.83769365845790134 ) ) ;
#39830=CARTESIAN_POINT ( 'NONE',  ( 44.91824650936478491, 31.00000000000000355, 5.910997147197376123 ) ) ;
#39833=B_SPLINE_SURFACE_WITH_KNOTS ( 'NONE', 1, 3, ( 
 ( #3353, #16721, #34121, #40865, #21080, #4658, #11019, #28250, #34331, #934, #37601, #21730, #41076, #11442, #25210, #1594, #14946, #41516, #7504, #4425, #4214, #31296, #14513, #24347, #11664, #11228, #14729, #17799, #41738, #28474, #34771, #1381, #34979, #27820, #18449, #5088, #14284, #20867, #11882, #38251, #31072, #27592, #28033, #41295, #18242, #31716, #15170, #7716, #17583, #25008, #8367, #24777, #38031, #1160, #8159, #1812, #24560, #37812, #30856, #21523, #7931, #4881, #31506, #21295, #34546, #18034, #25833, #36037, #39295, #32563, #12726, #42375, #8795, #16217, #12304, #15793, #19505, #9430, #35607, #29099, #25629, #12519, #38454, #41943, #35188, #38671, #29514, #28881, #16010, #5726, #22153, #2650, #39095, #9215, #26030, #21933, #22566, #2223, #2430, #5934, #29309, #5311, #38893, #35808, #19292, #42577, #6161, #42782, #25412, #12093, #42147, #22783, #35411, #12943, #5526, #18680, #32774, #2857, #9009, #15581, #8573, #2019, #28677, #31942, #18883, #32345, #32142, #22360, #15383, #19083, #7015, #6802, #17091, #23002, #458, #40381, #10073, #13379, #33630, #29955, #30602, #10301, #23645, #16434, #32981, #27117, #10517, #36903, #26892, #3062, #3507, #36246, #13819, #26671, #33852, #667, #23852, #19939, #20163, #13594, #6573, #39940, #19717, #20367, #29738, #221, #16884, #30166, #16670, #39730, #40162, #37117, #9657, #23418, #13165, #7225, #20581, #3940, #6369, #17325, #30380, #3712, #26248, #39519, #33208, #43010, #26458, #9857, #33422, #9, #36679, #23209, #36458, #3291, #14462, #17977, #31663, #1109, #14236, #31248, #24514, #7665, #10966, #1333, #24953, #21031, #11178, #14676, #27988, #20815, #14893, #34282, #21676, #38203, #27772, #28192, #34074, #37336, #4374, #41246, #37763, #11389, #30807, #883, #24298, #34720, #41029, #37978, #27540, #11612, #7882, #31458, #34932, #21240, #17748, #41462, #40814, #8319, #21469, #5041, #4833, #34493, #18401, #40590, #4158, #37556, #4604, #17533, #18190, #31019, #7450, #24723, #14028, #8104, #1545, #27323, #10728, #24068, #9760, #20058, #42481, #28419, #26143, #9322, #5838, #36360, #6059, #9555, #29210, #36574, #23315, #29631, #39417, #29865, #22679, #13277, #43126, #9117, #1759, #6698, #33096, #12626, #22470, #22910, #36149, #13066, #16559, #9966, #35711, #41693, #39633, #23114, #6269, #19616, #19194, #32883, #26571, #39199, #32677, #25741, #2962, #39843, #16325, #42905, #26368, #6472, #15118, #19830, #12423, #3183, #38995, #32462, #2550, #15916, #25938, #2757, #35931, #19411, #16119, #29419, #42685, #12834, #10186, #27430, #40050, #40489, #14136, #23535, #7340, #10627, #37226, #23746, #3616, #20701, #20923, #16779, #30495, #20268, #14349, #27659, #34177, #120, #11079, #37448, #33966, #782, #996, #27009, #40926, #7565, #4274, #13923, #37017, #7123, #40699, #24405, #574, #33740, #4054, #7779, #20478, #17645, #17429, #16986, #37658, #3828, #23959, #33325, #30909, #27220, #30707, #17210, #10852, #3408, #36803, #30067, #33531, #13488, #24183, #26778, #6906, #30271, #341, #13705, #40281, #10411, #4485, #41581, #28088, #28315, #31784, #15236, #31137, #21581, #8427, #21790, #25068, #31995, #12149, #7990, #24617, #24841, #5373, #37869, #25470, #21355, #1226, #15441, #28531, #34827, #41351, #41796, #27878, #11284, #38307, #34607, #15005, #4722, #18090, #35247, #1652, #1873, #11731, #11942, #17863, #38512, #18737, #4940, #8222, #25264, #38094, #38732, #5145, #18507, #31351, #41135, #21988, #2074, #8632, #35037, #1436, #28735, #14575, #41998, #18298, #21137, #34385, #14788, #11501, #31559, #2705, #35667, #42430, #32200, #22417, #9498, #29162, #26094, #12369, #29577, #25894, #6220, #13011, #12575, #5785, #2916, #25690, #42847, #39358, #26314, #22853, #9274, #32833, #35465, #28941, #38947, #39152, #42211, #36101, #9065, #2277, #19141, #16276, #32408, #19357, #23060, #19562, #39584, #9714, #8858, #2494, #5581, #22630, #15859, #35873, #22214, #6005, #16066, #32628, #18941, #15637, #29371, #42634, #12784, #24990, #15566, #32126, #11427, #4640, #8997, #35394, #1579, #24761, #28454 ),
 ( #22341, #34965, #22135, #8558, #18226, #25613, #21712, #25193, #28863, #18865, #1797, #38440, #5073, #21917, #18016, #8142, #1365, #4863, #38871, #38236, #25395, #15155, #31493, #12077, #35168, #5291, #5511, #31282, #18665, #11649, #11866, #15363, #41928, #14714, #18434, #31922, #2006, #28658, #42129, #28019, #34757, #21504, #8351, #2208, #14928, #41278, #28233, #38014, #12287, #38652, #31697, #41725, #8776, #41498, #9605, #32722, #36198, #39679, #13116, #2600, #39891, #2803, #3457, #20112, #39467, #10018, #15964, #19240, #29468, #42955, #6316, #9806, #12675, #25984, #6108, #16617, #26191, #19882, #39243, #36625, #22956, #13327, #16831, #19666, #16167, #23363, #9371, #33371, #3238, #6749, #29910, #32932, #30115, #22521, #29260, #22727, #3010, #42524, #43173, #35983, #32512, #19458, #171, #42729, #26414, #13538, #33151, #26619, #39041, #9166, #12885, #35753, #16377, #29682, #23160, #5884, #36409, #6520, #10463, #17918, #4540, #10906, #20758, #11127, #3882, #37707, #24454, #33580, #26832, #31193, #14401, #23797, #3663, #7393, #34018, #37503, #40978, #34437, #17036, #23589, #20972, #34227, #4106, #30754, #30324, #17477, #7827, #20528, #13971, #6959, #832, #21185, #14182, #24241, #27481, #17692, #1280, #40755, #40104, #27714, #4321, #10242, #7612, #30961, #36855, #27268, #20316, #1049, #40538, #396, #13760, #27062, #40330, #37067, #7172, #33793, #17268, #30549, #37277, #617, #10676, #24014, #8475, #28785, #8272, #1702, #37922, #21837, #25526, #1923, #41845, #35085, #5426, #32248, #15286, #12202, #15489, #8685, #35513, #28577, #22045, #42046, #15060, #14625, #5198, #28366, #8043, #18563, #21410, #34665, #35302, #4781, #31836, #14838, #11995, #25113, #21628, #11553, #5629, #41637, #34876, #11784, #25314, #38560, #18140, #38782, #4991, #22265, #8915, #38359, #18991, #31403, #1488, #18347, #18788, #32043, #2126, #28135, #41405, #24896, #27932, #41187, #11335, #38150, #24666, #31606, #19829, #9965, #32675, #9321, #29864, #32461, #26570, #9759, #13276, #23113, #26142, #3182, #28997, #35709, #15914, #42683, #5837, #36359, #29209, #38994, #2549, #16558, #35930, #6267, #20057, #39632, #6471, #33095, #2327, #42480, #42265, #39416, #22678, #19193, #43125, #6058, #9554, #12625, #36572, #23314, #29630, #22909, #39842, #19410, #6697, #15693, #9116, #12422, #25740, #22469, #25937, #39197, #36148, #19615, #13065, #2756, #16118, #29418, #12833, #32882, #2961, #16324, #42904, #26367, #40048, #34176, #4273, #17428, #33965, #10185, #10626, #119, #7564, #33739, #40925, #7778, #17644, #27008, #13922, #20700, #13704, #3826, #26777, #14135, #23534, #7338, #23958, #37225, #23745, #3615, #4053, #20922, #16778, #30494, #20267, #14347, #27658, #30908, #13487, #11078, #37447, #30706, #781, #995, #40280, #24404, #37657, #33324, #27219, #37016, #7122, #40698, #3407, #573, #17209, #27429, #30066, #20477, #36802, #10850, #16985, #6905, #40488, #24182, #33530, #30270, #340, #10410, #8221, #11730, #21136, #24616, #17861, #21354, #41997, #11500, #41795, #31558, #34606, #28530, #38306, #25067, #8631, #4484, #41580, #28087, #28313, #41134, #11941, #8426, #2073, #21789, #35036, #5144, #31994, #12148, #7989, #37868, #24839, #5372, #4721, #25469, #18089, #1225, #15440, #25263, #21580, #41350, #15235, #27877, #11283, #18506, #31350, #15004, #1435, #14787, #35245, #1651, #1872, #31782, #38511, #31136, #21987, #18736, #4939, #34826, #28734, #38093, #38730, #34384, #14574, #18297, #38946, #23059, #42429, #12783, #26514, #2915, #16275, #29576, #8857, #5784, #35464, #32626, #15858, #12368, #42846, #12574, #16065, #35666, #43072, #29806, #36099, #2704, #36308, #29160, #19776, #6425, #15636, #22213, #13225, #39582, #19140, #28940, #29370, #42633, #19561, #33040, #16503, #42209, #5580, #13009, #26313, #26093, #39357, #25689, #9496, #3125, #2493, #39151, #32199, #22852, #18940, #6219, #32832, #9713, #2276, #9064, #22416, #32407, #25893, #9273, #22629, #35872, #6003, #19356, #26949, #14289, #30439, #40224, #33272, #3769, #3358, #16725, #33912, #30015, #17150, #39997 ) ),
 .UNSPECIFIED., .F., .F., .F.,
 ( 2, 2 ),
 ( 4, 2, 2, 2, 2, 2, 2, 2, 2, 2, 2, 2, 2, 2, 2, 2, 2, 2, 2, 2, 2, 2, 2, 2, 2, 2, 2, 2, 2, 2, 2, 2, 2, 2, 2, 2, 2, 2, 2, 2, 2, 2, 2, 2, 2, 2, 2, 2, 2, 2, 2, 2, 2, 2, 2, 2, 2, 2, 2, 2, 2, 2, 2, 2, 2, 2, 2, 2, 2, 2, 2, 2, 2, 2, 2, 2, 2, 2, 2, 2, 2, 2, 2, 2, 2, 2, 2, 2, 2, 2, 2, 2, 2, 2, 2, 2, 2, 2, 2, 2, 2, 2, 2, 2, 2, 2, 2, 2, 2, 2, 2, 2, 2, 2, 2, 2, 2, 2, 2, 2, 2, 2, 2, 2, 2, 2, 2, 2, 2, 2, 2, 2, 2, 2, 2, 2, 2, 2, 2, 2, 2, 2, 2, 2, 2, 2, 2, 2, 2, 2, 2, 2, 2, 2, 2, 2, 2, 2, 2, 2, 2, 2, 2, 2, 2, 2, 2, 2, 2, 2, 2, 2, 2, 2, 2, 2, 2, 2, 2, 2, 2, 2, 2, 2, 2, 2, 2, 2, 2, 2, 2, 2, 2, 2, 2, 2, 2, 2, 2, 2, 2, 2, 2, 2, 2, 2, 2, 2, 2, 2, 2, 2, 2, 2, 2, 2, 2, 2, 2, 2, 2, 2, 2, 2, 2, 2, 2, 2, 2, 2, 2, 2, 2, 2, 2, 2, 2, 2, 2, 2, 2, 2, 2, 2, 2, 2, 2, 2, 2, 2, 2, 2, 2, 2, 2, 2, 4 ),
 ( 0.5000000000000002220, 0.9090909090909090606 ),
 ( 0.000000000000000000, 0.003906250000000000000, 0.007812500000000000000, 0.01171875000000000000, 0.01562500000000000000, 0.01953125000000000000, 0.02343750000000000000, 0.02734375000000000000, 0.03125000000000000000, 0.03515625000000000000, 0.03906250000000000000, 0.04296875000000000000, 0.04687500000000000000, 0.05078125000000000000, 0.05468750000000000000, 0.05859375000000000000, 0.06250000000000000000, 0.06640625000000000000, 0.07031250000000000000, 0.07421875000000000000, 0.07812500000000000000, 0.08203125000000000000, 0.08593750000000000000, 0.08984375000000000000, 0.09375000000000000000, 0.09765625000000000000, 0.1015625000000000000, 0.1054687500000000000, 0.1093750000000000000, 0.1132812500000000000, 0.1171875000000000000, 0.1210937500000000000, 0.1250000000000000000, 0.1289062500000000000, 0.1328125000000000000, 0.1367187500000000000, 0.1406250000000000000, 0.1445312500000000000, 0.1484375000000000000, 0.1523437500000000000, 0.1562500000000000000, 0.1601562500000000000, 0.1640625000000000000, 0.1679687500000000000, 0.1718750000000000000, 0.1757812500000000000, 0.1796875000000000000, 0.1835937500000000000, 0.1875000000000000000, 0.1914062500000000000, 0.1953125000000000000, 0.1992187500000000000, 0.2031250000000000000, 0.2070312500000000000, 0.2109375000000000000, 0.2148437500000000000, 0.2187500000000000000, 0.2226562500000000000, 0.2265625000000000000, 0.2304687500000000000, 0.2343750000000000000, 0.2382812500000000000, 0.2421875000000000000, 0.2460937500000000000, 0.2500000000000000000, 0.2539062500000000000, 0.2578125000000000000, 0.2617187500000000000, 0.2656250000000000000, 0.2695312500000000000, 0.2734375000000000000, 0.2773437500000000000, 0.2812500000000000000, 0.2851562500000000000, 0.2890625000000000000, 0.2929687500000000000, 0.2968750000000000000, 0.3007812500000000000, 0.3046875000000000000, 0.3085937500000000000, 0.3125000000000000000, 0.3164062500000000000, 0.3203125000000000000, 0.3242187500000000000, 0.3281250000000000000, 0.3320312500000000000, 0.3359375000000000000, 0.3398437500000000000, 0.3437500000000000000, 0.3476562500000000000, 0.3515625000000000000, 0.3554687500000000000, 0.3593750000000000000, 0.3632812500000000000, 0.3671875000000000000, 0.3710937500000000000, 0.3750000000000000000, 0.3789062500000000000, 0.3828125000000000000, 0.3867187500000000000, 0.3906250000000000000, 0.3945312500000000000, 0.3984375000000000000, 0.4023437500000000000, 0.4062500000000000000, 0.4101562500000000000, 0.4140625000000000000, 0.4179687500000000000, 0.4218750000000000000, 0.4257812500000000000, 0.4296875000000000000, 0.4335937500000000000, 0.4375000000000000000, 0.4414062500000000000, 0.4453125000000000000, 0.4492187500000000000, 0.4531250000000000000, 0.4570312500000000000, 0.4609375000000000000, 0.4648437500000000000, 0.4687500000000000000, 0.4726562500000000000, 0.4765625000000000000, 0.4804687500000000000, 0.4843750000000000000, 0.4882812500000000000, 0.4921875000000000000, 0.4960937500000000000, 0.5000000000000000000, 0.5039062500000000000, 0.5078125000000000000, 0.5117187500000000000, 0.5156250000000000000, 0.5195312500000000000, 0.5234375000000000000, 0.5273437500000000000, 0.5312500000000000000, 0.5351562500000000000, 0.5390625000000000000, 0.5429687500000000000, 0.5468750000000000000, 0.5507812500000000000, 0.5546875000000000000, 0.5585937500000000000, 0.5625000000000000000, 0.5664062500000000000, 0.5703125000000000000, 0.5742187500000000000, 0.5781250000000000000, 0.5820312500000000000, 0.5859375000000000000, 0.5898437500000000000, 0.5937500000000000000, 0.5976562500000000000, 0.6015625000000000000, 0.6054687500000000000, 0.6093750000000000000, 0.6132812500000000000, 0.6171875000000000000, 0.6210937500000000000, 0.6250000000000000000, 0.6289062500000000000, 0.6328125000000000000, 0.6367187500000000000, 0.6406250000000000000, 0.6445312500000000000, 0.6484375000000000000, 0.6523437500000000000, 0.6562500000000000000, 0.6601562500000000000, 0.6640625000000000000, 0.6679687500000000000, 0.6718750000000000000, 0.6757812500000000000, 0.6796875000000000000, 0.6835937500000000000, 0.6875000000000000000, 0.6914062500000000000, 0.6953125000000000000, 0.6992187500000000000, 0.7031250000000000000, 0.7070312500000000000, 0.7109375000000000000, 0.7148437500000000000, 0.7187500000000000000, 0.7226562500000000000, 0.7265625000000000000, 0.7304687500000000000, 0.7343750000000000000, 0.7382812500000000000, 0.7421875000000000000, 0.7460937500000000000, 0.7500000000000000000, 0.7539062500000000000, 0.7578125000000000000, 0.7617187500000000000, 0.7656250000000000000, 0.7695312500000000000, 0.7734375000000000000, 0.7773437500000000000, 0.7812500000000000000, 0.7851562500000000000, 0.7890625000000000000, 0.7929687500000000000, 0.7968750000000000000, 0.8007812500000000000, 0.8046875000000000000, 0.8085937500000000000, 0.8125000000000000000, 0.8164062500000000000, 0.8203125000000000000, 0.8242187500000000000, 0.8281250000000000000, 0.8320312500000000000, 0.8359375000000000000, 0.8398437500000000000, 0.8437500000000000000, 0.8476562500000000000, 0.8515625000000000000, 0.8554687500000000000, 0.8593750000000000000, 0.8632812500000000000, 0.8671875000000000000, 0.8710937500000000000, 0.8750000000000000000, 0.8789062500000000000, 0.8828125000000000000, 0.8867187500000000000, 0.8906250000000000000, 0.8945312500000000000, 0.8984375000000000000, 0.9023437500000000000, 0.9062500000000000000, 0.9101562500000000000, 0.9140625000000000000, 0.9179687500000000000, 0.9218750000000000000, 0.9257812500000000000, 0.9296875000000000000, 0.9335937500000000000, 0.9375000000000000000, 0.9414062500000000000, 0.9453125000000000000, 0.9492187500000000000, 0.9531250000000000000, 0.9570312500000000000, 0.9609375000000000000, 0.9648437500000000000, 0.9687500000000000000, 0.9726562500000000000, 0.9765625000000000000, 0.9804687500000000000, 0.9843750000000000000, 0.9882812500000000000, 0.9921875000000000000, 0.9960937500000000000, 1.000000000000000000 ),
 .UNSPECIFIED. ) ;
#39836=CARTESIAN_POINT ( 'NONE',  ( -94.39576909109665337, 31.00000000000000711, 32.06004391471374504 ) ) ;
#39842=CARTESIAN_POINT ( 'NONE',  ( 66.90003082756123831, 31.00000000000000000, -4.275635516647131595 ) ) ;
#39843=CARTESIAN_POINT ( 'NONE',  ( 22.12550800842195287, 40.00000000000000000, 65.48657384633656875 ) ) ;
#39857=CARTESIAN_POINT ( 'NONE',  ( 55.27058341129635721, 39.99999999999999289, -63.02248852588876105 ) ) ;
#39868=CARTESIAN_POINT ( 'NONE',  ( 16.96065435355295392, 40.00000000000000000, -19.31014141889295743 ) ) ;
#39886=CARTESIAN_POINT ( 'NONE',  ( -53.60515337853228601, 31.00000000000000355, -47.01024902908782366 ) ) ;
#39891=CARTESIAN_POINT ( 'NONE',  ( -28.12618851199096781, 31.00000000000000355, 13.81902982503210708 ) ) ;
#39894=CARTESIAN_POINT ( 'NONE',  ( -63.57631528421845957, 40.00000000000000711, -31.33741679916209222 ) ) ;
#39902=CARTESIAN_POINT ( 'NONE',  ( -40.10416666498607441, 40.00000000000000000, -2.617993869485698344 ) ) ;
#39915=CARTESIAN_POINT ( 'NONE',  ( 5.735608225908778834, 31.00000000000000355, 89.40012361740336644 ) ) ;
#39927=DIRECTION ( 'NONE',  ( 0.000000000000000000, 0.000000000000000000, -1.000000000000000000 ) ) ;
#39931=CARTESIAN_POINT ( 'NONE',  ( 4.274771203358150196, 31.00000000000000355, -32.49882260841580006 ) ) ;
#39939=CARTESIAN_POINT ( 'NONE',  ( -35.29531037056285214, 40.00000000000000000, 17.40921588598563119 ) ) ;
#39940=CARTESIAN_POINT ( 'NONE',  ( 47.09643503918425012, 40.00000000000000000, 3.164684800459844904 ) ) ;
#39967=CARTESIAN_POINT ( 'NONE',  ( 43.45541166190962912, 31.00000000000000355, -49.38773770141698805 ) ) ;
#39975=CARTESIAN_POINT ( 'NONE',  ( -35.65230965300054322, 40.00000000000000000, 72.05959145982365044 ) ) ;
#39986=CARTESIAN_POINT ( 'NONE',  ( 34.02738612458995959, 31.00000000000000355, 69.00154638599002510 ) ) ;
#39997=CARTESIAN_POINT ( 'NONE',  ( -101.9959696149863646, 31.00000000000000711, -0.1269066430510134569 ) ) ;
#40018=CARTESIAN_POINT ( 'NONE',  ( -24.64063138600606351, 31.00000000000000355, 18.85097431369995746 ) ) ;
#40028=CARTESIAN_POINT ( 'NONE',  ( 54.55067978551168295, 40.00000000000000000, 18.62288743479739495 ) ) ;
#40037=CARTESIAN_POINT ( 'NONE',  ( -24.21661388771557100, 31.00000000000000355, 41.94898165618241137 ) ) ;
#40044=CARTESIAN_POINT ( 'NONE',  ( 11.68784703496123711, 40.00000000000000000, -20.25319168173327355 ) ) ;
#40048=CARTESIAN_POINT ( 'NONE',  ( -35.33737842959504150, 31.00000000000000355, 60.98257694382487415 ) ) ;
#40050=CARTESIAN_POINT ( 'NONE',  ( -68.78002826189113250, 40.00000000000000711, -23.46745878763887916 ) ) ;
#40052=ADVANCED_FACE ( 'NONE', ( #42559 ), #22339, .F. ) ;
#40056=DIRECTION ( 'NONE',  ( 0.000000000000000000, 0.000000000000000000, -1.000000000000000000 ) ) ;
#40064=CARTESIAN_POINT ( 'NONE',  ( -10.77850749866037816, 40.00000000000000000, -81.75987728344749428 ) ) ;
#40076=DIRECTION ( 'NONE',  ( -0.000000000000000000, -1.060184893785364939E-15, -1.000000000000000000 ) ) ;
#40078=ORIENTED_EDGE ( 'NONE', *, *, #17270, .T. ) ;
#40079=CARTESIAN_POINT ( 'NONE',  ( -18.31940394017777862, 40.00000000000000000, -14.05611420671344014 ) ) ;
#40094=CARTESIAN_POINT ( 'NONE',  ( -18.63466726053507472, 31.00000000000000355, -9.179856479542758407 ) ) ;
#40101=CARTESIAN_POINT ( 'NONE',  ( 59.08215048199704711, 31.00000000000000000, 29.12166076728773589 ) ) ;
#40104=CARTESIAN_POINT ( 'NONE',  ( 45.11287655886648906, 31.00000000000000355, -12.00022417491544324 ) ) ;
#40105=CARTESIAN_POINT ( 'NONE',  ( -34.66105084696506822, 40.00000000000000000, 70.31756248751102589 ) ) ;
#40121=CARTESIAN_POINT ( 'NONE',  ( 28.40420691229738281, 40.00000000000000000, 49.17333623205379922 ) ) ;
#40133=CARTESIAN_POINT ( 'NONE',  ( 63.29164158772582027, 31.00000000000000000, -71.97807289022838972 ) ) ;
#40141=AXIS2_PLACEMENT_3D ( 'NONE', #21823, #31593, #27916 ) ;
#40154=CARTESIAN_POINT ( 'NONE',  ( -27.33276042269523387, 31.00000000000000355, -31.15086293565511966 ) ) ;
#40161=CARTESIAN_POINT ( 'NONE',  ( -44.11856065373272173, 40.00000000000000000, -25.46949057303769948 ) ) ;
#40162=CARTESIAN_POINT ( 'NONE',  ( 29.49207856986237530, 40.00000000000000000, 38.57905506995709288 ) ) ;
#40172=CARTESIAN_POINT ( 'NONE',  ( -19.76500330823589735, 40.00000000000000000, -5.286999072153966139 ) ) ;
#40192=CARTESIAN_POINT ( 'NONE',  ( 51.26988013555838819, 31.00000000000000355, 45.10883117380814866 ) ) ;
#40203=CARTESIAN_POINT ( 'NONE',  ( 77.59064570039033981, 39.99999999999999289, -38.12735739512951483 ) ) ;
#40209=DIRECTION ( 'NONE',  ( 0.000000000000000000, 1.000000000000000000, -1.060184893785364939E-15 ) ) ;
#40217=CARTESIAN_POINT ( 'NONE',  ( -6.054110834496889026, 31.00000000000000355, -92.39583333400220511 ) ) ;
#40219=ORIENTED_EDGE ( 'NONE', *, *, #23937, .T. ) ;
#40224=CARTESIAN_POINT ( 'NONE',  ( -76.05825820879897492, 31.00000000000000711, 66.55365856249082412 ) ) ;
#40247=CARTESIAN_POINT ( 'NONE',  ( -7.793954689941437586, 31.00000000000000355, 28.94896179907300748 ) ) ;
#40257=CARTESIAN_POINT ( 'NONE',  ( 6.367266499441480931, 40.00000000000000000, 48.98256792610028754 ) ) ;
#40258=LINE ( 'NONE', #16758, #41677 ) ;
#40267=CARTESIAN_POINT ( 'NONE',  ( 21.71086051706764763, 31.00000000000000355, -37.60982366119799991 ) ) ;
#40274=CARTESIAN_POINT ( 'NONE',  ( -20.10416666680962550, 40.00000000000000000, -1.308996940106889273 ) ) ;
#40280=CARTESIAN_POINT ( 'NONE',  ( 74.15939217261870908, 31.00000000000000000, -19.75058139460982432 ) ) ;
#40281=CARTESIAN_POINT ( 'NONE',  ( -81.90010630563853056, 40.00000000000000711, 5.248159452637418454 ) ) ;
#40293=CARTESIAN_POINT ( 'NONE',  ( -26.42126989340051324, 40.00000000000000000, -77.78956226056263290 ) ) ;
#40305=VERTEX_POINT ( 'NONE', #11370 ) ;
#40308=CARTESIAN_POINT ( 'NONE',  ( 22.27703560431449148, 40.00000000000000000, 17.12883495622503816 ) ) ;
#40318=CARTESIAN_POINT ( 'NONE',  ( -19.99999999999999645, 31.00000000000000355, -7.355690625810191807E-15 ) ) ;
#40326=CARTESIAN_POINT ( 'NONE',  ( 17.40022565512299479, 31.00000000000000355, 64.93645345284011228 ) ) ;
#40330=CARTESIAN_POINT ( 'NONE',  ( 21.53706125532763593, 31.00000000000000355, 43.87245753946415761 ) ) ;
#40331=CARTESIAN_POINT ( 'NONE',  ( 5.072363130230502115, 40.00000000000000000, 77.39583333421907696 ) ) ;
#40341=CARTESIAN_POINT ( 'NONE',  ( -51.34291522965900612, 40.00000000000000000, 29.65708359768123970 ) ) ;
#40355=CARTESIAN_POINT ( 'NONE',  ( 12.87762912550514827, 31.00000000000000355, 98.66289914823325091 ) ) ;
#40374=CARTESIAN_POINT ( 'NONE',  ( -12.24460912605626106, 31.00000000000000355, 36.08157028455360660 ) ) ;
#40380=CARTESIAN_POINT ( 'NONE',  ( 43.19851606872948935, 40.00000000000000000, 14.66122656362567689 ) ) ;
#40381=CARTESIAN_POINT ( 'NONE',  ( -34.17541447290003020, 40.00000000000000000, -26.31327426976606887 ) ) ;
#40391=CARTESIAN_POINT ( 'NONE',  ( -17.40445659762299968, 40.00000000000000000, 22.69748452323785060 ) ) ;
#40399=CARTESIAN_POINT ( 'NONE',  ( -99.91857577502598531, 17.11489954122026447, -1.280628618496984839 ) ) ;
#40407=CARTESIAN_POINT ( 'NONE',  ( 4.329677741076777053, 31.00000000000000355, -64.59417075179258916 ) ) ;
#40414=CARTESIAN_POINT ( 'NONE',  ( -65.95487968126425926, 40.00000000000000711, -50.74205456615700882 ) ) ;
#40428=CARTESIAN_POINT ( 'NONE',  ( -66.93673649651354651, 31.00000000000000711, 58.72203107584222437 ) ) ;
#40447=VECTOR ( 'NONE', #3324, 999.9999999999998863 ) ;
#40460=CARTESIAN_POINT ( 'NONE',  ( -15.23573235977617379, 31.00000000000000355, 26.30445775087292404 ) ) ;
#40466=CARTESIAN_POINT ( 'NONE',  ( -39.97893566998936876, 40.00000000000000000, -35.18630237794886995 ) ) ;
#40477=CARTESIAN_POINT ( 'NONE',  ( 25.16436199730139123, 31.00000000000000355, 51.02488717759543135 ) ) ;
#40483=CARTESIAN_POINT ( 'NONE',  ( 42.89041025189590783, 31.00000000000000355, 86.97820559439793442 ) ) ;
#40488=CARTESIAN_POINT ( 'NONE',  ( 5.085823974618866039, 31.00000000000000355, 79.40009828669005287 ) ) ;
#40489=CARTESIAN_POINT ( 'NONE',  ( -65.32047834219908111, 40.00000000000000711, -32.32491738442255524 ) ) ;
#40502=VERTEX_POINT ( 'NONE', #1958 ) ;
#40504=CARTESIAN_POINT ( 'NONE',  ( -80.23695839127151430, 40.00000000000000711, 39.56677620416681407 ) ) ;
#40507=VECTOR ( 'NONE', #15032, 1000.000000000000000 ) ;
#40519=CARTESIAN_POINT ( 'NONE',  ( -22.06642698273767067, 40.00000000000000000, -2.901557744773887393 ) ) ;
#40528=CARTESIAN_POINT ( 'NONE',  ( -17.40445659762299968, 31.00000000000000355, 22.69748452323785060 ) ) ;
#40534=CARTESIAN_POINT ( 'NONE',  ( 32.44529481510334534, 31.00000000000000355, -65.82339768528792945 ) ) ;
#40538=CARTESIAN_POINT ( 'NONE',  ( 36.21668514974006570, 31.00000000000000355, 31.87730689759005287 ) ) ;
#40541=CARTESIAN_POINT ( 'NONE',  ( -10.77850749866037816, 40.00000000000000000, -81.75987728344749428 ) ) ;
#40552=CARTESIAN_POINT ( 'NONE',  ( 32.65420139560029611, 40.00000000000000000, -42.57517516360295673 ) ) ;
#40570=DIRECTION ( 'NONE',  ( 0.000000000000000000, 1.000000000000000000, 0.000000000000000000 ) ) ;
#40578=LINE ( 'NONE', #37541, #1231 ) ;
#40582=CARTESIAN_POINT ( 'NONE',  ( 13.85568741775851542, 31.00000000000000355, -40.82620080729295609 ) ) ;
#40588=CARTESIAN_POINT ( 'NONE',  ( -44.28363997456384737, 40.00000000000000000, 21.84072794957603492 ) ) ;
#40590=CARTESIAN_POINT ( 'NONE',  ( -15.62887661519555493, 40.00000000000000000, 57.97203279869352599 ) ) ;
#40598=CARTESIAN_POINT ( 'NONE',  ( 24.21999397792122366, 40.00000000000000000, 8.216913396989165008 ) ) ;
#40613=CARTESIAN_POINT ( 'NONE',  ( 46.16409756963976463, 31.00000000000000355, -59.99419878592187416 ) ) ;
#40621=CARTESIAN_POINT ( 'NONE',  ( 12.51314706078825090, 40.00000000000000000, -94.07914177280382262 ) ) ;
#40632=STYLED_ITEM ( 'NONE', ( #6049 ), #42324 ) ;
#40634=CARTESIAN_POINT ( 'NONE',  ( 50.95389515256417923, 31.00000000000000355, -66.42840393140320998 ) ) ;
#40656=ORIENTED_EDGE ( 'NONE', *, *, #5408, .F. ) ;
#40666=CARTESIAN_POINT ( 'NONE',  ( 41.46880187713386334, 31.00000000000000355, 24.04226233541373858 ) ) ;
#40671=ORIENTED_EDGE ( 'NONE', *, *, #1361, .F. ) ;
#40673=CARTESIAN_POINT ( 'NONE',  ( -41.78821403078462282, 40.00000000000000000, -47.79414628086202299 ) ) ;
#40675=EDGE_CURVE ( 'NONE', #16446, #11466, #27253, .T. ) ;
#40687=CARTESIAN_POINT ( 'NONE',  ( -58.48566925783705983, 31.00000000000000711, -15.65830181327787862 ) ) ;
#40693=CARTESIAN_POINT ( 'NONE',  ( -5.732510072307491988, 40.00000000000000000, -21.37570426403446078 ) ) ;
#40698=CARTESIAN_POINT ( 'NONE',  ( 69.81317433577432041, 31.00000000000000000, 34.54326205989952570 ) ) ;
#40699=CARTESIAN_POINT ( 'NONE',  ( 76.69346925290108175, 39.99999999999999289, 10.21457306974340007 ) ) ;
#40718=CARTESIAN_POINT ( 'NONE',  ( -49.69442049507403425, 40.00000000000000000, -64.76435429890716478 ) ) ;
#40728=CARTESIAN_POINT ( 'NONE',  ( 12.70938237924789860, 40.00000000000000000, -21.97768283340562689 ) ) ;
#40729=DIRECTION ( 'NONE',  ( 0.000000000000000000, 1.541976423090494844E-15, 1.000000000000000000 ) ) ;
#40744=CARTESIAN_POINT ( 'NONE',  ( -3.620280825866593055, 31.00000000000000355, 27.53105304817175636 ) ) ;
#40752=CARTESIAN_POINT ( 'NONE',  ( -18.69663849766352826, 31.00000000000000355, -69.77653669617104981 ) ) ;
#40755=CARTESIAN_POINT ( 'NONE',  ( 44.12914893500597202, 31.00000000000000355, -14.89880614700436112 ) ) ;
#40756=CARTESIAN_POINT ( 'NONE',  ( 50.95389515256417923, 40.00000000000000000, -66.42840393140320998 ) ) ;
#40768=CARTESIAN_POINT ( 'NONE',  ( -31.39472673864601049, 40.00000000000000000, -40.91112553188754930 ) ) ;
#40784=CARTESIAN_POINT ( 'NONE',  ( -101.9959696149863930, 31.00000000000000355, -0.1269066430507536924 ) ) ;
#40801=CARTESIAN_POINT ( 'NONE',  ( 44.50160557815096496, 31.00000000000000355, -5.869829666507492050 ) ) ;
#40805=DIRECTION ( 'NONE',  ( 1.541976423090495042E-15, -1.000000000000000000, 4.818676322157797005E-17 ) ) ;
#40813=CARTESIAN_POINT ( 'NONE',  ( -50.10416666532988472, 40.00000000000000000, -3.272492339034341224 ) ) ;
#40814=CARTESIAN_POINT ( 'NONE',  ( 25.95756378415974908, 40.00000000000000000, 52.86556711864420066 ) ) ;
#40821=CARTESIAN_POINT ( 'NONE',  ( -7.088330391075835735, 40.00000000000000000, -20.85399598300688595 ) ) ;
#40825=ORIENTED_EDGE ( 'NONE', *, *, #23817, .T. ) ;
#40827=DIRECTION ( 'NONE',  ( 0.000000000000000000, 1.000000000000000000, 0.000000000000000000 ) ) ;
#40839=CARTESIAN_POINT ( 'NONE',  ( -32.59403919554602425, 31.00000000000000355, -66.35267222981636337 ) ) ;
#40849=CARTESIAN_POINT ( 'NONE',  ( 94.26586287999622016, 39.99999999999999289, 25.37251369638877563 ) ) ;
#40860=CARTESIAN_POINT ( 'NONE',  ( -77.37786320076959612, 31.00000000000000711, 44.69160382239309115 ) ) ;
#40865=CARTESIAN_POINT ( 'NONE',  ( -21.70016380022027391, 40.00000000000000000, -5.809120511592388958 ) ) ;
#40892=CARTESIAN_POINT ( 'NONE',  ( 34.59698569360211451, 31.00000000000000355, -30.23997570423561498 ) ) ;
#40893=CARTESIAN_POINT ( 'NONE',  ( -22.00000000000000711, 40.00000000000000000, 0.000000000000000000 ) ) ;
#40900=CARTESIAN_POINT ( 'NONE',  ( 21.04585062969761822, 40.00000000000000000, -61.66509230325024760 ) ) ;
#40909=SHAPE_REPRESENTATION_RELATIONSHIP ( 'NONE' , 'NONE' ,  #41895, #31788 ) ;
#40915=CARTESIAN_POINT ( 'NONE',  ( -57.43240763726046794, 31.00000000000000355, -19.49446143887317717 ) ) ;
#40920=CARTESIAN_POINT ( 'NONE',  ( -17.40445659762299968, 40.00000000000000000, 22.69748452323785060 ) ) ;
#40925=CARTESIAN_POINT ( 'NONE',  ( -71.90006454728114704, 31.00000000000000711, 4.599370544632132685 ) ) ;
#40926=CARTESIAN_POINT ( 'NONE',  ( 68.60033760563641181, 39.99999999999999289, -33.70054013428169526 ) ) ;
#40945=CARTESIAN_POINT ( 'NONE',  ( 31.25450476884064699, 40.00000000000000000, 92.02345382966369414 ) ) ;
#40954=CARTESIAN_POINT ( 'NONE',  ( -30.58448433907587827, 40.00000000000000000, 8.146263651249089577 ) ) ;
#40969=CARTESIAN_POINT ( 'NONE',  ( 5.935205493550105516, 31.00000000000000355, -22.18504493031268865 ) ) ;
#40976=CARTESIAN_POINT ( 'NONE',  ( 5.072363130230502115, 31.00000000000000355, 77.39583333421907696 ) ) ;
#40978=CARTESIAN_POINT ( 'NONE',  ( -32.45554871466278968, 31.00000000000000355, -28.56710966684966380 ) ) ;
#40979=CARTESIAN_POINT ( 'NONE',  ( -77.84600223180727596, 40.00000000000000711, -20.84395318355897686 ) ) ;
#40995=CARTESIAN_POINT ( 'NONE',  ( -16.75480014238754478, 40.00000000000000000, -49.32177912249007790 ) ) ;
#41021=CARTESIAN_POINT ( 'NONE',  ( 18.38119342899891961, 31.00000000000000355, 31.81670425098764099 ) ) ;
#41028=CARTESIAN_POINT ( 'NONE',  ( 23.39270017067629936, 40.00000000000000000, 40.49502024156475244 ) ) ;
#41029=CARTESIAN_POINT ( 'NONE',  ( 56.82522199879618086, 40.00000000000000000, 7.581518937762242949 ) ) ;
#41038=CARTESIAN_POINT ( 'NONE',  ( -18.92511213055653130, 40.00000000000000000, 21.58621387822740090 ) ) ;
#41039=VERTEX_POINT ( 'NONE', #15833 ) ;
#41053=CARTESIAN_POINT ( 'NONE',  ( 72.60479858918232310, 31.00000000000000000, -24.53750584076950503 ) ) ;
#41060=CARTESIAN_POINT ( 'NONE',  ( -24.28006566513952791, 40.00000000000000000, -91.10131089348455191 ) ) ;
#41073=CARTESIAN_POINT ( 'NONE',  ( 22.58587702529213104, 31.00000000000000355, 84.29678642628191199 ) ) ;
#41076=CARTESIAN_POINT ( 'NONE',  ( -10.52919346384764054, 40.00000000000000000, -21.36894910329525743 ) ) ;
#41103=CARTESIAN_POINT ( 'NONE',  ( -41.92568936860566708, 31.00000000000000355, -5.596851440150872214 ) ) ;
#41110=CARTESIAN_POINT ( 'NONE',  ( -55.11358496761538106, 40.00000000000000711, 27.06326608206703099 ) ) ;
#41122=CARTESIAN_POINT ( 'NONE',  ( -35.70415035507907930, 31.00000000000000355, 46.55071329160319493 ) ) ;
#41124=PLANE ( 'NONE',  #29552 ) ;
#41128=CARTESIAN_POINT ( 'NONE',  ( -20.72449291656876369, 40.00000000000000000, -23.61699481730619610 ) ) ;
#41134=CARTESIAN_POINT ( 'NONE',  ( -54.99468034530342919, 31.00000000000000355, -62.86974495748531666 ) ) ;
#41135=CARTESIAN_POINT ( 'NONE',  ( -23.42519174997118014, 40.00000000000000000, 87.00664592748896098 ) ) ;
#41150=CARTESIAN_POINT ( 'NONE',  ( 84.73112319332513209, 39.99999999999999289, -41.78253223598262167 ) ) ;
#41163=CARTESIAN_POINT ( 'NONE',  ( -20.36888183406675168, 40.00000000000000000, -26.63352584488937325 ) ) ;
#41177=CARTESIAN_POINT ( 'NONE',  ( 24.89583333603155069, 31.00000000000000355, -1.636246165087041016 ) ) ;
#41184=CARTESIAN_POINT ( 'NONE',  ( -10.77850749866037816, 31.00000000000000355, -81.75987728344749428 ) ) ;
#41187=CARTESIAN_POINT ( 'NONE',  ( -3.998040010416403334, 31.00000000000000355, 59.59469406578620720 ) ) ;
#41188=CARTESIAN_POINT ( 'NONE',  ( -45.94448050778635917, 40.00000000000000000, -79.54744219826071117 ) ) ;
#41202=CARTESIAN_POINT ( 'NONE',  ( 57.76613438074698337, 39.99999999999999289, -28.48799604501563110 ) ) ;
#41216=CARTESIAN_POINT ( 'NONE',  ( -80.34276469477588023, 31.00000000000000711, 61.48650092630385444 ) ) ;
#41233=DIRECTION ( 'NONE',  ( 0.000000000000000000, 1.000000000000000000, 0.000000000000000000 ) ) ;
#41237=CARTESIAN_POINT ( 'NONE',  ( 47.00375723443311671, 31.00000000000000355, -27.15133022689256137 ) ) ;
#41245=CARTESIAN_POINT ( 'NONE',  ( 50.84997085138504502, 39.99999999999999289, -39.01959913716785167 ) ) ;
#41246=CARTESIAN_POINT ( 'NONE',  ( 48.78760054484346398, 40.00000000000000000, -28.06521077754944926 ) ) ;
#41254=CARTESIAN_POINT ( 'NONE',  ( 27.23661496637203427, 40.00000000000000000, 23.88131275951389654 ) ) ;
#41270=CARTESIAN_POINT ( 'NONE',  ( -67.85934734803990409, 31.00000000000000711, 22.92939687791763248 ) ) ;
#41277=CARTESIAN_POINT ( 'NONE',  ( 30.72743980831338462, 40.00000000000000000, -90.12673907452091271 ) ) ;
#41278=CARTESIAN_POINT ( 'NONE',  ( 9.304442065603227618, 31.00000000000000355, 27.50946418541002458 ) ) ;
#41291=CARTESIAN_POINT ( 'NONE',  ( -49.27414759474276451, 31.00000000000000711, 85.34056160678568403 ) ) ;
#41295=CARTESIAN_POINT ( 'NONE',  ( 14.33709021557830887, 40.00000000000000000, 24.89380824183666618 ) ) ;
#41297=ORIENTED_EDGE ( 'NONE', *, *, #20424, .T. ) ;
#41311=ORIENTED_EDGE ( 'NONE', *, *, #38389, .T. ) ;
#41320=CARTESIAN_POINT ( 'NONE',  ( -40.32452739092001792, 31.00000000000000355, -13.76986825753265897 ) ) ;
#41328=CARTESIAN_POINT ( 'NONE',  ( 40.05902963217418744, 40.00000000000000000, -52.04757428485088866 ) ) ;
#41331=CYLINDRICAL_SURFACE ( 'NONE', #18646, 4.500000000000000888 ) ;
#41332=ORIENTED_EDGE ( 'NONE', *, *, #32426, .F. ) ;
#41339=CARTESIAN_POINT ( 'NONE',  ( 55.68207322489292466, 31.00000000000000000, -32.16283696845439266 ) ) ;
#41350=CARTESIAN_POINT ( 'NONE',  ( 82.09539989324809994, 31.00000000000000000, -27.75477508811727390 ) ) ;
#41351=CARTESIAN_POINT ( 'NONE',  ( 68.41293481152064260, 39.99999999999999289, -52.34142988144959219 ) ) ;
#41366=CARTESIAN_POINT ( 'NONE',  ( 74.70319961851696178, 39.99999999999999289, -57.31929289364909152 ) ) ;
#41378=DIRECTION ( 'NONE',  ( 0.000000000000000000, 1.000000000000000000, -1.060184893785364939E-15 ) ) ;
#41381=CARTESIAN_POINT ( 'NONE',  ( 21.72498709343026846, 40.00000000000000000, -28.22316639787646864 ) ) ;
#41394=CARTESIAN_POINT ( 'NONE',  ( -29.59829689555773058, 31.00000000000000355, 3.906358533625565954 ) ) ;
#41401=CARTESIAN_POINT ( 'NONE',  ( -64.44063486737354651, 31.00000000000000711, -49.42892067282641477 ) ) ;
#41405=CARTESIAN_POINT ( 'NONE',  ( 15.22596115864829791, 31.00000000000000355, 57.21640888978779316 ) ) ;
#41408=CARTESIAN_POINT ( 'NONE',  ( -28.35539204363714205, 40.00000000000000000, 83.52787551312086123 ) ) ;
#41420=CARTESIAN_POINT ( 'NONE',  ( -60.10416666555506993, 40.00000000000000711, -3.926990808566252156 ) ) ;
#41423=ORIENTED_EDGE ( 'NONE', *, *, #11186, .F. ) ;
#41451=CARTESIAN_POINT ( 'NONE',  ( 3.108867721649529958, 31.00000000000000355, 47.39583333474234905 ) ) ;
#41460=CARTESIAN_POINT ( 'NONE',  ( -56.43872490705654599, 40.00000000000000711, 19.17141758012168751 ) ) ;
#41462=CARTESIAN_POINT ( 'NONE',  ( 29.31577600748121881, 40.00000000000000000, 50.95836110724019363 ) ) ;
#41470=CARTESIAN_POINT ( 'NONE',  ( 10.28773449565296083, 31.00000000000000355, -20.88174966193524895 ) ) ;
#41472=CARTESIAN_POINT ( 'NONE',  ( 9.621748599878955588, 40.00000000000000000, 35.89595399306684698 ) ) ;
#41487=CARTESIAN_POINT ( 'NONE',  ( -43.11175393642376008, 31.00000000000000355, 56.02072642018850246 ) ) ;
#41497=CARTESIAN_POINT ( 'NONE',  ( 96.56285295106285105, 39.99999999999999289, 12.84127866192819312 ) ) ;
#41498=CARTESIAN_POINT ( 'NONE',  ( -13.43146050690766380, 31.00000000000000355, 27.15249184975281693 ) ) ;
#41513=CARTESIAN_POINT ( 'NONE',  ( 61.87885091699251916, 31.00000000000000000, -70.55635664373320992 ) ) ;
#41516=CARTESIAN_POINT ( 'NONE',  ( 1.622176940739286310, 40.00000000000000000, -24.60292901074089045 ) ) ;
#41550=CARTESIAN_POINT ( 'NONE',  ( 2.511863649308172519, 31.00000000000000355, 39.39933062586388957 ) ) ;
#41556=CARTESIAN_POINT ( 'NONE',  ( -15.99999999999997691, 17.11489954122026447, 5.571627607371296764E-15 ) ) ;
#41557=CARTESIAN_POINT ( 'NONE',  ( 45.08926718327026606, 40.00000000000000000, 51.56349680124436219 ) ) ;
#41571=CARTESIAN_POINT ( 'NONE',  ( -53.60515337853228601, 31.00000000000000355, -47.01024902908782366 ) ) ;
#41580=CARTESIAN_POINT ( 'NONE',  ( -71.82650799747224823, 31.00000000000000711, -41.60779115368423220 ) ) ;
#41581=CARTESIAN_POINT ( 'NONE',  ( -79.74759331938361129, 40.00000000000000711, -21.47736420602193874 ) ) ;
#41597=CARTESIAN_POINT ( 'NONE',  ( 94.17930118497612568, 39.99999999999999289, -12.41473344271720691 ) ) ;
#41611=ORIENTED_EDGE ( 'NONE', *, *, #15485, .F. ) ;
#41613=CARTESIAN_POINT ( 'NONE',  ( 14.33709021557830887, 40.00000000000000000, 24.89380824183666618 ) ) ;
#41624=CARTESIAN_POINT ( 'NONE',  ( 9.621748599878955588, 31.00000000000000355, 35.89595399306684698 ) ) ;
#41631=CARTESIAN_POINT ( 'NONE',  ( -59.40286837853895463, 31.00000000000000711, 52.11376356991771530 ) ) ;
#41637=CARTESIAN_POINT ( 'NONE',  ( 48.78760054486801323, 31.00000000000000355, -28.06521077754944926 ) ) ;
#41638=CARTESIAN_POINT ( 'NONE',  ( -39.09256291070916944, 40.00000000000000000, 79.30589209199378331 ) ) ;
#41651=CARTESIAN_POINT ( 'NONE',  ( 28.01378275134445772, 40.00000000000000000, -56.83506808085938644 ) ) ;
#41658=VERTEX_POINT ( 'NONE', #440 ) ;
#41677=VECTOR ( 'NONE', #10392, 999.9999999999998863 ) ;
#41682=CARTESIAN_POINT ( 'NONE',  ( -49.88601606984090608, 31.00000000000000355, -6.565487524765669214 ) ) ;
#41691=CARTESIAN_POINT ( 'NONE',  ( -52.79687664379660816, 40.00000000000000000, -30.48099731442381710 ) ) ;
#41693=CARTESIAN_POINT ( 'NONE',  ( 67.09393615765254992, 39.99999999999999289, 4.495243625008655819 ) ) ;
#41701=CARTESIAN_POINT ( 'NONE',  ( -4.233603722440171246, 40.00000000000000000, -32.08218167604271542 ) ) ;
#41714=CARTESIAN_POINT ( 'NONE',  ( 20.39742982868580157, 31.00000000000000355, 76.57971376064386959 ) ) ;
#41725=CARTESIAN_POINT ( 'NONE',  ( -7.793954689941437586, 31.00000000000000355, 28.94896179907300748 ) ) ;
#41734=CARTESIAN_POINT ( 'NONE',  ( 76.36724925129128394, 31.00000000000000000, 58.57876755120444301 ) ) ;
#41738=CARTESIAN_POINT ( 'NONE',  ( 23.62253089228586944, 40.00000000000000000, -11.62353008834529255 ) ) ;
#41767=CARTESIAN_POINT ( 'NONE',  ( -38.36856355434107257, 31.00000000000000355, 33.53830235993100217 ) ) ;
#41772=UNCERTAINTY_MEASURE_WITH_UNIT (LENGTH_MEASURE( 1.000000000000000082E-05 ), #4708, 'distance_accuracy_value', 'NONE');
#41774=CARTESIAN_POINT ( 'NONE',  ( 60.45897909546184934, 39.99999999999999289, -46.24578392211154210 ) ) ;
#41776=VECTOR ( 'NONE', #42400, 1000.000000000000000 ) ;
#41785=CARTESIAN_POINT ( 'NONE',  ( 21.58803501788969115, 31.00000000000000355, 63.55567069162312777 ) ) ;
#41795=CARTESIAN_POINT ( 'NONE',  ( -79.00001692110807028, 31.00000000000000711, 21.04436337235335230 ) ) ;
#41796=CARTESIAN_POINT ( 'NONE',  ( 74.83201185296370284, 39.99999999999999289, -43.08100868844128684 ) ) ;
#41798=ORIENTED_EDGE ( 'NONE', *, *, #28981, .T. ) ;
#41823=CARTESIAN_POINT ( 'NONE',  ( 15.66220904948252546, 40.00000000000000000, -31.63873590539992975 ) ) ;
#41835=CARTESIAN_POINT ( 'NONE',  ( -25.53337963587170023, 31.00000000000000355, 29.12008199578403023 ) ) ;
#41836=ORIENTED_EDGE ( 'NONE', *, *, #42019, .T. ) ;
#41843=CARTESIAN_POINT ( 'NONE',  ( 5.399612364985509672, 31.00000000000000355, -82.60416666586320389 ) ) ;
#41845=CARTESIAN_POINT ( 'NONE',  ( -49.95450512538511134, 31.00000000000000355, 13.28959769214884545 ) ) ;
#41847=CARTESIAN_POINT ( 'NONE',  ( 22.58587702529213104, 40.00000000000000000, 84.29678642628191199 ) ) ;
#41860=CARTESIAN_POINT ( 'NONE',  ( -30.22953878324074495, 40.00000000000000000, 61.32923288305941867 ) ) ;
#41886=CARTESIAN_POINT ( 'NONE',  ( -104.8158553526607477, 17.11489954122027157, 3.963965400206364453 ) ) ;
#41887=CARTESIAN_POINT ( 'NONE',  ( -13.51098712749246467, 31.00000000000000355, -50.41620372279128048 ) ) ;
#41895=SHAPE_REPRESENTATION ( 'Return Coil Spring', ( #13552 ), #18474 ) ;
#41896=CARTESIAN_POINT ( 'NONE',  ( -38.74991464700507748, 40.00000000000000000, 44.18781823130588293 ) ) ;
#41905=CARTESIAN_POINT ( 'NONE',  ( -23.50435451693408950, 40.00000000000000000, 30.64856077952424940 ) ) ;
#41919=CARTESIAN_POINT ( 'NONE',  ( 37.87019299815447937, 31.00000000000000355, -76.55254356380190472 ) ) ;
#41928=CARTESIAN_POINT ( 'NONE',  ( 26.89767027507546615, 31.00000000000000355, -1.736414864505229527 ) ) ;
#41939=CARTESIAN_POINT ( 'NONE',  ( 81.71702119589899382, 31.00000000000000000, -47.19735719316410183 ) ) ;
#41942=CARTESIAN_POINT ( 'NONE',  ( 22.42277067908921850, 40.00000000000000000, 12.94072372014797701 ) ) ;
#41943=CARTESIAN_POINT ( 'NONE',  ( 9.106956811744730373, 40.00000000000000000, -33.78410985268681799 ) ) ;
#41966=CARTESIAN_POINT ( 'NONE',  ( -105.9879088449591933, 17.11489954122026447, -2.880719929157669945 ) ) ;
#41971=CARTESIAN_POINT ( 'NONE',  ( -51.89982240187124063, 31.00000000000000355, 3.308651922604603168 ) ) ;
#41977=CARTESIAN_POINT ( 'NONE',  ( -43.11175393642376719, 40.00000000000000000, 56.02072642018850246 ) ) ;
#41988=CARTESIAN_POINT ( 'NONE',  ( 40.54457361686378647, 31.00000000000000355, 52.83773991529862712 ) ) ;
#41997=CARTESIAN_POINT ( 'NONE',  ( -73.09555549758189841, 31.00000000000000711, 35.91380138263622257 ) ) ;
#41998=CARTESIAN_POINT ( 'NONE',  ( -79.17211738000736432, 40.00000000000000711, 45.58486055166100215 ) ) ;
#42014=ORIENTED_EDGE ( 'NONE', *, *, #33914, .T. ) ;
#42019=EDGE_CURVE ( 'NONE', #17691, #40502, #4358, .T. ) ;
#42026=CARTESIAN_POINT ( 'NONE',  ( -40.32452739091078797, 40.00000000000000000, -13.76986825753265720 ) ) ;
#42036=CARTESIAN_POINT ( 'NONE',  ( -12.24460912605626106, 31.00000000000000355, 36.08157028455360660 ) ) ;
#42043=CARTESIAN_POINT ( 'NONE',  ( 6.054110834496887250, 31.00000000000000355, -92.60416666599778068 ) ) ;
#42046=CARTESIAN_POINT ( 'NONE',  ( -35.18788409414197815, 31.00000000000000355, -40.25400722681192178 ) ) ;
#42047=CARTESIAN_POINT ( 'NONE',  ( 57.05379307147669721, 39.99999999999999289, -74.37948018729004218 ) ) ;
#42058=AXIS2_PLACEMENT_3D ( 'NONE', #30717, #9978, #39643 ) ;
#42060=CARTESIAN_POINT ( 'NONE',  ( -62.77658523491555798, 40.00000000000000711, 48.16944601536268777 ) ) ;
#42092=CARTESIAN_POINT ( 'NONE',  ( -12.41726970680908515, 31.00000000000000355, 46.38546114896210071 ) ) ;
#42098=CARTESIAN_POINT ( 'NONE',  ( 42.05404839982585941, 40.00000000000000000, -47.95475229022623864 ) ) ;
#42105=CARTESIAN_POINT ( 'NONE',  ( -26.76192867387533170, 40.00000000000000000, -15.44647709060871321 ) ) ;
#42120=CARTESIAN_POINT ( 'NONE',  ( -37.02054590706428172, 31.00000000000000355, -75.34311506435014394 ) ) ;
#42128=CARTESIAN_POINT ( 'NONE',  ( -13.16936484334534008, 40.00000000000000000, 99.04657264458933241 ) ) ;
#42129=CARTESIAN_POINT ( 'NONE',  ( 24.14050371820132668, 31.00000000000000355, 13.97356841391235704 ) ) ;
#42146=CARTESIAN_POINT ( 'NONE',  ( -21.73352778766994575, 40.00000000000000000, 19.07242603999910457 ) ) ;
#42147=CARTESIAN_POINT ( 'NONE',  ( 10.06970066534629815, 40.00000000000000000, 37.84957806120350199 ) ) ;
#42152=CARTESIAN_POINT ( 'NONE',  ( -16.80298683001097260, 31.00000000000000355, -2.367532924972505892 ) ) ;
#42174=CARTESIAN_POINT ( 'NONE',  ( 36.84045577241590763, 31.00000000000000355, -41.86038302678687018 ) ) ;
#42183=CARTESIAN_POINT ( 'NONE',  ( 66.15140951845482675, 39.99999999999999289, -38.07406969931857077 ) ) ;
#42194=CARTESIAN_POINT ( 'NONE',  ( 61.18335543008118549, 31.00000000000000000, -20.78249587198964576 ) ) ;
#42209=CARTESIAN_POINT ( 'NONE',  ( 83.51212062385671686, 31.00000000000000000, -48.08891344041042970 ) ) ;
#42211=CARTESIAN_POINT ( 'NONE',  ( 91.58570893733640617, 39.99999999999999289, -30.97307622143650718 ) ) ;
#42224=EDGE_CURVE ( 'NONE', #17691, #9181, #31185, .T. ) ;
#42228=CARTESIAN_POINT ( 'NONE',  ( -15.43003214871278139, 31.00000000000000355, -17.59684744742187945 ) ) ;
#42241=CARTESIAN_POINT ( 'NONE',  ( 44.12914893502614433, 40.00000000000000000, -14.89880614700436645 ) ) ;
#42251=ORIENTED_EDGE ( 'NONE', *, *, #38185, .T. ) ;
#42254=CARTESIAN_POINT ( 'NONE',  ( 8.528031178950213231, 31.00000000000000355, -31.86521141804621493 ) ) ;
#42260=CARTESIAN_POINT ( 'NONE',  ( 74.70319961851696178, 31.00000000000000000, -57.31929289364909152 ) ) ;
#42265=CARTESIAN_POINT ( 'NONE',  ( 21.04585062970478759, 31.00000000000000355, -61.66509230325024049 ) ) ;
#42267=CARTESIAN_POINT ( 'NONE',  ( -12.78314611188302052, 40.00000000000000000, 97.07982689498881257 ) ) ;
#42283=CARTESIAN_POINT ( 'NONE',  ( 74.72486387243833406, 39.99999999999999289, 9.837939412698395003 ) ) ;
#42311=CARTESIAN_POINT ( 'NONE',  ( 54.89583333452979730, 31.00000000000000355, -3.599741573803383332 ) ) ;
#42320=CARTESIAN_POINT ( 'NONE',  ( 64.78932475141161262, 39.99999999999999289, 8.528958657501300777 ) ) ;
#42322=DIRECTION ( 'NONE',  ( 0.000000000000000000, 1.000000000000000000, 0.000000000000000000 ) ) ;
#42324=MANIFOLD_SOLID_BREP ( 'Extrude-Thin1', #1724 ) ;
#42330=VERTEX_POINT ( 'NONE', #42676 ) ;
#42331=CARTESIAN_POINT ( 'NONE',  ( -38.45388554590046937, 40.00000000000000000, -13.05014827191142679 ) ) ;
#42345=CARTESIAN_POINT ( 'NONE',  ( 64.75392801420538547, 31.00000000000000000, -56.64582372546510669 ) ) ;
#42349=B_SPLINE_CURVE_WITH_KNOTS ( 'NONE', 3,
 ( #12803, #25909, #32646, #19583, #2295, #2933, #26115, #22873, #32427, #42228, #12390, #16087, #42872, #5804, #22437, #39170, #8653, #38961, #39380, #22647, #22234, #6022, #42653, #22010, #29387, #6237, #32853, #16294, #13029, #35266, #5392, #18757, #35685, #32013, #2095, #19159, #28754, #25490, #38750, #8880, #35478, #18962, #32216, #25711, #2511, #33293, #36536, #26969, #7302, #3375, #36765, #40247, #13671, #3150, #40460, #16744, #4022, #20667, #40018, #10592, #16523, #19794, #33934, #3790, #10150, #9935, #17397, #6444, #16954, #302, #26536, #33498, #39808, #30035, #30674, #23925, #29826, #39602, #749, #27190, #6660, #541, #10380, #7090, #14108, #85, #9731, #13891, #37192, #20235, #13456, #26749, #17175, #23080, #6880, #23501, #23718, #36327, #3581, #33061, #36980, #20443, #30237, #30459, #43092, #33706, #13242, #23284, #20024, #5116, #28060, #21550, #41550, #14543, #1842, #18061, #27846, #20894, #34576, #34145, #4242, #31322, #14973, #10816, #4686, #34359, #1405, #38064, #34798, #37411, #41103, #14759, #41320, #11469, #38277, #18478, #14312, #30883, #31102, #11695, #962, #17614, #7535, #17826, #24807, #37835, #27624, #28279, #1188, #31748, #4907, #11256, #8186, #40892, #25036, #24585, #1620, #35007, #7959, #4455, #8394, #21758, #27399, #21324, #18269, #31534, #40666, #24147, #11048, #24374, #37626, #7747, #21106, #16038, #42402, #15823, #35217, #35637, #25237, #32593, #15606, #22597, #35839, #32801, #12119, #41767, #38919, #22180, #18707, #5966, #18911, #22390, #41971, #25659, #15409, #35436, #5555, #42603, #2247, #2676, #19112, #12546, #5754, #19324, #15203, #2460, #12755, #29337, #9246, #36066, #29130, #26060, #39323, #28910, #28505, #32375, #42174, #8599, #25862, #21961, #5341, #39126, #9461, #11910, #22816, #32168, #6188, #19533, #38482, #31971, #12336, #2047, #28706, #25439, #38701, #8824, #9034, #6397, #6602, #30409, #19744, #9684, #26278, #36485, #6830, #13404, #33007, #3737, #19971, #23879, #23671, #33240, #26916, #3094, #484, #29983, #20395, #10541, #3321, #9887, #13843, #33655, #17120, #36, #16697, #10329, #26700, #7250, #30188, #249, #36277, #23028, #27144, #40407, #13620, #3533, #16465, #23447, #12973, #37142, #39967, #36928, #7040, #20608, #43041, #29545, #10097, #23237, #29768, #2882, #36712, #20189, #13194, #33447, #26485, #16909, #40192, #16246, #42814, #39549, #39757, #14917, #28221, #21495, #695, #11638, #38002, #37788, #1355, #1570, #27565, #41487, #8130, #34746, #14487, #24324, #37580, #41270, #24980, #31044, #34308, #21056, #20842, #38226, #8343, #4854, #14056, #33883, #18213, #7907, #14702, #3971, #40839, #17350, #31484, #30628, #27796, #7689, #4401, #11414, #27350, #17773, #21269, #40613, #1136, #10759, #34516, #4185, #24093, #41053, #11203, #37363, #7480, #24536, #4629, #18005, #31269, #34098, #17561, #30835, #907, #28009, #24751, #14261, #10994, #28446, #41714, #15766, #11858, #28853, #21908, #25605, #32117, #15355, #18651, #8984, #32538, #28646, #18857, #22334, #38863, #12700, #8550, #25183, #25385, #5911, #38431, #26005, #35161, #1785, #15985, #29075, #22125, #5280, #29282, #31688, #42120, #35582, #31915, #15558, #1995, #5500, #39066, #42549, #8765, #41919, #19264, #12067, #2626, #42345, #39266, #12492, #2198, #22544, #5065, #38644, #35384, #12277, #5702, #25809, #19058, #32320, #2400, #9192, #15145, #35780, #21698, #34954, #18423, #36877, #3035, #33177, #39915, #32956, #9833, #2828, #33395, #42754, #26648, #29932, #9630, #29707, #42983, #6985, #13141, #20342, #33605, #3687, #36430, #26860, #17065, #39702, #16406, #30350, #39494, #426, #16858, #13792, #30142, #3266, #10272, #36651, #6778, #12914, #16192, #23619, #27088, #20138, #10045, #29490, #19854, #19481, #40133, #23185, #9399, #22752, #36008, #26432, #16645, #23389, #6546, #26218, #197, #19910, #13354, #36222, #3481, #22978, #13566, #6134, #32745, #6342, #19690, #24695, #3910, #40355, #1517, #27961, #37311, #17298, #21004, #7855, #8075, #34047, #34693, #14654, #41216, #34255, #30782, #858, #4574, #18168, #37532, #40784 ),
 .UNSPECIFIED., .F., .F.,
 ( 4, 2, 2, 2, 2, 2, 2, 2, 2, 2, 2, 2, 2, 2, 2, 2, 2, 2, 2, 2, 2, 2, 2, 2, 2, 2, 2, 2, 2, 2, 2, 2, 2, 2, 2, 2, 2, 2, 2, 2, 2, 2, 2, 2, 2, 2, 2, 2, 2, 2, 2, 2, 2, 2, 2, 2, 2, 2, 2, 2, 2, 2, 2, 2, 2, 2, 2, 2, 2, 2, 2, 2, 2, 2, 2, 2, 2, 2, 2, 2, 2, 2, 2, 2, 2, 2, 2, 2, 2, 2, 2, 2, 2, 2, 2, 2, 2, 2, 2, 2, 2, 2, 2, 2, 2, 2, 2, 2, 2, 2, 2, 2, 2, 2, 2, 2, 2, 2, 2, 2, 2, 2, 2, 2, 2, 2, 2, 2, 2, 2, 2, 2, 2, 2, 2, 2, 2, 2, 2, 2, 2, 2, 2, 2, 2, 2, 2, 2, 2, 2, 2, 2, 2, 2, 2, 2, 2, 2, 2, 2, 2, 2, 2, 2, 2, 2, 2, 2, 2, 2, 2, 2, 2, 2, 2, 2, 2, 2, 2, 2, 2, 2, 2, 2, 2, 2, 2, 2, 2, 2, 2, 2, 2, 2, 2, 2, 2, 2, 2, 2, 2, 2, 2, 2, 2, 2, 2, 2, 2, 2, 2, 2, 2, 2, 2, 2, 2, 2, 2, 2, 2, 2, 2, 2, 2, 2, 2, 2, 2, 2, 2, 2, 2, 2, 2, 2, 2, 2, 2, 2, 2, 2, 2, 2, 2, 2, 2, 2, 2, 2, 2, 2, 2, 2, 2, 2, 4 ),
 ( 0.000000000000000000, 0.003906250000000000000, 0.007812500000000000000, 0.01171875000000000000, 0.01562500000000000000, 0.01953125000000000000, 0.02343750000000000000, 0.02734375000000000000, 0.03125000000000000000, 0.03515625000000000000, 0.03906250000000000000, 0.04296875000000000000, 0.04687500000000000000, 0.05078125000000000000, 0.05468750000000000000, 0.05859375000000000000, 0.06250000000000000000, 0.06640625000000000000, 0.07031250000000000000, 0.07421875000000000000, 0.07812500000000000000, 0.08203125000000000000, 0.08593750000000000000, 0.08984375000000000000, 0.09375000000000000000, 0.09765625000000000000, 0.1015625000000000000, 0.1054687500000000000, 0.1093750000000000000, 0.1132812500000000000, 0.1171875000000000000, 0.1210937500000000000, 0.1250000000000000000, 0.1289062500000000000, 0.1328125000000000000, 0.1367187500000000000, 0.1406250000000000000, 0.1445312500000000000, 0.1484375000000000000, 0.1523437500000000000, 0.1562500000000000000, 0.1601562500000000000, 0.1640625000000000000, 0.1679687500000000000, 0.1718750000000000000, 0.1757812500000000000, 0.1796875000000000000, 0.1835937500000000000, 0.1875000000000000000, 0.1914062500000000000, 0.1953125000000000000, 0.1992187500000000000, 0.2031250000000000000, 0.2070312500000000000, 0.2109375000000000000, 0.2148437500000000000, 0.2187500000000000000, 0.2226562500000000000, 0.2265625000000000000, 0.2304687500000000000, 0.2343750000000000000, 0.2382812500000000000, 0.2421875000000000000, 0.2460937500000000000, 0.2500000000000000000, 0.2539062500000000000, 0.2578125000000000000, 0.2617187500000000000, 0.2656250000000000000, 0.2695312500000000000, 0.2734375000000000000, 0.2773437500000000000, 0.2812500000000000000, 0.2851562500000000000, 0.2890625000000000000, 0.2929687500000000000, 0.2968750000000000000, 0.3007812500000000000, 0.3046875000000000000, 0.3085937500000000000, 0.3125000000000000000, 0.3164062500000000000, 0.3203125000000000000, 0.3242187500000000000, 0.3281250000000000000, 0.3320312500000000000, 0.3359375000000000000, 0.3398437500000000000, 0.3437500000000000000, 0.3476562500000000000, 0.3515625000000000000, 0.3554687500000000000, 0.3593750000000000000, 0.3632812500000000000, 0.3671875000000000000, 0.3710937500000000000, 0.3750000000000000000, 0.3789062500000000000, 0.3828125000000000000, 0.3867187500000000000, 0.3906250000000000000, 0.3945312500000000000, 0.3984375000000000000, 0.4023437500000000000, 0.4062500000000000000, 0.4101562500000000000, 0.4140625000000000000, 0.4179687500000000000, 0.4218750000000000000, 0.4257812500000000000, 0.4296875000000000000, 0.4335937500000000000, 0.4375000000000000000, 0.4414062500000000000, 0.4453125000000000000, 0.4492187500000000000, 0.4531250000000000000, 0.4570312500000000000, 0.4609375000000000000, 0.4648437500000000000, 0.4687500000000000000, 0.4726562500000000000, 0.4765625000000000000, 0.4804687500000000000, 0.4843750000000000000, 0.4882812500000000000, 0.4921875000000000000, 0.4960937500000000000, 0.5000000000000000000, 0.5039062500000000000, 0.5078125000000000000, 0.5117187500000000000, 0.5156250000000000000, 0.5195312500000000000, 0.5234375000000000000, 0.5273437500000000000, 0.5312500000000000000, 0.5351562500000000000, 0.5390625000000000000, 0.5429687500000000000, 0.5468750000000000000, 0.5507812500000000000, 0.5546875000000000000, 0.5585937500000000000, 0.5625000000000000000, 0.5664062500000000000, 0.5703125000000000000, 0.5742187500000000000, 0.5781250000000000000, 0.5820312500000000000, 0.5859375000000000000, 0.5898437500000000000, 0.5937500000000000000, 0.5976562500000000000, 0.6015625000000000000, 0.6054687500000000000, 0.6093750000000000000, 0.6132812500000000000, 0.6171875000000000000, 0.6210937500000000000, 0.6250000000000000000, 0.6289062500000000000, 0.6328125000000000000, 0.6367187500000000000, 0.6406250000000000000, 0.6445312500000000000, 0.6484375000000000000, 0.6523437500000000000, 0.6562500000000000000, 0.6601562500000000000, 0.6640625000000000000, 0.6679687500000000000, 0.6718750000000000000, 0.6757812500000000000, 0.6796875000000000000, 0.6835937500000000000, 0.6875000000000000000, 0.6914062500000000000, 0.6953125000000000000, 0.6992187500000000000, 0.7031250000000000000, 0.7070312500000000000, 0.7109375000000000000, 0.7148437500000000000, 0.7187500000000000000, 0.7226562500000000000, 0.7265625000000000000, 0.7304687500000000000, 0.7343750000000000000, 0.7382812500000000000, 0.7421875000000000000, 0.7460937500000000000, 0.7500000000000000000, 0.7539062500000000000, 0.7578125000000000000, 0.7617187500000000000, 0.7656250000000000000, 0.7695312500000000000, 0.7734375000000000000, 0.7773437500000000000, 0.7812500000000000000, 0.7851562500000000000, 0.7890625000000000000, 0.7929687500000000000, 0.7968750000000000000, 0.8007812500000000000, 0.8046875000000000000, 0.8085937500000000000, 0.8125000000000000000, 0.8164062500000000000, 0.8203125000000000000, 0.8242187500000000000, 0.8281250000000000000, 0.8320312500000000000, 0.8359375000000000000, 0.8398437500000000000, 0.8437500000000000000, 0.8476562500000000000, 0.8515625000000000000, 0.8554687500000000000, 0.8593750000000000000, 0.8632812500000000000, 0.8671875000000000000, 0.8710937500000000000, 0.8750000000000000000, 0.8789062500000000000, 0.8828125000000000000, 0.8867187500000000000, 0.8906250000000000000, 0.8945312500000000000, 0.8984375000000000000, 0.9023437500000000000, 0.9062500000000000000, 0.9101562500000000000, 0.9140625000000000000, 0.9179687500000000000, 0.9218750000000000000, 0.9257812500000000000, 0.9296875000000000000, 0.9335937500000000000, 0.9375000000000000000, 0.9414062500000000000, 0.9453125000000000000, 0.9492187500000000000, 0.9531250000000000000, 0.9570312500000000000, 0.9609375000000000000, 0.9648437500000000000, 0.9687500000000000000, 0.9726562500000000000, 0.9765625000000000000, 0.9804687500000000000, 0.9843750000000000000, 0.9882812500000000000, 0.9921875000000000000, 0.9960937500000000000, 1.000000000000000000 ),
 .UNSPECIFIED. ) ;
#42352=CARTESIAN_POINT ( 'NONE',  ( 25.57473013256711880, 40.00000000000000000, 95.94174708832935039 ) ) ;
#42361=ORIENTED_EDGE ( 'NONE', *, *, #26266, .F. ) ;
#42364=AXIS2_PLACEMENT_3D ( 'NONE', #10113, #40209, #29782 ) ;
#42365=CARTESIAN_POINT ( 'NONE',  ( 3.579113344806025054, 31.00000000000000355, 27.11441211503905535 ) ) ;
#42374=CARTESIAN_POINT ( 'NONE',  ( 24.89583333603155069, 40.00000000000000000, -1.636246165087041016 ) ) ;
#42375=CARTESIAN_POINT ( 'NONE',  ( -26.24023198663969580, 40.00000000000000000, -20.19409642360271917 ) ) ;
#42395=CARTESIAN_POINT ( 'NONE',  ( -87.52616871875942195, 40.00000000000000711, -23.43677886868077209 ) ) ;
#42400=DIRECTION ( 'NONE',  ( 0.000000000000000000, 1.000000000000000000, 0.000000000000000000 ) ) ;
#42402=CARTESIAN_POINT ( 'NONE',  ( 12.64472494877221997, 31.00000000000000355, 47.53373494968589341 ) ) ;
#42404=CARTESIAN_POINT ( 'NONE',  ( -105.9879088449591933, 40.00000000000000000, 2.119280070842335384 ) ) ;
#42408=CARTESIAN_POINT ( 'NONE',  ( 51.69257347811147696, 40.00000000000000000, 59.10123636508003386 ) ) ;
#42412=VERTEX_POINT ( 'NONE', #8903 ) ;
#42417=CARTESIAN_POINT ( 'NONE',  ( -5.399612364985466151, 31.00000000000000355, -82.39583333413678190 ) ) ;
#42429=CARTESIAN_POINT ( 'NONE',  ( -59.98614492175870794, 31.00000000000000711, 68.21249229744711329 ) ) ;
#42430=CARTESIAN_POINT ( 'NONE',  ( -87.75478321342750121, 40.00000000000000711, -29.92102470460831753 ) ) ;
#42459=CARTESIAN_POINT ( 'NONE',  ( 45.87644943786595064, 40.00000000000000000, 12.37342411884007731 ) ) ;
#42469=CARTESIAN_POINT ( 'NONE',  ( 31.10108666877329853, 31.00000000000000355, 17.95223046116557697 ) ) ;
#42474=CARTESIAN_POINT ( 'NONE',  ( -86.71682804797315214, 31.00000000000000711, 23.23408344657299196 ) ) ;
#42475=VECTOR ( 'NONE', #5536, 1000.000000000000114 ) ;
#42480=CARTESIAN_POINT ( 'NONE',  ( 16.92944795086299337, 31.00000000000000355, -62.81076020704204410 ) ) ;
#42481=CARTESIAN_POINT ( 'NONE',  ( -59.29355402628473826, 40.00000000000000000, -20.23837177251483155 ) ) ;
#42482=CARTESIAN_POINT ( 'NONE',  ( 58.84426737335365232, 40.00000000000000000, 76.69096868241209108 ) ) ;
#42493=CARTESIAN_POINT ( 'NONE',  ( -63.57631528421845957, 40.00000000000000711, -31.33741679916209222 ) ) ;
#42494=DIRECTION ( 'NONE',  ( 7.709882115452478166E-16, -1.000000000000000000, -0.000000000000000000 ) ) ;
#42514=ORIENTED_EDGE ( 'NONE', *, *, #15662, .F. ) ;
#42521=CARTESIAN_POINT ( 'NONE',  ( 55.10416666547021691, 31.00000000000000355, 3.599741573803287853 ) ) ;
#42524=CARTESIAN_POINT ( 'NONE',  ( 37.09854380387523776, 31.00000000000000355, 2.490183985263670685 ) ) ;
#42525=CARTESIAN_POINT ( 'NONE',  ( 43.85342918759069164, 40.00000000000000000, 49.98553323097543455 ) ) ;
#42535=ORIENTED_EDGE ( 'NONE', *, *, #40675, .F. ) ;
#42536=CARTESIAN_POINT ( 'NONE',  ( -24.21661388771557100, 40.00000000000000000, 41.94898165618241137 ) ) ;
#42546=VERTEX_POINT ( 'NONE', #16548 ) ;
#42549=CARTESIAN_POINT ( 'NONE',  ( 22.12670472278668399, 31.00000000000000355, -82.16725659058067777 ) ) ;
#42559=FACE_OUTER_BOUND ( 'NONE', #34511, .T. ) ;
#42570=CARTESIAN_POINT ( 'NONE',  ( -27.62299686580952240, 31.00000000000000355, -13.61136854378590577 ) ) ;
#42576=CARTESIAN_POINT ( 'NONE',  ( -27.33276042269523387, 40.00000000000000000, -31.15086293565511966 ) ) ;
#42577=CARTESIAN_POINT ( 'NONE',  ( 25.29542371717657545, 40.00000000000000000, 28.93716311999360613 ) ) ;
#42594=AXIS2_PLACEMENT_3D ( 'NONE', #10035, #6767, #22534 ) ;
#42603=CARTESIAN_POINT ( 'NONE',  ( -47.35250803175854628, 31.00000000000000355, -23.44639516808300073 ) ) ;
#42613=CARTESIAN_POINT ( 'NONE',  ( 46.16409756962309530, 40.00000000000000000, -59.99419878592187416 ) ) ;
#42626=CARTESIAN_POINT ( 'NONE',  ( 50.46169669344906339, 31.00000000000000355, 57.51940134901310131 ) ) ;
#42633=CARTESIAN_POINT ( 'NONE',  ( 58.37089435908782065, 31.00000000000000000, -75.89027429297952665 ) ) ;
#42634=CARTESIAN_POINT ( 'NONE',  ( -50.38378093996033869, 40.00000000000000711, 87.00968337440519917 ) ) ;
#42653=CARTESIAN_POINT ( 'NONE',  ( 12.70938237924789327, 31.00000000000000355, -21.97768283340561979 ) ) ;
#42656=B_SPLINE_CURVE_WITH_KNOTS ( 'NONE', 3,
 ( #26404, #13318, #386, #35597, #39672, #40094, #36843, #19071, #9797, #23789, #6951, #36397, #7162, #19870, #20518, #28867, #22344, #32332, #33141, #40969, #4095, #30952, #21403, #11545, #34217, #10896, #31394, #34009, #28128, #11325, #14828, #24656, #41177, #27468, #14391, #20962, #17468, #1036, #7385, #37913, #14174, #37493, #7602, #30540, #13964, #34650, #4311, #24888, #21619, #1478, #40744, #27700, #34426, #24228, #17683, #40528, #27923, #37269, #21176, #24443, #7817, #31182, #11116, #41394, #37698, #38138, #8262, #10663, #3871, #17253, #4772, #820, #24004, #4532, #17906, #14616, #18130, #608, #20742, #1271, #8034, #27258, #30746, #42254, #12615, #32034, #35292, #38771, #9313, #22035, #9107, #8901, #5188, #25930, #8675, #12192, #15900, #5826, #2118, #25516, #5412, #35501, #42469, #15049, #38350, #2539, #25305, #15281, #25731, #22255, #41624, #28569, #2317, #35075, #32449, #28358, #42036, #28776, #5620, #8467, #41835, #18982, #21828, #32236, #18554, #31826, #19184, #15478, #15680, #28987, #38982, #31599, #22459, #29201, #18781, #12408, #35702, #39189, #34868, #1912, #4983, #18338, #11988, #1694, #38553, #11778, #25102, #33520, #13053, #26559, #40267, #16767, #30054, #109, #22667, #19604, #6048, #3171, #29619, #26134, #13476, #12824, #39830, #43116, #9954, #26356, #36141, #23303, #10171, #19400, #19816, #9545, #3604, #16975, #23525, #32667, #325, #26766, #36556, #33310, #30258, #13692, #40037, #6685, #23103, #33083, #16316, #36787, #26994, #16547, #36348, #20046, #35919, #9750, #6897, #3395, #6257, #2744, #39623, #13262, #16109, #20252, #29408, #42675, #39404, #22895, #32873, #2951, #42894, #6462, #29846, #33955, #1212, #14333, #17197, #30482, #4474, #558, #17634, #10612, #27646, #30897, #13913, #31125, #981, #34594, #3812, #24170, #771, #7322, #37434, #14561, #27207, #20687, #24394, #7764, #40477, #24604, #34160, #34375, #4263, #37857, #23947, #4712, #17845, #21342, #27867, #41122, #4039, #20912, #27415, #37213, #7552, #17415, #11273, #30695, #33727, #14126, #18078, #40687, #40915, #10837, #31343, #28078, #7979, #11065, #37643, #21127, #1425, #14778, #10401, #23734, #37001, #7113, #20465, #2065, #31767, #11722, #28727, #28930, #24825, #25679, #4927, #41339, #2480, #42194, #38299, #18287, #21979, #35233, #8844, #12358, #5773, #31551, #15226, #15427, #1863, #9056, #41988, #1640, #5360, #41785, #12138, #15843, #28521, #15624, #25459, #25054, #19130, #11932, #18729, #22407, #38934, #38503, #31984, #25253, #38718, #11492, #22202, #8620, #38083, #35454, #21779, #32187, #5571, #14994, #28301, #18929, #41571, #2267, #8413, #35655, #32396, #5136, #35028, #8210, #21570, #34818, #18496, #16713, #20206, #42835, #33260, #5988, #39346, #43061, #26505, #19344, #9483, #30004, #29565, #26081, #36732, #32819, #39778, #56, #13425, #33030, #16056, #23048, #29358, #42626, #10118, #36506, #39986, #6627, #23254, #22839, #39571, #2903, #12775, #26301, #32614, #19988, #36088, #9264, #22617, #23469, #19552, #3116, #3552, #6851, #29151, #26716, #6205, #9701, #16487, #16268, #12994, #35862, #9905, #2694, #29792, #6415, #13210, #36298, #19766, #3345, #33467, #12565, #42417, #25883, #39142, #21290, #4422, #13867, #23688, #40634, #10782, #27589, #31068, #24557, #36949, #33902, #34117, #20633, #27817, #20863, #7060, #24115, #1155, #4210, #34541, #3992, #34326, #17579, #30427, #37808, #17368, #37383, #41073, #14509, #14076, #7500, #30648, #30852, #16926, #927, #27369, #30209, #14280, #40428, #7713, #40860, #20415, #33677, #11015, #3760, #24344, #17142, #37596, #21077, #23898, #27162, #7927, #716, #17793, #511, #11224, #270, #13642, #26936, #10563, #37162, #40217, #10351, #7272, #31503, #15375, #38247, #4877, #8789, #41513, #8570, #28671, #41939, #28470, #8152, #18443, #21519, #38028, #5083, #21929, #31712, #18675, #28245, #34768, #41734, #12088, #18030, #21726, #18239, #38665, #22148, #25407, #14726, #35406, #31936, #11879, #35181, #5521, #18878, #41291, #11659, #25207, #25002, #4652, #38451, #24772, #1809, #31293, #8363, #34976, #11438 ),
 .UNSPECIFIED., .F., .F.,
 ( 4, 2, 2, 2, 2, 2, 2, 2, 2, 2, 2, 2, 2, 2, 2, 2, 2, 2, 2, 2, 2, 2, 2, 2, 2, 2, 2, 2, 2, 2, 2, 2, 2, 2, 2, 2, 2, 2, 2, 2, 2, 2, 2, 2, 2, 2, 2, 2, 2, 2, 2, 2, 2, 2, 2, 2, 2, 2, 2, 2, 2, 2, 2, 2, 2, 2, 2, 2, 2, 2, 2, 2, 2, 2, 2, 2, 2, 2, 2, 2, 2, 2, 2, 2, 2, 2, 2, 2, 2, 2, 2, 2, 2, 2, 2, 2, 2, 2, 2, 2, 2, 2, 2, 2, 2, 2, 2, 2, 2, 2, 2, 2, 2, 2, 2, 2, 2, 2, 2, 2, 2, 2, 2, 2, 2, 2, 2, 2, 2, 2, 2, 2, 2, 2, 2, 2, 2, 2, 2, 2, 2, 2, 2, 2, 2, 2, 2, 2, 2, 2, 2, 2, 2, 2, 2, 2, 2, 2, 2, 2, 2, 2, 2, 2, 2, 2, 2, 2, 2, 2, 2, 2, 2, 2, 2, 2, 2, 2, 2, 2, 2, 2, 2, 2, 2, 2, 2, 2, 2, 2, 2, 2, 2, 2, 2, 2, 2, 2, 2, 2, 2, 2, 2, 2, 2, 2, 2, 2, 2, 2, 2, 2, 2, 2, 2, 2, 2, 2, 2, 2, 2, 2, 2, 2, 2, 2, 2, 2, 2, 2, 2, 2, 2, 2, 2, 2, 2, 2, 2, 2, 2, 2, 2, 2, 2, 2, 2, 2, 2, 2, 2, 2, 2, 2, 2, 2, 4 ),
 ( 0.000000000000000000, 0.003906250000000000000, 0.007812500000000000000, 0.01171875000000000000, 0.01562500000000000000, 0.01953125000000000000, 0.02343750000000000000, 0.02734375000000000000, 0.03125000000000000000, 0.03515625000000000000, 0.03906250000000000000, 0.04296875000000000000, 0.04687500000000000000, 0.05078125000000000000, 0.05468750000000000000, 0.05859375000000000000, 0.06250000000000000000, 0.06640625000000000000, 0.07031250000000000000, 0.07421875000000000000, 0.07812500000000000000, 0.08203125000000000000, 0.08593750000000000000, 0.08984375000000000000, 0.09375000000000000000, 0.09765625000000000000, 0.1015625000000000000, 0.1054687500000000000, 0.1093750000000000000, 0.1132812500000000000, 0.1171875000000000000, 0.1210937500000000000, 0.1250000000000000000, 0.1289062500000000000, 0.1328125000000000000, 0.1367187500000000000, 0.1406250000000000000, 0.1445312500000000000, 0.1484375000000000000, 0.1523437500000000000, 0.1562500000000000000, 0.1601562500000000000, 0.1640625000000000000, 0.1679687500000000000, 0.1718750000000000000, 0.1757812500000000000, 0.1796875000000000000, 0.1835937500000000000, 0.1875000000000000000, 0.1914062500000000000, 0.1953125000000000000, 0.1992187500000000000, 0.2031250000000000000, 0.2070312500000000000, 0.2109375000000000000, 0.2148437500000000000, 0.2187500000000000000, 0.2226562500000000000, 0.2265625000000000000, 0.2304687500000000000, 0.2343750000000000000, 0.2382812500000000000, 0.2421875000000000000, 0.2460937500000000000, 0.2500000000000000000, 0.2539062500000000000, 0.2578125000000000000, 0.2617187500000000000, 0.2656250000000000000, 0.2695312500000000000, 0.2734375000000000000, 0.2773437500000000000, 0.2812500000000000000, 0.2851562500000000000, 0.2890625000000000000, 0.2929687500000000000, 0.2968750000000000000, 0.3007812500000000000, 0.3046875000000000000, 0.3085937500000000000, 0.3125000000000000000, 0.3164062500000000000, 0.3203125000000000000, 0.3242187500000000000, 0.3281250000000000000, 0.3320312500000000000, 0.3359375000000000000, 0.3398437500000000000, 0.3437500000000000000, 0.3476562500000000000, 0.3515625000000000000, 0.3554687500000000000, 0.3593750000000000000, 0.3632812500000000000, 0.3671875000000000000, 0.3710937500000000000, 0.3750000000000000000, 0.3789062500000000000, 0.3828125000000000000, 0.3867187500000000000, 0.3906250000000000000, 0.3945312500000000000, 0.3984375000000000000, 0.4023437500000000000, 0.4062500000000000000, 0.4101562500000000000, 0.4140625000000000000, 0.4179687500000000000, 0.4218750000000000000, 0.4257812500000000000, 0.4296875000000000000, 0.4335937500000000000, 0.4375000000000000000, 0.4414062500000000000, 0.4453125000000000000, 0.4492187500000000000, 0.4531250000000000000, 0.4570312500000000000, 0.4609375000000000000, 0.4648437500000000000, 0.4687500000000000000, 0.4726562500000000000, 0.4765625000000000000, 0.4804687500000000000, 0.4843750000000000000, 0.4882812500000000000, 0.4921875000000000000, 0.4960937500000000000, 0.5000000000000000000, 0.5039062500000000000, 0.5078125000000000000, 0.5117187500000000000, 0.5156250000000000000, 0.5195312500000000000, 0.5234375000000000000, 0.5273437500000000000, 0.5312500000000000000, 0.5351562500000000000, 0.5390625000000000000, 0.5429687500000000000, 0.5468750000000000000, 0.5507812500000000000, 0.5546875000000000000, 0.5585937500000000000, 0.5625000000000000000, 0.5664062500000000000, 0.5703125000000000000, 0.5742187500000000000, 0.5781250000000000000, 0.5820312500000000000, 0.5859375000000000000, 0.5898437500000000000, 0.5937500000000000000, 0.5976562500000000000, 0.6015625000000000000, 0.6054687500000000000, 0.6093750000000000000, 0.6132812500000000000, 0.6171875000000000000, 0.6210937500000000000, 0.6250000000000000000, 0.6289062500000000000, 0.6328125000000000000, 0.6367187500000000000, 0.6406250000000000000, 0.6445312500000000000, 0.6484375000000000000, 0.6523437500000000000, 0.6562500000000000000, 0.6601562500000000000, 0.6640625000000000000, 0.6679687500000000000, 0.6718750000000000000, 0.6757812500000000000, 0.6796875000000000000, 0.6835937500000000000, 0.6875000000000000000, 0.6914062500000000000, 0.6953125000000000000, 0.6992187500000000000, 0.7031250000000000000, 0.7070312500000000000, 0.7109375000000000000, 0.7148437500000000000, 0.7187500000000000000, 0.7226562500000000000, 0.7265625000000000000, 0.7304687500000000000, 0.7343750000000000000, 0.7382812500000000000, 0.7421875000000000000, 0.7460937500000000000, 0.7500000000000000000, 0.7539062500000000000, 0.7578125000000000000, 0.7617187500000000000, 0.7656250000000000000, 0.7695312500000000000, 0.7734375000000000000, 0.7773437500000000000, 0.7812500000000000000, 0.7851562500000000000, 0.7890625000000000000, 0.7929687500000000000, 0.7968750000000000000, 0.8007812500000000000, 0.8046875000000000000, 0.8085937500000000000, 0.8125000000000000000, 0.8164062500000000000, 0.8203125000000000000, 0.8242187500000000000, 0.8281250000000000000, 0.8320312500000000000, 0.8359375000000000000, 0.8398437500000000000, 0.8437500000000000000, 0.8476562500000000000, 0.8515625000000000000, 0.8554687500000000000, 0.8593750000000000000, 0.8632812500000000000, 0.8671875000000000000, 0.8710937500000000000, 0.8750000000000000000, 0.8789062500000000000, 0.8828125000000000000, 0.8867187500000000000, 0.8906250000000000000, 0.8945312500000000000, 0.8984375000000000000, 0.9023437500000000000, 0.9062500000000000000, 0.9101562500000000000, 0.9140625000000000000, 0.9179687500000000000, 0.9218750000000000000, 0.9257812500000000000, 0.9296875000000000000, 0.9335937500000000000, 0.9375000000000000000, 0.9414062500000000000, 0.9453125000000000000, 0.9492187500000000000, 0.9531250000000000000, 0.9570312500000000000, 0.9609375000000000000, 0.9648437500000000000, 0.9687500000000000000, 0.9726562500000000000, 0.9765625000000000000, 0.9804687500000000000, 0.9843750000000000000, 0.9882812500000000000, 0.9921875000000000000, 0.9960937500000000000, 1.000000000000000000 ),
 .UNSPECIFIED. ) ;
#42664=CARTESIAN_POINT ( 'NONE',  ( -10.41556553088919834, 40.00000000000000000, 38.62046602037417387 ) ) ;
#42675=CARTESIAN_POINT ( 'NONE',  ( -25.89845354150052259, 31.00000000000000355, -44.83417823681238445 ) ) ;
#42676=CARTESIAN_POINT ( 'NONE',  ( -16.80298683001097260, 40.00000000000000000, 2.367532924972517439 ) ) ;
#42680=CARTESIAN_POINT ( 'NONE',  ( -66.93673649651354651, 31.00000000000000711, 58.72203107584222437 ) ) ;
#42683=CARTESIAN_POINT ( 'NONE',  ( -56.33579487689731735, 31.00000000000000355, -27.88694065509425002 ) ) ;
#42685=CARTESIAN_POINT ( 'NONE',  ( -71.90006454724937157, 40.00000000000000711, 4.599370544632132685 ) ) ;
#42686=CARTESIAN_POINT ( 'NONE',  ( -31.57754862722326905, 40.00000000000000000, 93.01713655900283584 ) ) ;
#42688=ADVANCED_FACE ( 'NONE', ( #4713 ), #41124, .F. ) ;
#42697=CARTESIAN_POINT ( 'NONE',  ( 75.10416666583130052, 39.99999999999999289, 4.908738512847474311 ) ) ;
#42700=DIRECTION ( 'NONE',  ( 0.000000000000000000, 0.000000000000000000, 1.000000000000000000 ) ) ;
#42726=CARTESIAN_POINT ( 'NONE',  ( -37.49462465745612860, 31.00000000000000355, -48.86220178749748300 ) ) ;
#42729=CARTESIAN_POINT ( 'NONE',  ( 30.20675218207096790, 31.00000000000000355, 23.25504409023748309 ) ) ;
#42730=CARTESIAN_POINT ( 'NONE',  ( 64.36038921521112854, 39.99999999999999289, -37.17434371002195803 ) ) ;
#42740=CARTESIAN_POINT ( 'NONE',  ( 30.63689417572177831, 40.00000000000000000, 34.91779699477408627 ) ) ;
#42754=CARTESIAN_POINT ( 'NONE',  ( -40.08783408682389648, 31.00000000000000355, 81.04563091337925584 ) ) ;
#42773=CARTESIAN_POINT ( 'NONE',  ( -30.10416666442597844, 31.00000000000000355, -1.963495399902747574 ) ) ;
#42780=CARTESIAN_POINT ( 'NONE',  ( 34.94781834021004840, 40.00000000000000000, -26.81980329959834108 ) ) ;
#42782=CARTESIAN_POINT ( 'NONE',  ( 19.31996883371318674, 40.00000000000000000, 33.58758284028577634 ) ) ;
#42814=CARTESIAN_POINT ( 'NONE',  ( 41.67488199336423804, 31.00000000000000355, 54.49293397273885375 ) ) ;
#42823=CARTESIAN_POINT ( 'NONE',  ( 37.87019299813560025, 40.00000000000000000, -76.55254356380190472 ) ) ;
#42835=CARTESIAN_POINT ( 'NONE',  ( 32.44529481510334534, 31.00000000000000355, -65.82339768528792945 ) ) ;
#42846=CARTESIAN_POINT ( 'NONE',  ( -87.75478321338633236, 31.00000000000000711, -29.92102470462889130 ) ) ;
#42847=CARTESIAN_POINT ( 'NONE',  ( 24.72345498302142630, 40.00000000000000000, -91.84610802670698604 ) ) ;
#42858=CARTESIAN_POINT ( 'NONE',  ( -101.6738636939643357, 39.99999999999999289, -5.192942712545352890 ) ) ;
#42871=EDGE_LOOP ( 'NONE', ( #31791, #34412, #9869, #25645, #38929, #2046, #42251, #13167, #34597, #40656, #6771, #11981, #346, #26987, #15829, #40078, #21362, #7717, #33950, #24088, #17873, #41332, #27439, #5574, #38737, #41798 ) ) ;
#42872=CARTESIAN_POINT ( 'NONE',  ( -10.52919346384764054, 31.00000000000000355, -21.36894910329525032 ) ) ;
#42879=CARTESIAN_POINT ( 'NONE',  ( -20.27214883179920690, 40.00000000000000000, 34.96734655410256210 ) ) ;
#42881=CIRCLE ( 'NONE', #24124, 2.000000000000000888 ) ;
#42894=CARTESIAN_POINT ( 'NONE',  ( -3.436116956419240864, 31.00000000000000355, -52.39583333462812931 ) ) ;
#42901=CARTESIAN_POINT ( 'NONE',  ( -89.62817255407412631, 31.00000000000000711, -11.80141054548196422 ) ) ;
#42904=CARTESIAN_POINT ( 'NONE',  ( -22.66037885604483648, 31.00000000000000355, 66.40833514169634100 ) ) ;
#42905=CARTESIAN_POINT ( 'NONE',  ( 8.965261019434027645, 40.00000000000000000, 68.85524230650666766 ) ) ;
#42924=CARTESIAN_POINT ( 'NONE',  ( -51.96644965832453522, 40.00000000000000711, 59.25555446698126616 ) ) ;
#42952=CARTESIAN_POINT ( 'NONE',  ( -46.07128526072433772, 31.00000000000000355, -40.40198152342698990 ) ) ;
#42955=CARTESIAN_POINT ( 'NONE',  ( -29.39530816626169241, 31.00000000000000355, -14.54745122861254814 ) ) ;
#42957=CARTESIAN_POINT ( 'NONE',  ( 40.54457361686378647, 40.00000000000000000, 52.83773991529862712 ) ) ;
#42965=ORIENTED_EDGE ( 'NONE', *, *, #9832, .F. ) ;
#42966=CARTESIAN_POINT ( 'NONE',  ( -5.542584477697039880, 40.00000000000000000, -42.01772079774592328 ) ) ;
#42983=CARTESIAN_POINT ( 'NONE',  ( -72.38966680861454961, 31.00000000000000711, 55.38960906678870089 ) ) ;
#43000=CARTESIAN_POINT ( 'NONE',  ( 20.45440555730427690, 31.00000000000000355, -26.67302265141799467 ) ) ;
#43007=CARTESIAN_POINT ( 'NONE',  ( 11.12085686420672381, 40.00000000000000000, -41.54537790535560760 ) ) ;
#43010=CARTESIAN_POINT ( 'NONE',  ( -38.36856355434107968, 40.00000000000000000, 33.53830235993100217 ) ) ;
#43026=LINE ( 'NONE', #39740, #13217 ) ;
#43041=CARTESIAN_POINT ( 'NONE',  ( 59.60939625460783731, 31.00000000000000000, -29.27517545780145269 ) ) ;
#43050=CARTESIAN_POINT ( 'NONE',  ( 10.26812810425290579, 40.00000000000000000, 78.79123036454033979 ) ) ;
#43061=CARTESIAN_POINT ( 'NONE',  ( 55.63593431947571588, 31.00000000000000000, -48.80962981700470493 ) ) ;
#43072=CARTESIAN_POINT ( 'NONE',  ( -70.09526419939506070, 31.00000000000000711, -61.63891210113990837 ) ) ;
#43090=FACE_OUTER_BOUND ( 'NONE', #5836, .T. ) ;
#43092=CARTESIAN_POINT ( 'NONE',  ( 28.69597684714336339, 31.00000000000000355, 25.25520295781697655 ) ) ;
#43100=CARTESIAN_POINT ( 'NONE',  ( -35.18788409414197815, 40.00000000000000000, -40.25400722681193599 ) ) ;
#43116=CARTESIAN_POINT ( 'NONE',  ( 43.96541952717798551, 31.00000000000000355, 11.76906328551413239 ) ) ;
#43121=CARTESIAN_POINT ( 'NONE',  ( -12.78314611188302052, 31.00000000000000355, 97.07982689498881257 ) ) ;
#43125=CARTESIAN_POINT ( 'NONE',  ( 43.45541166190962912, 31.00000000000000355, -49.38773770141698805 ) ) ;
#43126=CARTESIAN_POINT ( 'NONE',  ( 21.04585062969761822, 40.00000000000000000, -61.66509230325024760 ) ) ;
#43127=CARTESIAN_POINT ( 'NONE',  ( 76.36724925129128394, 39.99999999999999289, 58.57876755120444301 ) ) ;
#43142=CARTESIAN_POINT ( 'NONE',  ( -39.09256291070916944, 40.00000000000000000, 79.30589209199378331 ) ) ;
#43170=CARTESIAN_POINT ( 'NONE',  ( -3.763366191185464782, 31.00000000000000355, 57.60416666550938203 ) ) ;
#43173=CARTESIAN_POINT ( 'NONE',  ( 36.95980244579787666, 31.00000000000000355, 4.931273285801173856 ) ) ;
#43174=CARTESIAN_POINT ( 'NONE',  ( 17.40022565512299479, 40.00000000000000000, 64.93645345284011228 ) ) ;
#43181=CARTESIAN_POINT ( 'NONE',  ( -27.33276042269523387, 40.00000000000000000, -31.15086293565511966 ) ) ;
ENDSEC;
END-ISO-10303-21;
